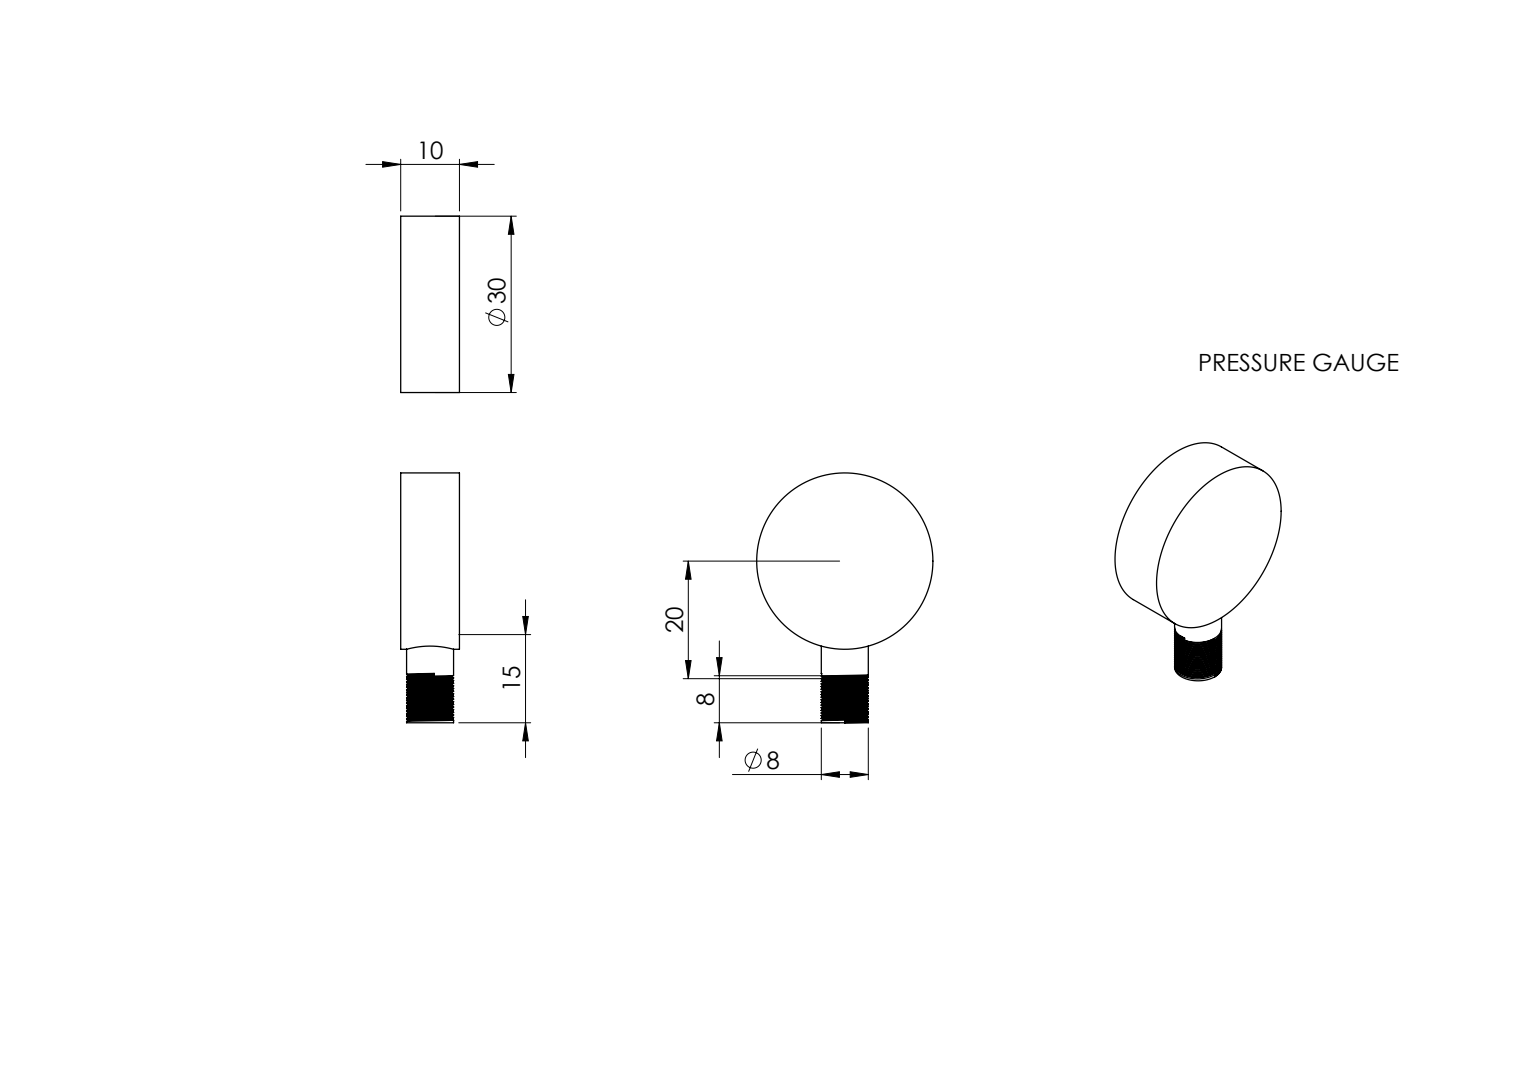
ISO-10303-21;
HEADER;
FILE_DESCRIPTION (('STEP AP214'),
    '1' );
FILE_NAME ('pressure gauge.step',
    '2026-10-26T05:42:23',
    ( '' ),
    ( '' ),
    'SwSTEP 2.0',
    'SolidWorks 2026',
    '' );
FILE_SCHEMA (( 'AUTOMOTIVE_DESIGN' ));
ENDSEC;

DATA;
#24=CARTESIAN_POINT ( 'NONE',  ( -7.967954043666661671E-16, 16.24062499938548143, 34.33755215474603517 ) ) ;
#66=CARTESIAN_POINT ( 'NONE',  ( -3.756430356250000102, 17.92812499938548498, 30.00000000000000000 ) ) ;
#88=CARTESIAN_POINT ( 'NONE',  ( -3.999999999999999112, 19.88749999999999929, 27.69059892324149530 ) ) ;
#102=CARTESIAN_POINT ( 'NONE',  ( -1.071796769724496334, 15.72634618820330310, 26.00000000000000355 ) ) ;
#120=CARTESIAN_POINT ( 'NONE',  ( 3.756430356250000546, 13.57812499938548711, 27.83122392262697886 ) ) ;
#135=CARTESIAN_POINT ( 'NONE',  ( 1.878215178125000495, 19.01562499938548356, 26.74683588394047007 ) ) ;
#150=CARTESIAN_POINT ( 'NONE',  ( 2.828200636599751609E-16, 18.40624999877096712, 25.38119784648299415 ) ) ;
#153=CARTESIAN_POINT ( 'NONE',  ( -3.999999999999999112, 17.58124999877096428, 27.69059892324149530 ) ) ;
#183=CARTESIAN_POINT ( 'NONE',  ( -1.071796769724492115, 14.61740381056766402, 34.00000000000000000 ) ) ;
#197=ORIENTED_EDGE ( 'NONE', *, *, #67048, .T. ) ;
#202=ORIENTED_EDGE ( 'NONE', *, *, #63479, .F. ) ;
#210=ORIENTED_EDGE ( 'NONE', *, *, #33045, .F. ) ;
#259=DIRECTION ( 'NONE',  ( -0.000000000000000000, -1.000000000000000000, -0.000000000000000000 ) ) ;
#264=CARTESIAN_POINT ( 'NONE',  ( -7.967954043666661671E-16, 14.44062499938548250, 34.33755215474603517 ) ) ;
#265=CARTESIAN_POINT ( 'NONE',  ( -1.999999999999999112, 13.94374999877096677, 26.53589838486224650 ) ) ;
#274=EDGE_LOOP ( 'NONE', ( #54307, #37100, #57406 ) ) ;
#276=( BOUNDED_CURVE ( )  B_SPLINE_CURVE ( 2, ( #33865, #44247, #5440, #72677, #27980, #66778, #16868, #50510, #73036 ),
 .UNSPECIFIED., .F., .F. ) 
 B_SPLINE_CURVE_WITH_KNOTS ( ( 3, 2, 2, 2, 3 ),
 ( 0.2916666666666666852, 0.2962962962962962798, 0.3055555555555555802, 0.3148148148148148251, 0.3194444444444444753 ),
 .UNSPECIFIED. ) 
 CURVE ( )  GEOMETRIC_REPRESENTATION_ITEM ( )  RATIONAL_B_SPLINE_CURVE ( ( 0.9330127018922194093, 0.9330127018922197424, 1.000000000000000000, 0.8660254037844387076, 1.000000000000000000, 0.8660254037844387076, 1.000000000000000000, 0.9330127018922189652, 0.9330127018922194093 ) ) 
 REPRESENTATION_ITEM ( '' )  );
#296=CARTESIAN_POINT ( 'NONE',  ( -1.999999999999999112, 17.60000000000000142, 26.53589838486224650 ) ) ;
#341=CARTESIAN_POINT ( 'NONE',  ( -1.626862140677534273E-15, 15.03124999877096535, 34.00000000000000000 ) ) ;
#343=CYLINDRICAL_SURFACE ( 'NONE', #34692, 4.000000000000000000 ) ;
#374=CARTESIAN_POINT ( 'NONE',  ( -1.878215178125001827, 14.85312499938548214, 33.25316411605952283 ) ) ;
#413=ORIENTED_EDGE ( 'NONE', *, *, #34178, .T. ) ;
#416=CARTESIAN_POINT ( 'NONE',  ( 2.655984681222220721E-16, 16.46562499938548285, 25.66244784525396483 ) ) ;
#458=EDGE_CURVE ( 'NONE', #51815, #43576, #43970, .T. ) ;
#473=CARTESIAN_POINT ( 'NONE',  ( 1.878215178125000495, 18.11562499938548498, 26.74683588394047007 ) ) ;
#498=CARTESIAN_POINT ( 'NONE',  ( -4.000000000000000000, 17.16874999877096641, 30.00000000000000000 ) ) ;
#506=CARTESIAN_POINT ( 'NONE',  ( 4.000000000000000000, 17.88124999877096855, 27.69059892324149530 ) ) ;
#534=CARTESIAN_POINT ( 'NONE',  ( 2.000000000000000444, 14.82500000000000107, 26.53589838486224650 ) ) ;
#617=CIRCLE ( 'NONE', #41869, 14.99999999999999822 ) ;
#625=CARTESIAN_POINT ( 'NONE',  ( 4.000000000000000000, 13.85000000000000142, 30.00000000000000000 ) ) ;
#629=CARTESIAN_POINT ( 'NONE',  ( 1.626862140677534470E-15, 13.23124999877096819, 34.00000000000000000 ) ) ;
#631=CARTESIAN_POINT ( 'NONE',  ( 3.756430356250000546, 15.94062499938548427, 27.83122392262697886 ) ) ;
#661=CARTESIAN_POINT ( 'NONE',  ( -2.000000000000001776, 19.54999999999999716, 33.46410161513775705 ) ) ;
#677=AXIS2_PLACEMENT_3D ( 'NONE', #72142, #59579, #42605 ) ;
#697=CARTESIAN_POINT ( 'NONE',  ( 1.071796769724491227, 18.38615380933863008, 26.00000000000000000 ) ) ;
#719=DIRECTION ( 'NONE',  ( -0.000000000000000000, -1.000000000000000000, -0.000000000000000000 ) ) ;
#721=EDGE_CURVE ( 'NONE', #60301, #16877, #21451, .T. ) ;
#724=CARTESIAN_POINT ( 'NONE',  ( 3.756430356250000102, 12.64062499938548356, 30.00000000000000000 ) ) ;
#743=CARTESIAN_POINT ( 'NONE',  ( -7.967954043666661671E-16, 18.49062499938548143, 34.33755215474603517 ) ) ;
#752=CARTESIAN_POINT ( 'NONE',  ( -2.000000000000001776, 16.40000000000000213, 33.46410161513775705 ) ) ;
#783=CARTESIAN_POINT ( 'NONE',  ( 1.878215178124997609, 18.52812499938548285, 33.25316411605952993 ) ) ;
#796=AXIS2_PLACEMENT_3D ( 'NONE', #15994, #54797, #66618 ) ;
#840=CARTESIAN_POINT ( 'NONE',  ( -3.756430356250000102, 16.46562499938548285, 30.00000000000000000 ) ) ;
#842=ORIENTED_EDGE ( 'NONE', *, *, #18114, .T. ) ;
#849=LINE ( 'NONE', #7827, #71099 ) ;
#872=CARTESIAN_POINT ( 'NONE',  ( -1.999999999999999112, 19.34374999877096712, 26.53589838486224650 ) ) ;
#920=ORIENTED_EDGE ( 'NONE', *, *, #27236, .F. ) ;
#926=ORIENTED_EDGE ( 'NONE', *, *, #17867, .T. ) ;
#929=CARTESIAN_POINT ( 'NONE',  ( -2.498395430326213790E-14, 18.85624999877096641, 26.00000000000000000 ) ) ;
#933=CARTESIAN_POINT ( 'NONE',  ( -3.756430356250001434, 14.25312499938548250, 32.16877607737301048 ) ) ;
#995=CARTESIAN_POINT ( 'NONE',  ( 3.756430356250000102, 16.80312499938548498, 30.00000000000000000 ) ) ;
#1026=CARTESIAN_POINT ( 'NONE',  ( 4.000000000000000000, 20.15000000000000213, 30.00000000000000000 ) ) ;
#1043=CARTESIAN_POINT ( 'NONE',  ( -1.626862140677534273E-15, 20.43124999877096570, 34.00000000000000000 ) ) ;
#1108=CARTESIAN_POINT ( 'NONE',  ( -3.756430356250001434, 18.41562499938548214, 32.16877607737301048 ) ) ;
#1110=CARTESIAN_POINT ( 'NONE',  ( 4.000000000000000000, 13.43750000000000000, 27.69059892324149530 ) ) ;
#1183=CARTESIAN_POINT ( 'NONE',  ( -4.000000000000000888, 15.85624999877096641, 32.30940107675850470 ) ) ;
#1201=CARTESIAN_POINT ( 'NONE',  ( -3.756430356250000102, 17.36562499938548498, 30.00000000000000000 ) ) ;
#1223=CARTESIAN_POINT ( 'NONE',  ( -3.999999999999999112, 17.13124999877096499, 27.69059892324149530 ) ) ;
#1230=CARTESIAN_POINT ( 'NONE',  ( 2.655984681222220721E-16, 12.86562499938548321, 25.66244784525396483 ) ) ;
#1241=CARTESIAN_POINT ( 'NONE',  ( -1.243387493232115393E-14, 16.21250000000000213, 26.00000000000000000 ) ) ;
#1260=CARTESIAN_POINT ( 'NONE',  ( -5.000000000000000000, 39.99999999999999289, 45.00000000000000000 ) ) ;
#1282=CARTESIAN_POINT ( 'NONE',  ( 5.810221930991193690E-16, 19.36250000000000071, 26.00000000000000000 ) ) ;
#1289=CARTESIAN_POINT ( 'NONE',  ( 3.756430356249998770, 16.20312499938548356, 32.16877607737302469 ) ) ;
#1316=CARTESIAN_POINT ( 'NONE',  ( -1.243387493232115393E-14, 15.70624999877096784, 26.00000000000000000 ) ) ;
#1352=CARTESIAN_POINT ( 'NONE',  ( 1.878215178125000495, 18.22812499938548214, 26.74683588394047007 ) ) ;
#1385=CARTESIAN_POINT ( 'NONE',  ( -4.000000000000000888, 19.96250000000000213, 32.30940107675850470 ) ) ;
#1412=CARTESIAN_POINT ( 'NONE',  ( -1.626862140677534273E-15, 14.63749999999999929, 34.00000000000000000 ) ) ;
#1422=ORIENTED_EDGE ( 'NONE', *, *, #54762, .F. ) ;
#1424=CARTESIAN_POINT ( 'NONE',  ( 4.000000000000000000, 14.33750000000000213, 27.69059892324149885 ) ) ;
#1435=CARTESIAN_POINT ( 'NONE',  ( 3.999999999999998668, 17.86250000000000071, 32.30940107675850470 ) ) ;
#1452=CARTESIAN_POINT ( 'NONE',  ( 2.009231068734822045, 25.40577629059018605, 33.46852441891628871 ) ) ;
#1469=CARTESIAN_POINT ( 'NONE',  ( -7.967954043666661671E-16, 18.94062499938548783, 34.33755215474603517 ) ) ;
#1471=CARTESIAN_POINT ( 'NONE',  ( 4.000000000000000000, 12.53749999999999964, 27.69059892324149530 ) ) ;
#1506=ORIENTED_EDGE ( 'NONE', *, *, #71856, .F. ) ;
#1509=CARTESIAN_POINT ( 'NONE',  ( -1.878215178125001827, 19.80312499938548143, 33.25316411605952283 ) ) ;
#1561=FACE_OUTER_BOUND ( 'NONE', #67156, .T. ) ;
#1563=CARTESIAN_POINT ( 'NONE',  ( -3.756430356250000990, 17.85312499938548214, 32.16877607737301048 ) ) ;
#1576=CARTESIAN_POINT ( 'NONE',  ( 0.000000000000000000, 27.50000000000000000, 26.00000000000000000 ) ) ;
#1592=CARTESIAN_POINT ( 'NONE',  ( 3.756430356250000546, 12.79062499938548392, 27.83122392262697886 ) ) ;
#1622=EDGE_CURVE ( 'NONE', #69015, #46020, #617, .T. ) ;
#1654=CARTESIAN_POINT ( 'NONE',  ( -3.756430356249999214, 17.32812499938548356, 27.83122392262697531 ) ) ;
#1678=CARTESIAN_POINT ( 'NONE',  ( 3.999999999999998668, 13.30624999877096748, 32.30940107675850470 ) ) ;
#1695=PLANE ( 'NONE',  #41938 ) ;
#1711=CARTESIAN_POINT ( 'NONE',  ( -1.878215178125001827, 16.65312499938548285, 33.25316411605952283 ) ) ;
#1746=CARTESIAN_POINT ( 'NONE',  ( 2.000000000000000444, 19.32500000000000284, 26.53589838486224650 ) ) ;
#1760=CARTESIAN_POINT ( 'NONE',  ( 1.626862140677534470E-15, 13.68124999877096748, 34.00000000000000000 ) ) ;
#1810=DIRECTION ( 'NONE',  ( -0.000000000000000000, -1.000000000000000000, -0.000000000000000000 ) ) ;
#1816=CARTESIAN_POINT ( 'NONE',  ( 0.5273506787484333325, 25.53584304230190938, 33.97379189798129318 ) ) ;
#1830=( BOUNDED_CURVE ( )  B_SPLINE_CURVE ( 2, ( #4171, #10790, #50685, #88, #22593, #38878, #55498, #61397, #4537 ),
 .UNSPECIFIED., .F., .F. ) 
 B_SPLINE_CURVE_WITH_KNOTS ( ( 3, 2, 2, 2, 3 ),
 ( 0.9027777777777777901, 0.9074074074074074403, 0.9166666666666666297, 0.9259259259259259300, 0.9305555555555555802 ),
 .UNSPECIFIED. ) 
 CURVE ( )  GEOMETRIC_REPRESENTATION_ITEM ( )  RATIONAL_B_SPLINE_CURVE ( ( 0.9330127018922194093, 0.9330127018922194093, 1.000000000000000000, 0.8660254037844387076, 1.000000000000000000, 0.8660254037844387076, 1.000000000000000000, 0.9330127018922194093, 0.9330127018922194093 ) ) 
 REPRESENTATION_ITEM ( '' )  );
#1832=CARTESIAN_POINT ( 'NONE',  ( 3.756430356250000102, 17.70312499938548356, 30.00000000000000000 ) ) ;
#1834=CARTESIAN_POINT ( 'NONE',  ( -8.484601909799255319E-16, 13.73749999999999893, 34.61880215351700940 ) ) ;
#1852=EDGE_CURVE ( 'NONE', #15973, #9585, #41547, .T. ) ;
#1873=CARTESIAN_POINT ( 'NONE',  ( -3.756430356250001434, 19.76562499938548356, 32.16877607737301048 ) ) ;
#1877=VECTOR ( 'NONE', #39271, 1000.000000000000000 ) ;
#1883=AXIS2_PLACEMENT_3D ( 'NONE', #31887, #72139, #43707 ) ;
#1915=CARTESIAN_POINT ( 'NONE',  ( -0.2617081364693537582, 25.54316770519903557, 33.99999999999999289 ) ) ;
#1918=CARTESIAN_POINT ( 'NONE',  ( 0.000000000000000000, 27.50000000000000000, 26.00000000000000000 ) ) ;
#1919=ORIENTED_EDGE ( 'NONE', *, *, #12871, .T. ) ;
#1930=CARTESIAN_POINT ( 'NONE',  ( -3.756430356250000990, 18.30312499938548143, 32.16877607737301048 ) ) ;
#1959=CARTESIAN_POINT ( 'NONE',  ( -4.000000000000000888, 19.90624999877096357, 32.30940107675850470 ) ) ;
#1971=EDGE_CURVE ( 'NONE', #40431, #36300, #21687, .T. ) ;
#1983=DIRECTION ( 'NONE',  ( 0.000000000000000000, 0.000000000000000000, -1.000000000000000000 ) ) ;
#2019=CARTESIAN_POINT ( 'NONE',  ( 3.756430356250000102, 17.14062499938548356, 30.00000000000000000 ) ) ;
#2042=CARTESIAN_POINT ( 'NONE',  ( -4.000000000000000000, 14.46874999877096712, 30.00000000000000000 ) ) ;
#2075=CARTESIAN_POINT ( 'NONE',  ( -1.878215178125001827, 17.55312499938548498, 33.25316411605952283 ) ) ;
#2103=VERTEX_POINT ( 'NONE', #30875 ) ;
#2127=CARTESIAN_POINT ( 'NONE',  ( 5.810221930991193690E-16, 13.96249999999999858, 26.00000000000000000 ) ) ;
#2172=CARTESIAN_POINT ( 'NONE',  ( 3.197688915245457508, 25.19820453330248000, 32.45943478522090686 ) ) ;
#2188=CARTESIAN_POINT ( 'NONE',  ( 2.655984681222220721E-16, 17.36562499938548498, 25.66244784525396483 ) ) ;
#2190=CARTESIAN_POINT ( 'NONE',  ( 2.000000000000000444, 12.57500000000000107, 26.53589838486224650 ) ) ;
#2215=( BOUNDED_CURVE ( )  B_SPLINE_CURVE ( 2, ( #15681, #21961, #60746, #10157, #29678, #12683, #12320, #13040, #47036 ),
 .UNSPECIFIED., .F., .F. ) 
 B_SPLINE_CURVE_WITH_KNOTS ( ( 3, 2, 2, 2, 3 ),
 ( 0.1805555555555555525, 0.1851851851851851749, 0.1944444444444444475, 0.2037037037037036924, 0.2083333333333333426 ),
 .UNSPECIFIED. ) 
 CURVE ( )  GEOMETRIC_REPRESENTATION_ITEM ( )  RATIONAL_B_SPLINE_CURVE ( ( 0.9330127018922194093, 0.9330127018922194093, 1.000000000000000000, 0.8660254037844387076, 1.000000000000000000, 0.8660254037844387076, 1.000000000000000000, 0.9330127018922191873, 0.9330127018922194093 ) ) 
 REPRESENTATION_ITEM ( '' )  );
#2229=CARTESIAN_POINT ( 'NONE',  ( -3.756430356249999214, 19.69062499938548427, 27.83122392262697531 ) ) ;
#2251=ORIENTED_EDGE ( 'NONE', *, *, #16220, .T. ) ;
#2280=CARTESIAN_POINT ( 'NONE',  ( 1.878215178125000495, 20.36562499938548143, 26.74683588394047007 ) ) ;
#2311=CARTESIAN_POINT ( 'NONE',  ( 3.756430356250000102, 13.20312499938548356, 30.00000000000000000 ) ) ;
#2319=CARTESIAN_POINT ( 'NONE',  ( -2.498395430326213790E-14, 18.91249999999999787, 26.00000000000000000 ) ) ;
#2322=EDGE_LOOP ( 'NONE', ( #17460, #59592, #43723 ) ) ;
#2332=CARTESIAN_POINT ( 'NONE',  ( -1.999999999999999112, 13.10000000000000142, 26.53589838486224650 ) ) ;
#2362=DIRECTION ( 'NONE',  ( -1.000000000000000000, -0.000000000000000000, -0.000000000000000000 ) ) ;
#2370=CARTESIAN_POINT ( 'NONE',  ( -1.878215178125001827, 18.34062499938548285, 33.25316411605952283 ) ) ;
#2380=CARTESIAN_POINT ( 'NONE',  ( 3.756430356250000546, 16.27812499938548285, 27.83122392262697886 ) ) ;
#2388=CARTESIAN_POINT ( 'NONE',  ( -4.000000000000000888, 15.01250000000000107, 32.30940107675850470 ) ) ;
#2424=CARTESIAN_POINT ( 'NONE',  ( 3.756430356250000102, 17.25312499938548072, 30.00000000000000000 ) ) ;
#2453=EDGE_LOOP ( 'NONE', ( #8138, #56982, #51535, #7010, #49708, #2581 ) ) ;
#2527=CARTESIAN_POINT ( 'NONE',  ( 1.039375613666550624, 25.50811497328423982, 26.12855575835990152 ) ) ;
#2545=CARTESIAN_POINT ( 'NONE',  ( -7.967954043666661671E-16, 12.97812499938548392, 34.33755215474603517 ) ) ;
#2547=CARTESIAN_POINT ( 'NONE',  ( -7.967954043666661671E-16, 19.72812499938548214, 34.33755215474603517 ) ) ;
#2580=CARTESIAN_POINT ( 'NONE',  ( -2.000000000000001776, 17.75000000000000355, 33.46410161513775705 ) ) ;
#2581=ORIENTED_EDGE ( 'NONE', *, *, #44171, .F. ) ;
#2584=CARTESIAN_POINT ( 'NONE',  ( -3.756430356250000102, 19.72812499938548214, 30.00000000000000000 ) ) ;
#2624=CARTESIAN_POINT ( 'NONE',  ( -1.878215178124999163, 13.80312499938548321, 26.74683588394047007 ) ) ;
#2626=ORIENTED_EDGE ( 'NONE', *, *, #70842, .F. ) ;
#2637=AXIS2_PLACEMENT_3D ( 'NONE', #49337, #31609, #32707 ) ;
#2639=CARTESIAN_POINT ( 'NONE',  ( 3.756430356250000546, 18.52812499938548285, 27.83122392262697886 ) ) ;
#2655=CARTESIAN_POINT ( 'NONE',  ( -1.071796769724496334, 15.33259618943233527, 26.00000000000000355 ) ) ;
#2659=EDGE_LOOP ( 'NONE', ( #4142, #55837, #64847, #1422 ) ) ;
#2671=CARTESIAN_POINT ( 'NONE',  ( -1.999999999999999112, 19.79374999877096286, 26.53589838486224650 ) ) ;
#2697=CARTESIAN_POINT ( 'NONE',  ( 2.000000000000000444, 20.22500000000000142, 26.53589838486224650 ) ) ;
#2729=CARTESIAN_POINT ( 'NONE',  ( 3.756430356250000546, 12.67812499938548143, 27.83122392262697886 ) ) ;
#2735=CARTESIAN_POINT ( 'NONE',  ( 3.756430356250000102, 16.69062499938548427, 30.00000000000000000 ) ) ;
#2744=CARTESIAN_POINT ( 'NONE',  ( -3.756430356250000102, 15.11562499938548321, 30.00000000000000000 ) ) ;
#2751=CARTESIAN_POINT ( 'NONE',  ( 1.138803498474273873E-14, 15.08749999999999858, 34.00000000000000000 ) ) ;
#2758=CARTESIAN_POINT ( 'NONE',  ( -4.000000000000000888, 14.50624999877096677, 32.30940107675850470 ) ) ;
#2787=EDGE_CURVE ( 'NONE', #53615, #51815, #29242, .T. ) ;
#2790=CARTESIAN_POINT ( 'NONE',  ( -3.756430356250000990, 19.31562499938548427, 32.16877607737301048 ) ) ;
#2825=CARTESIAN_POINT ( 'NONE',  ( 5.810221930991193690E-16, 19.36250000000000071, 26.00000000000000000 ) ) ;
#2882=CARTESIAN_POINT ( 'NONE',  ( -1.878215178124999163, 13.35312499938548392, 26.74683588394047007 ) ) ;
#2908=CARTESIAN_POINT ( 'NONE',  ( -7.967954043666661671E-16, 13.42812499938548321, 34.33755215474603517 ) ) ;
#2910=CARTESIAN_POINT ( 'NONE',  ( -4.000000000000000000, 15.87500000000000000, 30.00000000000000000 ) ) ;
#2920=( BOUNDED_CURVE ( )  B_SPLINE_CURVE ( 1, ( #61889, #16451 ),
 .UNSPECIFIED., .F., .F. ) 
 B_SPLINE_CURVE_WITH_KNOTS ( ( 2, 2 ),
 ( 0.000000000000000000, 1.000000000000000000 ),
 .UNSPECIFIED. ) 
 CURVE ( )  GEOMETRIC_REPRESENTATION_ITEM ( )  RATIONAL_B_SPLINE_CURVE ( ( 0.9401540605060327849, 0.9401540605060327849 ) ) 
 REPRESENTATION_ITEM ( '' )  );
#2944=( BOUNDED_CURVE ( )  B_SPLINE_CURVE ( 2, ( #4358, #66399, #32416, #15411, #15051, #15776, #49781, #65291, #44243 ),
 .UNSPECIFIED., .F., .F. ) 
 B_SPLINE_CURVE_WITH_KNOTS ( ( 3, 2, 2, 2, 3 ),
 ( 0.6805555555555555802, 0.6851851851851852304, 0.6944444444444444198, 0.7037037037037037202, 0.7083333333333333703 ),
 .UNSPECIFIED. ) 
 CURVE ( )  GEOMETRIC_REPRESENTATION_ITEM ( )  RATIONAL_B_SPLINE_CURVE ( ( 0.9330127018922194093, 0.9330127018922194093, 1.000000000000000000, 0.8660254037844387076, 1.000000000000000000, 0.8660254037844387076, 1.000000000000000000, 0.9330127018922185211, 0.9330127018922192983 ) ) 
 REPRESENTATION_ITEM ( '' )  );
#2989=CARTESIAN_POINT ( 'NONE',  ( -3.594031514960484675, 25.10343495127339608, 28.22486214709212149 ) ) ;
#2992=CARTESIAN_POINT ( 'NONE',  ( -3.756430356250000102, 13.87812499938548250, 30.00000000000000000 ) ) ;
#3004=CARTESIAN_POINT ( 'NONE',  ( -7.967954043666661671E-16, 18.82812499938548356, 34.33755215474603517 ) ) ;
#3023=ORIENTED_EDGE ( 'NONE', *, *, #4912, .T. ) ;
#3036=CARTESIAN_POINT ( 'NONE',  ( 2.655984681222220721E-16, 14.21562499938548463, 25.66244784525396483 ) ) ;
#3081=CARTESIAN_POINT ( 'NONE',  ( 0.000000000000000000, 12.50000000000000000, 30.00000000000000000 ) ) ;
#3101=CARTESIAN_POINT ( 'NONE',  ( -3.756430356250001434, 20.55312499938548498, 32.16877607737301048 ) ) ;
#3110=CARTESIAN_POINT ( 'NONE',  ( 3.756430356249998770, 16.20312499938548356, 32.16877607737302469 ) ) ;
#3128=CARTESIAN_POINT ( 'NONE',  ( 4.000000000000000000, 14.28124999877096535, 27.69059892324149530 ) ) ;
#3163=CARTESIAN_POINT ( 'NONE',  ( 3.756430356249998770, 19.01562499938548356, 32.16877607737301759 ) ) ;
#3165=VECTOR ( 'NONE', #44966, 1000.000000000000000 ) ;
#3283=CARTESIAN_POINT ( 'NONE',  ( -1.878215178125001827, 20.70312499938548001, 33.25316411605952283 ) ) ;
#3285=CARTESIAN_POINT ( 'NONE',  ( -4.000000000000000888, 15.46250000000000036, 32.30940107675850470 ) ) ;
#3331=AXIS2_PLACEMENT_3D ( 'NONE', #51135, #6790, #28243 ) ;
#3360=CARTESIAN_POINT ( 'NONE',  ( 1.999999999999997335, 16.47500000000000142, 33.46410161513775705 ) ) ;
#3369=CARTESIAN_POINT ( 'NONE',  ( -0.5270301578798420872, 25.53585070951882230, 26.02618134498960245 ) ) ;
#3373=CARTESIAN_POINT ( 'NONE',  ( 4.000000000000000000, 15.65000000000000036, 30.00000000000000000 ) ) ;
#3384=CARTESIAN_POINT ( 'NONE',  ( -3.756430356250000990, 19.65312499938548640, 32.16877607737301048 ) ) ;
#3396=CARTESIAN_POINT ( 'NONE',  ( 4.000000000000000000, 14.73124999877096641, 27.69059892324149885 ) ) ;
#3416=CARTESIAN_POINT ( 'NONE',  ( 3.756430356249998770, 15.86562499938548321, 32.16877607737302469 ) ) ;
#3433=PRODUCT_DEFINITION ( 'UNKNOWN', '', #16707, #69118 ) ;
#3460=CARTESIAN_POINT ( 'NONE',  ( -4.000000000000000000, 19.86874999877096570, 30.00000000000000000 ) ) ;
#3477=( BOUNDED_SURFACE ( )  B_SPLINE_SURFACE ( 1, 2, ( 
 ( #26135, #30218, #52752, #24666, #48676, #30584, #53110, #44237, #32777, #49047, #66393, #39052, #37947, #43502, #55314, #27239, #4708, #49776, #27605, #26506, #72669, #26879, #43869, #60466, #71940, #15770, #71575, #16497, #44609, #67139, #32409, #72300, #49408, #61212, #38312, #54947, #33136, #22048, #15044, #9513, #5070, #21680, #21316, #20949, #66768, #66027, #16141, #60839, #32046, #10607, #54578, #4352, #9875, #15405, #3982, #10244, #38693, #37582, #60104, #55673, #50138, #25639, #64791, #30813, #53346, #47810, #2744, #69975, #9384, #14182, #37816, #7918, #41900, #70339, #65897, #19345, #14546, #64427, #42268, #53718, #48545, #54452, #19716, #26006, #65156, #31916, #13819, #36359, #25263, #3851, #36716, #59238, #8646, #48177, #31175, #3110, #70701, #2380, #48912, #65528, #37082, #26372, #71443, #58873, #8283, #20818, #54090, #20076, #42632, #71072, #59606, #20447, #9020, #24898, #14914, #52984, #31550, #3488, #42997, #47443, #37456, #59975, #30455, #15277, #43373, #21550, #4942, #44105, #10115, #32645, #27111, #55186, #49280, #61803, #66631, #17096, #60336, #21183, #49644, #45191, #71813, #67008, #43735, #16008, #33007, #27846, #33733, #72171, #5300, #44477, #11206, #66259, #15637, #4581, #56279, #38557, #61080, #10478, #27476, #55546, #50008, #72533, #54813, #28204, #44836, #16369, #5668, #50733, #38178, #60702, #135, #21921, #38924, #67723, #39289, #61443, #4219, #10836, #9745, #33372, #22641, #55908, #50377, #72902, #26747, #22284, #67371, #16734, #32279, #2547, #12538, #18785, #52789, #35788, #58311, #13615, #19148, #63143, #57952, #68340, #35428, #7722, #30256, #7001, #18063, #23977, #7360, #63860, #41350, #46163, #35072, #24704, #69428, #52067, #40624, #30618, #12174 ),
 ( #13250, #1471, #2190, #12895, #29532, #47248, #36160, #58678, #17700, #69781, #29889, #41702, #64226, #8088, #46525, #53148, #45804, #51707, #40261, #69067, #18426, #62782, #34702, #57231, #6646, #1110, #29173, #23617, #52428, #40992, #68703, #57598, #63508, #1834, #24342, #46890, #37257, #59043, #47609, #54615, #53894, #19888, #42441, #42075, #49087, #14354, #13984, #20618, #60506, #9912, #32450, #3652, #65324, #54256, #65695, #9185, #30983, #42802, #54985, #64963, #25441, #26175, #48716, #71238, #31720, #20988, #8447, #15440, #31353, #20250, #36889, #25813, #14715, #53516, #25066, #70139, #19517, #59408, #43176, #3285, #32084, #59779, #8816, #4021, #37984, #64597, #36523, #26546, #15082, #48351, #2910, #37619, #47984, #60141, #70876, #70512, #71615, #9550, #43541, #66062, #55352, #43909, #10645, #39091, #34252, #11735, #49813, #38731, #22089, #61251, #27280, #72338, #44277, #21718, #66432, #5829, #33175, #4391, #26920, #38352, #66808, #62339, #15810, #11009, #60879, #55713, #50178, #44997, #50896, #16180, #22448, #61608, #28360, #10284, #32814, #5108, #296, #27642, #73067, #39825, #49445, #71979, #56080, #44647, #33530, #67534, #5471, #4746, #67177, #21352, #72706, #16538, #28011, #50539, #16897, #39452, #22805, #61973, #67891, #11375, #33894, #56438, #45357, #17263, #17620, #64141, #19064, #41622, #68617, #29808, #12457, #63778, #23895, #17980, #35707, #47167, #69699, #28719, #58229, #52343, #6918, #12095, #1746, #40180, #46807, #29448, #51259, #13166, #661, #40539, #23532, #34616, #23169, #63055, #18338, #13528, #56784, #29090, #34988, #1385, #57517, #6558, #51626, #46082, #1026, #45723, #7634, #51986, #6190, #68258, #62700, #46443, #57146, #68981, #63424, #40911, #12811 ) ),
 .UNSPECIFIED., .F., .F., .F. ) 
 B_SPLINE_SURFACE_WITH_KNOTS ( ( 2, 2 ),
 ( 3, 2, 2, 2, 2, 2, 2, 2, 2, 2, 2, 2, 2, 2, 2, 2, 2, 2, 2, 2, 2, 2, 2, 2, 2, 2, 2, 2, 2, 2, 2, 2, 2, 2, 2, 2, 2, 2, 2, 2, 2, 2, 2, 2, 2, 2, 2, 2, 2, 2, 2, 2, 2, 2, 2, 2, 2, 2, 2, 2, 2, 2, 2, 2, 2, 2, 2, 2, 2, 2, 2, 2, 2, 2, 2, 2, 2, 2, 2, 2, 2, 2, 2, 2, 2, 2, 2, 2, 2, 2, 2, 2, 2, 2, 2, 2, 2, 2, 2, 2, 2, 2, 2, 2, 2, 2, 2, 2, 3 ),
 ( 0.000000000000000000, 1.000000000000000000 ),
 ( 0.000000000000000000, 0.009259259259259258745, 0.01851851851851851749, 0.02777777777777777624, 0.03703703703703703498, 0.04629629629629629373, 0.05555555555555555247, 0.06481481481481481122, 0.07407407407407406996, 0.08333333333333332871, 0.09259259259259258745, 0.1018518518518518462, 0.1111111111111111049, 0.1203703703703703637, 0.1296296296296296224, 0.1388888888888888951, 0.1481481481481481399, 0.1574074074074074125, 0.1666666666666666574, 0.1759259259259259300, 0.1851851851851851749, 0.1944444444444444475, 0.2037037037037036924, 0.2129629629629629650, 0.2222222222222222099, 0.2314814814814814825, 0.2407407407407407274, 0.2500000000000000000, 0.2592592592592592449, 0.2685185185185185452, 0.2777777777777777901, 0.2870370370370370350, 0.2962962962962962798, 0.3055555555555555802, 0.3148148148148148251, 0.3240740740740740700, 0.3333333333333333148, 0.3425925925925926152, 0.3518518518518518601, 0.3611111111111111049, 0.3703703703703703498, 0.3796296296296296502, 0.3888888888888888951, 0.3981481481481481399, 0.4074074074074073848, 0.4166666666666666852, 0.4259259259259259300, 0.4351851851851851749, 0.4444444444444444198, 0.4537037037037037202, 0.4629629629629629650, 0.4722222222222222099, 0.4814814814814814548, 0.4907407407407407551, 0.5000000000000000000, 0.5092592592592593004, 0.5185185185185184897, 0.5277777777777777901, 0.5370370370370370905, 0.5462962962962962798, 0.5555555555555555802, 0.5648148148148147696, 0.5740740740740740700, 0.5833333333333333703, 0.5925925925925925597, 0.6018518518518518601, 0.6111111111111111605, 0.6203703703703703498, 0.6296296296296296502, 0.6388888888888888395, 0.6481481481481481399, 0.6574074074074074403, 0.6666666666666666297, 0.6759259259259259300, 0.6851851851851852304, 0.6944444444444444198, 0.7037037037037037202, 0.7129629629629629095, 0.7222222222222222099, 0.7314814814814815103, 0.7407407407407406996, 0.7500000000000000000, 0.7592592592592593004, 0.7685185185185184897, 0.7777777777777777901, 0.7870370370370370905, 0.7962962962962962798, 0.8055555555555555802, 0.8148148148148147696, 0.8240740740740740700, 0.8333333333333333703, 0.8425925925925925597, 0.8518518518518518601, 0.8611111111111111605, 0.8703703703703703498, 0.8796296296296296502, 0.8888888888888888395, 0.8981481481481481399, 0.9074074074074074403, 0.9166666666666666297, 0.9259259259259259300, 0.9351851851851852304, 0.9444444444444444198, 0.9537037037037037202, 0.9629629629629629095, 0.9722222222222222099, 0.9814814814814815103, 0.9876227234888749207, 0.9974989507237637110 ),
 .UNSPECIFIED. ) 
 GEOMETRIC_REPRESENTATION_ITEM ( )  RATIONAL_B_SPLINE_SURFACE ( (
 ( 1.000000000000000000, 0.8660254037844387076, 1.000000000000000000, 0.8660254037844387076, 1.000000000000000000, 0.8660254037844387076, 1.000000000000000000, 0.8660254037844387076, 1.000000000000000000, 0.8660254037844387076, 1.000000000000000000, 0.8660254037844387076, 1.000000000000000000, 0.8660254037844387076, 1.000000000000000000, 0.8660254037844387076, 1.000000000000000000, 0.8660254037844387076, 1.000000000000000000, 0.8660254037844387076, 1.000000000000000000, 0.8660254037844387076, 1.000000000000000000, 0.8660254037844387076, 1.000000000000000000, 0.8660254037844387076, 1.000000000000000000, 0.8660254037844387076, 1.000000000000000000, 0.8660254037844387076, 1.000000000000000000, 0.8660254037844387076, 1.000000000000000000, 0.8660254037844387076, 1.000000000000000000, 0.8660254037844387076, 1.000000000000000000, 0.8660254037844387076, 1.000000000000000000, 0.8660254037844387076, 1.000000000000000000, 0.8660254037844387076, 1.000000000000000000, 0.8660254037844387076, 1.000000000000000000, 0.8660254037844387076, 1.000000000000000000, 0.8660254037844387076, 1.000000000000000000, 0.8660254037844387076, 1.000000000000000000, 0.8660254037844387076, 1.000000000000000000, 0.8660254037844387076, 1.000000000000000000, 0.8660254037844387076, 1.000000000000000000, 0.8660254037844387076, 1.000000000000000000, 0.8660254037844387076, 1.000000000000000000, 0.8660254037844387076, 1.000000000000000000, 0.8660254037844387076, 1.000000000000000000, 0.8660254037844387076, 1.000000000000000000, 0.8660254037844387076, 1.000000000000000000, 0.8660254037844387076, 1.000000000000000000, 0.8660254037844387076, 1.000000000000000000, 0.8660254037844387076, 1.000000000000000000, 0.8660254037844387076, 1.000000000000000000, 0.8660254037844387076, 1.000000000000000000, 0.8660254037844387076, 1.000000000000000000, 0.8660254037844387076, 1.000000000000000000, 0.8660254037844387076, 1.000000000000000000, 0.8660254037844387076, 1.000000000000000000, 0.8660254037844387076, 1.000000000000000000, 0.8660254037844387076, 1.000000000000000000, 0.8660254037844387076, 1.000000000000000000, 0.8660254037844387076, 1.000000000000000000, 0.8660254037844387076, 1.000000000000000000, 0.8660254037844387076, 1.000000000000000000, 0.8660254037844387076, 1.000000000000000000, 0.8660254037844387076, 1.000000000000000000, 0.8660254037844387076, 1.000000000000000000, 0.8660254037844387076, 1.000000000000000000, 0.8660254037844387076, 1.000000000000000000, 0.8660254037844387076, 1.000000000000000000, 0.8660254037844387076, 1.000000000000000000, 0.8660254037844387076, 1.000000000000000000, 0.8660254037844387076, 1.000000000000000000, 0.8660254037844387076, 1.000000000000000000, 0.8660254037844387076, 1.000000000000000000, 0.8660254037844387076, 1.000000000000000000, 0.8660254037844387076, 1.000000000000000000, 0.8660254037844387076, 1.000000000000000000, 0.8660254037844387076, 1.000000000000000000, 0.8660254037844387076, 1.000000000000000000, 0.8660254037844387076, 1.000000000000000000, 0.8660254037844387076, 1.000000000000000000, 0.8660254037844387076, 1.000000000000000000, 0.8660254037844387076, 1.000000000000000000, 0.8660254037844387076, 1.000000000000000000, 0.8660254037844387076, 1.000000000000000000, 0.8660254037844387076, 1.000000000000000000, 0.8660254037844387076, 1.000000000000000000, 0.8660254037844387076, 1.000000000000000000, 0.8660254037844387076, 1.000000000000000000, 0.8660254037844387076, 1.000000000000000000, 0.8660254037844387076, 1.000000000000000000, 0.8660254037844387076, 1.000000000000000000, 0.8660254037844387076, 1.000000000000000000, 0.8660254037844387076, 1.000000000000000000, 0.8660254037844387076, 1.000000000000000000, 0.8660254037844387076, 1.000000000000000000, 0.8660254037844387076, 1.000000000000000000, 0.8660254037844387076, 1.000000000000000000, 0.8660254037844387076, 1.000000000000000000, 0.8660254037844387076, 1.000000000000000000, 0.8660254037844387076, 1.000000000000000000, 0.8660254037844387076, 1.000000000000000000, 0.8660254037844387076, 1.000000000000000000, 0.8660254037844387076, 1.000000000000000000, 0.8660254037844387076, 1.000000000000000000, 0.8660254037844387076, 1.000000000000000000, 0.8660254037844387076, 1.000000000000000000, 0.8660254037844387076, 1.000000000000000000, 0.8660254037844387076, 1.000000000000000000, 0.8660254037844387076, 1.000000000000000000, 0.8660254037844387076, 1.000000000000000000, 0.8660254037844387076, 1.000000000000000000, 0.8660254037844387076, 1.000000000000000000, 0.8660254037844387076, 1.000000000000000000, 0.8660254037844387076, 1.000000000000000000, 0.8660254037844387076, 1.000000000000000000, 0.8660254037844387076, 1.000000000000000000, 0.8660254037844387076, 1.000000000000000000, 0.8660254037844387076, 1.000000000000000000, 0.8660254037844387076, 1.000000000000000000, 0.9111407948341212482, 0.9401540605060327849, 0.9401540605060327849, 0.9401540605060327849),
 ( 1.000000000000000000, 0.8660254037844387076, 1.000000000000000000, 0.8660254037844387076, 1.000000000000000000, 0.8660254037844387076, 1.000000000000000000, 0.8660254037844387076, 1.000000000000000000, 0.8660254037844387076, 1.000000000000000000, 0.8660254037844387076, 1.000000000000000000, 0.8660254037844387076, 1.000000000000000000, 0.8660254037844387076, 1.000000000000000000, 0.8660254037844387076, 1.000000000000000000, 0.8660254037844387076, 1.000000000000000000, 0.8660254037844387076, 1.000000000000000000, 0.8660254037844387076, 1.000000000000000000, 0.8660254037844387076, 1.000000000000000000, 0.8660254037844387076, 1.000000000000000000, 0.8660254037844387076, 1.000000000000000000, 0.8660254037844387076, 1.000000000000000000, 0.8660254037844387076, 1.000000000000000000, 0.8660254037844387076, 1.000000000000000000, 0.8660254037844387076, 1.000000000000000000, 0.8660254037844387076, 1.000000000000000000, 0.8660254037844387076, 1.000000000000000000, 0.8660254037844387076, 1.000000000000000000, 0.8660254037844387076, 1.000000000000000000, 0.8660254037844387076, 1.000000000000000000, 0.8660254037844387076, 1.000000000000000000, 0.8660254037844387076, 1.000000000000000000, 0.8660254037844387076, 1.000000000000000000, 0.8660254037844387076, 1.000000000000000000, 0.8660254037844387076, 1.000000000000000000, 0.8660254037844387076, 1.000000000000000000, 0.8660254037844387076, 1.000000000000000000, 0.8660254037844387076, 1.000000000000000000, 0.8660254037844387076, 1.000000000000000000, 0.8660254037844387076, 1.000000000000000000, 0.8660254037844387076, 1.000000000000000000, 0.8660254037844387076, 1.000000000000000000, 0.8660254037844387076, 1.000000000000000000, 0.8660254037844387076, 1.000000000000000000, 0.8660254037844387076, 1.000000000000000000, 0.8660254037844387076, 1.000000000000000000, 0.8660254037844387076, 1.000000000000000000, 0.8660254037844387076, 1.000000000000000000, 0.8660254037844387076, 1.000000000000000000, 0.8660254037844387076, 1.000000000000000000, 0.8660254037844387076, 1.000000000000000000, 0.8660254037844387076, 1.000000000000000000, 0.8660254037844387076, 1.000000000000000000, 0.8660254037844387076, 1.000000000000000000, 0.8660254037844387076, 1.000000000000000000, 0.8660254037844387076, 1.000000000000000000, 0.8660254037844387076, 1.000000000000000000, 0.8660254037844387076, 1.000000000000000000, 0.8660254037844387076, 1.000000000000000000, 0.8660254037844387076, 1.000000000000000000, 0.8660254037844387076, 1.000000000000000000, 0.8660254037844387076, 1.000000000000000000, 0.8660254037844387076, 1.000000000000000000, 0.8660254037844387076, 1.000000000000000000, 0.8660254037844387076, 1.000000000000000000, 0.8660254037844387076, 1.000000000000000000, 0.8660254037844387076, 1.000000000000000000, 0.8660254037844387076, 1.000000000000000000, 0.8660254037844387076, 1.000000000000000000, 0.8660254037844387076, 1.000000000000000000, 0.8660254037844387076, 1.000000000000000000, 0.8660254037844387076, 1.000000000000000000, 0.8660254037844387076, 1.000000000000000000, 0.8660254037844387076, 1.000000000000000000, 0.8660254037844387076, 1.000000000000000000, 0.8660254037844387076, 1.000000000000000000, 0.8660254037844387076, 1.000000000000000000, 0.8660254037844387076, 1.000000000000000000, 0.8660254037844387076, 1.000000000000000000, 0.8660254037844387076, 1.000000000000000000, 0.8660254037844387076, 1.000000000000000000, 0.8660254037844387076, 1.000000000000000000, 0.8660254037844387076, 1.000000000000000000, 0.8660254037844387076, 1.000000000000000000, 0.8660254037844387076, 1.000000000000000000, 0.8660254037844387076, 1.000000000000000000, 0.8660254037844387076, 1.000000000000000000, 0.8660254037844387076, 1.000000000000000000, 0.8660254037844387076, 1.000000000000000000, 0.8660254037844387076, 1.000000000000000000, 0.8660254037844387076, 1.000000000000000000, 0.8660254037844387076, 1.000000000000000000, 0.8660254037844387076, 1.000000000000000000, 0.8660254037844387076, 1.000000000000000000, 0.8660254037844387076, 1.000000000000000000, 0.8660254037844387076, 1.000000000000000000, 0.8660254037844387076, 1.000000000000000000, 0.8660254037844387076, 1.000000000000000000, 0.8660254037844387076, 1.000000000000000000, 0.8660254037844387076, 1.000000000000000000, 0.8660254037844387076, 1.000000000000000000, 0.8660254037844387076, 1.000000000000000000, 0.8660254037844387076, 1.000000000000000000, 0.8660254037844387076, 1.000000000000000000, 0.8660254037844387076, 1.000000000000000000, 0.8660254037844387076, 1.000000000000000000, 0.8660254037844387076, 1.000000000000000000, 0.8660254037844387076, 1.000000000000000000, 0.8660254037844387076, 1.000000000000000000, 0.8660254037844387076, 1.000000000000000000, 0.8660254037844387076, 1.000000000000000000, 0.8660254037844387076, 1.000000000000000000, 0.9111407948341212482, 0.9401540605060327849, 0.9401540605060327849, 0.9401540605060327849) ) ) 
 REPRESENTATION_ITEM ( '' )  SURFACE ( )  );
#3478=CARTESIAN_POINT ( 'NONE',  ( 1.878215178125000495, 19.01562499938548356, 26.74683588394047007 ) ) ;
#3488=CARTESIAN_POINT ( 'NONE',  ( -7.967954043666661671E-16, 17.02812499938548285, 34.33755215474603517 ) ) ;
#3502=CARTESIAN_POINT ( 'NONE',  ( -2.000000000000001776, 14.99374999877096570, 33.46410161513775705 ) ) ;
#3532=CARTESIAN_POINT ( 'NONE',  ( -3.756430356249999214, 19.69062499938548427, 27.83122392262697176 ) ) ;
#3541=DIRECTION ( 'NONE',  ( -0.000000000000000000, -1.000000000000000000, -0.000000000000000000 ) ) ;
#3547=EDGE_CURVE ( 'NONE', #46020, #17018, #41522, .T. ) ;
#3561=VERTEX_POINT ( 'NONE', #25620 ) ;
#3567=CARTESIAN_POINT ( 'NONE',  ( -4.000000000000000888, 19.51250000000000284, 32.30940107675850470 ) ) ;
#3608=EDGE_CURVE ( 'NONE', #41920, #28631, #11780, .T. ) ;
#3650=CARTESIAN_POINT ( 'NONE',  ( -1.878215178124999163, 20.55312499938548143, 26.74683588394047007 ) ) ;
#3652=CARTESIAN_POINT ( 'NONE',  ( 2.828200636599751609E-16, 14.41249999999999964, 25.38119784648299415 ) ) ;
#3665=ORIENTED_EDGE ( 'NONE', *, *, #40237, .F. ) ;
#3731=PLANE ( 'NONE',  #70149 ) ;
#3735=CARTESIAN_POINT ( 'NONE',  ( 3.756430356250000102, 13.20312499938548356, 30.00000000000000000 ) ) ;
#3746=CARTESIAN_POINT ( 'NONE',  ( -7.967954043666661671E-16, 19.72812499938547859, 34.33755215474603517 ) ) ;
#3777=CARTESIAN_POINT ( 'NONE',  ( 2.655984681222220721E-16, 14.66562499938548214, 25.66244784525396483 ) ) ;
#3835=CARTESIAN_POINT ( 'NONE',  ( 1.878215178125000495, 12.71562499938548463, 26.74683588394047007 ) ) ;
#3851=CARTESIAN_POINT ( 'NONE',  ( -3.756430356249999214, 15.97812499938548392, 27.83122392262697531 ) ) ;
#3865=CARTESIAN_POINT ( 'NONE',  ( -4.000000000000000000, 16.71874999877096712, 30.00000000000000000 ) ) ;
#3897=CARTESIAN_POINT ( 'NONE',  ( 1.626862140677534470E-15, 12.83750000000000213, 34.00000000000000000 ) ) ;
#3900=CARTESIAN_POINT ( 'NONE',  ( 3.756430356250000546, 19.54062499938548214, 27.83122392262697886 ) ) ;
#3901=DIRECTION ( 'NONE',  ( 0.000000000000000000, 0.000000000000000000, -1.000000000000000000 ) ) ;
#3914=ORIENTED_EDGE ( 'NONE', *, *, #55506, .T. ) ;
#3925=CARTESIAN_POINT ( 'NONE',  ( 1.071796769724491893, 14.15134618820330203, 34.00000000000000000 ) ) ;
#3932=DIRECTION ( 'NONE',  ( -0.000000000000000000, -1.000000000000000000, -0.000000000000000000 ) ) ;
#3935=CARTESIAN_POINT ( 'NONE',  ( -3.999999999999999112, 19.43750000000000000, 27.69059892324149530 ) ) ;
#3936=CARTESIAN_POINT ( 'NONE',  ( -1.999999999999999112, 17.99374999877096570, 26.53589838486224650 ) ) ;
#3973=DIRECTION ( 'NONE',  ( -0.000000000000000000, -1.000000000000000000, -0.000000000000000000 ) ) ;
#3982=CARTESIAN_POINT ( 'NONE',  ( -3.756430356250000102, 14.66562499938548214, 30.00000000000000000 ) ) ;
#3991=CARTESIAN_POINT ( 'NONE',  ( 0.000000000000000000, 27.50000000000000000, 30.00000000000000000 ) ) ;
#4019=CARTESIAN_POINT ( 'NONE',  ( -3.756430356250000102, 20.62812499938548072, 30.00000000000000000 ) ) ;
#4021=CARTESIAN_POINT ( 'NONE',  ( 3.999999999999998668, 15.61250000000000249, 32.30940107675850470 ) ) ;
#4027=DIRECTION ( 'NONE',  ( -0.000000000000000000, -1.000000000000000000, -0.000000000000000000 ) ) ;
#4034=VERTEX_POINT ( 'NONE', #22979 ) ;
#4046=CARTESIAN_POINT ( 'NONE',  ( -2.498395430326213790E-14, 18.85624999877096641, 26.00000000000000000 ) ) ;
#4064=EDGE_CURVE ( 'NONE', #19771, #2103, #50714, .T. ) ;
#4069=CARTESIAN_POINT ( 'NONE',  ( -2.000000000000001776, 13.19374999877096677, 33.46410161513775705 ) ) ;
#4071=CARTESIAN_POINT ( 'NONE',  ( 0.000000000000000000, 27.50000000000000000, 26.00000000000000000 ) ) ;
#4073=CARTESIAN_POINT ( 'NONE',  ( -3.486133158594716510E-16, 13.00624999877096855, 26.00000000000000355 ) ) ;
#4102=ADVANCED_FACE ( 'NONE', ( #1561 ), #62510, .T. ) ;
#4106=CARTESIAN_POINT ( 'NONE',  ( -1.878215178124999163, 12.90312499938548463, 26.74683588394047007 ) ) ;
#4116=DIRECTION ( 'NONE',  ( -0.000000000000000000, -1.000000000000000000, -0.000000000000000000 ) ) ;
#4142=ORIENTED_EDGE ( 'NONE', *, *, #19175, .F. ) ;
#4146=CARTESIAN_POINT ( 'NONE',  ( 3.756430356249998770, 14.96562499938548108, 32.16877607737302469 ) ) ;
#4171=CARTESIAN_POINT ( 'NONE',  ( 5.810221930991193690E-16, 19.81250000000000000, 26.00000000000000000 ) ) ;
#4202=CARTESIAN_POINT ( 'NONE',  ( -1.878215178125001827, 14.29062499938548392, 33.25316411605952283 ) ) ;
#4205=ORIENTED_EDGE ( 'NONE', *, *, #49986, .F. ) ;
#4209=CARTESIAN_POINT ( 'NONE',  ( -3.756430356250001434, 19.20312499938548356, 32.16877607737301048 ) ) ;
#4219=CARTESIAN_POINT ( 'NONE',  ( -1.878215178125001827, 19.24062499938548143, 33.25316411605952283 ) ) ;
#4226=( BOUNDED_CURVE ( )  B_SPLINE_CURVE ( 2, ( #60031, #71128, #20501, #43058, #44537, #65583, #14973, #9443, #31971 ),
 .UNSPECIFIED., .F., .F. ) 
 B_SPLINE_CURVE_WITH_KNOTS ( ( 3, 2, 2, 2, 3 ),
 ( 0.9583333333333333703, 0.9629629629629629095, 0.9722222222222222099, 0.9814814814814815103, 0.9861111111111111605 ),
 .UNSPECIFIED. ) 
 CURVE ( )  GEOMETRIC_REPRESENTATION_ITEM ( )  RATIONAL_B_SPLINE_CURVE ( ( 0.9330127018922192983, 0.9330127018922200755, 1.000000000000000000, 0.8660254037844387076, 1.000000000000000000, 0.8660254037844387076, 1.000000000000000000, 0.9330127018922186322, 0.9330127018922194093 ) ) 
 REPRESENTATION_ITEM ( '' )  );
#4236=CARTESIAN_POINT ( 'NONE',  ( -1.999999999999999112, 16.19374999877096499, 26.53589838486224650 ) ) ;
#4270=CARTESIAN_POINT ( 'NONE',  ( -7.967954043666661671E-16, 18.94062499938548427, 34.33755215474603517 ) ) ;
#4271=CARTESIAN_POINT ( 'NONE',  ( -1.999999999999999112, 14.45000000000000107, 26.53589838486224650 ) ) ;
#4284=EDGE_CURVE ( 'NONE', #4034, #40431, #7092, .T. ) ;
#4287=CARTESIAN_POINT ( 'NONE',  ( 3.999999999999998668, 19.21250000000000213, 32.30940107675850470 ) ) ;
#4299=ORIENTED_EDGE ( 'NONE', *, *, #54732, .F. ) ;
#4344=CARTESIAN_POINT ( 'NONE',  ( 1.071796769724479237, 17.03615380933862866, 25.99999999999999645 ) ) ;
#4352=CARTESIAN_POINT ( 'NONE',  ( 2.655984681222220721E-16, 14.55312499938548321, 25.66244784525396483 ) ) ;
#4358=CARTESIAN_POINT ( 'NONE',  ( 5.810221930991193690E-16, 18.40624999877096357, 26.00000000000000000 ) ) ;
#4361=CARTESIAN_POINT ( 'NONE',  ( 3.756430356250000546, 12.79062499938548214, 27.83122392262697886 ) ) ;
#4370=CARTESIAN_POINT ( 'NONE',  ( -2.672702088255949472E-15, 13.51250000000000107, 26.00000000000000000 ) ) ;
#4389=CARTESIAN_POINT ( 'NONE',  ( 1.878215178125000495, 14.06562499938548250, 26.74683588394047007 ) ) ;
#4391=CARTESIAN_POINT ( 'NONE',  ( -8.484601909799255319E-16, 16.88749999999999929, 34.61880215351700940 ) ) ;
#4435=ORIENTED_EDGE ( 'NONE', *, *, #34178, .F. ) ;
#4471=CARTESIAN_POINT ( 'NONE',  ( -3.756430356249999214, 16.99062499938548143, 27.83122392262697531 ) ) ;
#4480=CARTESIAN_POINT ( 'NONE',  ( 4.000000000000000000, 16.49374999877096570, 30.00000000000000000 ) ) ;
#4501=ORIENTED_EDGE ( 'NONE', *, *, #23875, .F. ) ;
#4514=CARTESIAN_POINT ( 'NONE',  ( 1.878215178125000495, 15.97812499938548392, 26.74683588394047007 ) ) ;
#4537=CARTESIAN_POINT ( 'NONE',  ( -1.626862140677534273E-15, 20.03749999999999787, 34.00000000000000000 ) ) ;
#4555=CARTESIAN_POINT ( 'NONE',  ( -2.000000000000001776, 19.94374999877096499, 33.46410161513775705 ) ) ;
#4566=CARTESIAN_POINT ( 'NONE',  ( -1.878215178124999163, 15.49062499938548321, 26.74683588394047007 ) ) ;
#4572=CARTESIAN_POINT ( 'NONE',  ( 1.878215178124997609, 19.31562499938548427, 33.25316411605952993 ) ) ;
#4581=CARTESIAN_POINT ( 'NONE',  ( -7.967954043666661671E-16, 18.37812499938548427, 34.33755215474603517 ) ) ;
#4596=CARTESIAN_POINT ( 'NONE',  ( 2.000000000000000444, 15.21874999877096535, 26.53589838486224650 ) ) ;
#4606=CARTESIAN_POINT ( 'NONE',  ( 1.138803498474273873E-14, 16.38124999877096499, 34.00000000000000000 ) ) ;
#4631=CARTESIAN_POINT ( 'NONE',  ( -1.626862140677534273E-15, 14.63749999999999929, 34.00000000000000000 ) ) ;
#4664=CARTESIAN_POINT ( 'NONE',  ( 2.411242101361345515E-14, 20.88124999877096499, 34.00000000000000000 ) ) ;
#4681=CARTESIAN_POINT ( 'NONE',  ( -2.000000000000001776, 19.09999999999999787, 33.46410161513775705 ) ) ;
#4688=CARTESIAN_POINT ( 'NONE',  ( 0.6840108831340462325, 20.53567971139829496, 33.87926509921195617 ) ) ;
#4700=CARTESIAN_POINT ( 'NONE',  ( 4.000000000000000000, 16.98124999877096641, 27.69059892324149885 ) ) ;
#4708=CARTESIAN_POINT ( 'NONE',  ( -1.878215178124999163, 13.24062499938548321, 26.74683588394047007 ) ) ;
#4716=CARTESIAN_POINT ( 'NONE',  ( -3.756430356249999214, 13.84062499938548463, 27.83122392262697176 ) ) ;
#4744=CARTESIAN_POINT ( 'NONE',  ( -3.756430356250001434, 16.05312499938548143, 32.16877607737301048 ) ) ;
#4746=CARTESIAN_POINT ( 'NONE',  ( 2.828200636599751609E-16, 18.01249999999999929, 25.38119784648299415 ) ) ;
#4747=CARTESIAN_POINT ( 'NONE',  ( -1.626862140677534273E-15, 17.33749999999999858, 34.00000000000000000 ) ) ;
#4822=CARTESIAN_POINT ( 'NONE',  ( 3.999999999999998668, 17.80624999877096570, 32.30940107675850470 ) ) ;
#4827=CARTESIAN_POINT ( 'NONE',  ( 1.878215178124997609, 15.37812499938548427, 33.25316411605952993 ) ) ;
#4869=CARTESIAN_POINT ( 'NONE',  ( -3.756430356250001434, 17.96562499938548285, 32.16877607737301048 ) ) ;
#4881=ORIENTED_EDGE ( 'NONE', *, *, #35090, .T. ) ;
#4893=CARTESIAN_POINT ( 'NONE',  ( -3.486133158594716510E-16, 12.61250000000000426, 26.00000000000000355 ) ) ;
#4912=EDGE_CURVE ( 'NONE', #71132, #41920, #9412, .T. ) ;
#4926=CARTESIAN_POINT ( 'NONE',  ( -3.756430356249999214, 15.52812499938548108, 27.83122392262697176 ) ) ;
#4942=CARTESIAN_POINT ( 'NONE',  ( -3.756430356250000102, 17.36562499938548498, 30.00000000000000000 ) ) ;
#4957=CARTESIAN_POINT ( 'NONE',  ( -4.000000000000000000, 14.91874999877096641, 30.00000000000000000 ) ) ;
#5070=CARTESIAN_POINT ( 'NONE',  ( -1.878215178124999163, 14.14062499938548356, 26.74683588394047007 ) ) ;
#5079=CARTESIAN_POINT ( 'NONE',  ( 1.878215178124997609, 14.02812499938548285, 33.25316411605952993 ) ) ;
#5101=VERTEX_POINT ( 'NONE', #66900 ) ;
#5105=CARTESIAN_POINT ( 'NONE',  ( -1.878215178125001827, 15.19062499938548427, 33.25316411605952283 ) ) ;
#5108=CARTESIAN_POINT ( 'NONE',  ( 2.828200636599751609E-16, 17.56250000000000000, 25.38119784648299415 ) ) ;
#5187=CARTESIAN_POINT ( 'NONE',  ( -1.878215178124999163, 15.60312499938548392, 26.74683588394047007 ) ) ;
#5227=CARTESIAN_POINT ( 'NONE',  ( -7.967954043666661671E-16, 17.59062499938548285, 34.33755215474603517 ) ) ;
#5283=CARTESIAN_POINT ( 'NONE',  ( 3.756430356250000102, 13.99062499938548498, 30.00000000000000000 ) ) ;
#5300=CARTESIAN_POINT ( 'NONE',  ( -1.878215178124999163, 18.19062499938548427, 26.74683588394047007 ) ) ;
#5308=( BOUNDED_CURVE ( )  B_SPLINE_CURVE ( 2, ( #5748, #61523, #67092, #38642, #61166, #33089, #39008, #15723, #55628 ),
 .UNSPECIFIED., .F., .F. ) 
 B_SPLINE_CURVE_WITH_KNOTS ( ( 3, 2, 2, 2, 3 ),
 ( 0.5416666666666667407, 0.5462962962962962798, 0.5555555555555555802, 0.5648148148148147696, 0.5694444444444444198 ),
 .UNSPECIFIED. ) 
 CURVE ( )  GEOMETRIC_REPRESENTATION_ITEM ( )  RATIONAL_B_SPLINE_CURVE ( ( 0.9330127018922192983, 0.9330127018922200755, 1.000000000000000000, 0.8660254037844387076, 1.000000000000000000, 0.8660254037844387076, 1.000000000000000000, 0.9330127018922194093, 0.9330127018922194093 ) ) 
 REPRESENTATION_ITEM ( '' )  );
#5318=CARTESIAN_POINT ( 'NONE',  ( 4.000000000000000000, 19.68124999877096570, 27.69059892324149530 ) ) ;
#5433=EDGE_CURVE ( 'NONE', #7083, #19771, #8098, .T. ) ;
#5439=CARTESIAN_POINT ( 'NONE',  ( -1.878215178125001827, 15.30312499938548321, 33.25316411605952283 ) ) ;
#5440=CARTESIAN_POINT ( 'NONE',  ( -1.999999999999999112, 15.29374999877096641, 26.53589838486224650 ) ) ;
#5459=CARTESIAN_POINT ( 'NONE',  ( 2.000000000000000444, 19.77500000000000213, 26.53589838486224650 ) ) ;
#5468=CARTESIAN_POINT ( 'NONE',  ( -3.756430356250001434, 15.60312499938548392, 32.16877607737301048 ) ) ;
#5471=CARTESIAN_POINT ( 'NONE',  ( 2.000000000000000444, 17.97500000000000142, 26.53589838486224650 ) ) ;
#5518=CARTESIAN_POINT ( 'NONE',  ( -3.999999999999999112, 13.08124999877096606, 27.69059892324149530 ) ) ;
#5549=DIRECTION ( 'NONE',  ( 0.000000000000000000, 0.000000000000000000, -1.000000000000000000 ) ) ;
#5553=CARTESIAN_POINT ( 'NONE',  ( 2.655984681222220721E-16, 15.56562499938548250, 25.66244784525396483 ) ) ;
#5583=EDGE_CURVE ( 'NONE', #3561, #64855, #13260, .T. ) ;
#5597=CARTESIAN_POINT ( 'NONE',  ( 3.756430356249998770, 16.76562499938548356, 32.16877607737302469 ) ) ;
#5653=CARTESIAN_POINT ( 'NONE',  ( 1.878215178125000495, 13.61562499938548321, 26.74683588394047007 ) ) ;
#5668=CARTESIAN_POINT ( 'NONE',  ( 1.878215178124997609, 18.86562499938548143, 33.25316411605952993 ) ) ;
#5682=CARTESIAN_POINT ( 'NONE',  ( -4.000000000000000888, 18.10624999877096641, 32.30940107675850470 ) ) ;
#5701=EDGE_CURVE ( 'NONE', #68118, #41920, #63150, .T. ) ;
#5707=( BOUNDED_CURVE ( )  B_SPLINE_CURVE ( 2, ( #19430, #26091, #3936, #41991, #59694, #48629, #31639, #71154, #26459 ),
 .UNSPECIFIED., .F., .F. ) 
 B_SPLINE_CURVE_WITH_KNOTS ( ( 3, 2, 2, 2, 3 ),
 ( 0.6250000000000000000, 0.6296296296296296502, 0.6388888888888888395, 0.6481481481481481399, 0.6527777777777777901 ),
 .UNSPECIFIED. ) 
 CURVE ( )  GEOMETRIC_REPRESENTATION_ITEM ( )  RATIONAL_B_SPLINE_CURVE ( ( 0.9330127018922194093, 0.9330127018922194093, 1.000000000000000000, 0.8660254037844387076, 1.000000000000000000, 0.8660254037844387076, 1.000000000000000000, 0.9330127018922194093, 0.9330127018922194093 ) ) 
 REPRESENTATION_ITEM ( '' )  );
#5722=EDGE_CURVE ( 'NONE', #68198, #11370, #43043, .T. ) ;
#5748=CARTESIAN_POINT ( 'NONE',  ( 2.393811435568372112E-14, 17.28124999877096712, 34.00000000000000000 ) ) ;
#5764=( BOUNDED_CURVE ( )  B_SPLINE_CURVE ( 2, ( #12387, #7934, #30472, #36375, #13457, #58524, #17914, #62992, #35282 ),
 .UNSPECIFIED., .F., .F. ) 
 B_SPLINE_CURVE_WITH_KNOTS ( ( 3, 2, 2, 2, 3 ),
 ( 0.7638888888888889506, 0.7685185185185184897, 0.7777777777777777901, 0.7870370370370370905, 0.7916666666666667407 ),
 .UNSPECIFIED. ) 
 CURVE ( )  GEOMETRIC_REPRESENTATION_ITEM ( )  RATIONAL_B_SPLINE_CURVE ( ( 0.9330127018922192983, 0.9330127018922200755, 1.000000000000000000, 0.8660254037844387076, 1.000000000000000000, 0.8660254037844387076, 1.000000000000000000, 0.9330127018922185211, 0.9330127018922192983 ) ) 
 REPRESENTATION_ITEM ( '' )  );
#5798=CARTESIAN_POINT ( 'NONE',  ( -7.967954043666661671E-16, 15.79062499938548392, 34.33755215474603517 ) ) ;
#5808=ORIENTED_EDGE ( 'NONE', *, *, #65184, .T. ) ;
#5829=CARTESIAN_POINT ( 'NONE',  ( -4.000000000000000888, 16.81250000000000000, 32.30940107675850470 ) ) ;
#5878=EDGE_CURVE ( 'NONE', #51815, #71973, #18010, .T. ) ;
#5908=CARTESIAN_POINT ( 'NONE',  ( 3.756430356250000546, 15.49062499938548321, 27.83122392262697886 ) ) ;
#5950=CARTESIAN_POINT ( 'NONE',  ( -1.878215178124999163, 16.95312499938548356, 26.74683588394047007 ) ) ;
#6006=CARTESIAN_POINT ( 'NONE',  ( 3.756430356250000102, 16.69062499938548427, 30.00000000000000000 ) ) ;
#6038=CARTESIAN_POINT ( 'NONE',  ( 2.828200636599751609E-16, 17.50624999877096499, 25.38119784648299415 ) ) ;
#6118=EDGE_CURVE ( 'NONE', #2103, #38096, #2920, .T. ) ;
#6153=CARTESIAN_POINT ( 'NONE',  ( 1.999999999999997335, 13.77500000000000036, 33.46410161513775705 ) ) ;
#6159=CARTESIAN_POINT ( 'NONE',  ( 3.756430356250000102, 15.90312499938548108, 30.00000000000000000 ) ) ;
#6165=CARTESIAN_POINT ( 'NONE',  ( 0.000000000000000000, 12.50000000000000000, 30.00000000000000000 ) ) ;
#6190=CARTESIAN_POINT ( 'NONE',  ( -1.999999999999999112, 20.29999999999999716, 26.53589838486224650 ) ) ;
#6209=EDGE_CURVE ( 'NONE', #51293, #9005, #5308, .T. ) ;
#6238=DIRECTION ( 'NONE',  ( -0.000000000000000000, -1.000000000000000000, -0.000000000000000000 ) ) ;
#6268=CYLINDRICAL_SURFACE ( 'NONE', #13559, 4.000000000000000000 ) ;
#6272=CARTESIAN_POINT ( 'NONE',  ( 1.878215178125000495, 17.77812499938548285, 26.74683588394047007 ) ) ;
#6281=CARTESIAN_POINT ( 'NONE',  ( -1.999999999999999112, 16.25000000000000000, 26.53589838486224650 ) ) ;
#6299=ORIENTED_EDGE ( 'NONE', *, *, #43763, .F. ) ;
#6313=CARTESIAN_POINT ( 'NONE',  ( 1.878215178124997609, 18.07812499938548356, 33.25316411605952993 ) ) ;
#6337=CARTESIAN_POINT ( 'NONE',  ( -1.243387493232115393E-14, 15.25624999877096677, 26.00000000000000000 ) ) ;
#6351=CARTESIAN_POINT ( 'NONE',  ( -1.071796769724492115, 15.91115380933863577, 34.00000000000000000 ) ) ;
#6367=CARTESIAN_POINT ( 'NONE',  ( 1.878215178125000495, 16.31562499938548427, 26.74683588394047007 ) ) ;
#6369=DIRECTION ( 'NONE',  ( -0.000000000000000000, -1.000000000000000000, -0.000000000000000000 ) ) ;
#6401=CARTESIAN_POINT ( 'NONE',  ( -8.484601909799255319E-16, 18.63124999877096499, 34.61880215351700940 ) ) ;
#6427=CARTESIAN_POINT ( 'NONE',  ( 1.071796769724485232, 14.84240381056766545, 25.99999999999999645 ) ) ;
#6504=AXIS2_PLACEMENT_3D ( 'NONE', #54407, #65850, #43691 ) ;
#6526=CARTESIAN_POINT ( 'NONE',  ( -3.756430356249999214, 17.44062499938548072, 27.83122392262697176 ) ) ;
#6535=ORIENTED_EDGE ( 'NONE', *, *, #67586, .T. ) ;
#6551=ORIENTED_EDGE ( 'NONE', *, *, #19199, .T. ) ;
#6558=CARTESIAN_POINT ( 'NONE',  ( -8.484601909799255319E-16, 20.03750000000000142, 34.61880215351700940 ) ) ;
#6598=CARTESIAN_POINT ( 'NONE',  ( 0.000000000000000000, 27.50000000000000000, 30.00000000000000000 ) ) ;
#6627=DIRECTION ( 'NONE',  ( -0.000000000000000000, -1.000000000000000000, -0.000000000000000000 ) ) ;
#6636=FACE_OUTER_BOUND ( 'NONE', #28702, .T. ) ;
#6644=CARTESIAN_POINT ( 'NONE',  ( -3.756430356250000102, 18.37812499938548427, 30.00000000000000000 ) ) ;
#6646=CARTESIAN_POINT ( 'NONE',  ( 4.000000000000000000, 13.40000000000000036, 30.00000000000000000 ) ) ;
#6654=EDGE_LOOP ( 'NONE', ( #64634, #28623, #38613, #16531 ) ) ;
#6681=CARTESIAN_POINT ( 'NONE',  ( 1.878215178125000495, 19.12812499938548427, 26.74683588394047007 ) ) ;
#6705=CARTESIAN_POINT ( 'NONE',  ( 4.000000000000000000, 15.14374999877096606, 30.00000000000000000 ) ) ;
#6734=CARTESIAN_POINT ( 'NONE',  ( 3.756430356249998770, 16.20312499938548356, 32.16877607737301759 ) ) ;
#6752=ORIENTED_EDGE ( 'NONE', *, *, #66773, .T. ) ;
#6763=CARTESIAN_POINT ( 'NONE',  ( 3.756430356249998770, 13.16562499938548392, 32.16877607737302469 ) ) ;
#6790=DIRECTION ( 'NONE',  ( -0.000000000000000000, -1.000000000000000000, -0.000000000000000000 ) ) ;
#6816=EDGE_LOOP ( 'NONE', ( #69077, #71287, #68155, #926 ) ) ;
#6824=CARTESIAN_POINT ( 'NONE',  ( -1.878215178124999163, 15.94062499938548427, 26.74683588394047007 ) ) ;
#6844=DIRECTION ( 'NONE',  ( 0.000000000000000000, 0.000000000000000000, -1.000000000000000000 ) ) ;
#6886=CARTESIAN_POINT ( 'NONE',  ( 3.756430356250000102, 16.35312499938548569, 30.00000000000000000 ) ) ;
#6918=CARTESIAN_POINT ( 'NONE',  ( 4.000000000000000000, 19.25000000000000000, 30.00000000000000000 ) ) ;
#6954=CARTESIAN_POINT ( 'NONE',  ( 4.000000000000000000, 15.59374999877096535, 30.00000000000000000 ) ) ;
#6999=CARTESIAN_POINT ( 'NONE',  ( -1.878215178125001827, 18.90312499938548285, 33.25316411605952283 ) ) ;
#7001=CARTESIAN_POINT ( 'NONE',  ( 3.756430356249998770, 20.25312499938547717, 32.16877607737302469 ) ) ;
#7010=ORIENTED_EDGE ( 'NONE', *, *, #39141, .T. ) ;
#7038=CARTESIAN_POINT ( 'NONE',  ( 1.878215178124997609, 18.97812499938548214, 33.25316411605952993 ) ) ;
#7063=CARTESIAN_POINT ( 'NONE',  ( 0.000000000000000000, 27.50000000000000000, 30.00000000000000000 ) ) ;
#7083=VERTEX_POINT ( 'NONE', #46833 ) ;
#7092=LINE ( 'NONE', #34795, #1877 ) ;
#7094=CARTESIAN_POINT ( 'NONE',  ( -1.878215178124999163, 17.74062499938548498, 26.74683588394047007 ) ) ;
#7096=VERTEX_POINT ( 'NONE', #36831 ) ;
#7123=CARTESIAN_POINT ( 'NONE',  ( 2.655984681222220721E-16, 13.76562499938548179, 25.66244784525396483 ) ) ;
#7185=CARTESIAN_POINT ( 'NONE',  ( 3.756430356249998770, 18.00312499938548427, 32.16877607737302469 ) ) ;
#7203=CARTESIAN_POINT ( 'NONE',  ( 0.000000000000000000, 27.50000000000000000, 30.00000000000000000 ) ) ;
#7206=SHAPE_REPRESENTATION_RELATIONSHIP ( 'NONE' , 'NONE' ,  #46217, #30285 ) ;
#7210=CARTESIAN_POINT ( 'NONE',  ( -1.999999999999999112, 14.39374999877096606, 26.53589838486224650 ) ) ;
#7221=ADVANCED_FACE ( 'NONE', ( #9493 ), #17110, .T. ) ;
#7237=CARTESIAN_POINT ( 'NONE',  ( 1.138803498474273873E-14, 15.98750000000000249, 34.00000000000000000 ) ) ;
#7244=CARTESIAN_POINT ( 'NONE',  ( -7.967954043666661671E-16, 16.69062499938548427, 34.33755215474603517 ) ) ;
#7295=CARTESIAN_POINT ( 'NONE',  ( 0.000000000000000000, 27.50000000000000000, 26.00000000000000000 ) ) ;
#7315=CARTESIAN_POINT ( 'NONE',  ( 1.999999999999997335, 14.22499999999999964, 33.46410161513775705 ) ) ;
#7316=DIRECTION ( 'NONE',  ( -0.000000000000000000, -1.000000000000000000, -0.000000000000000000 ) ) ;
#7341=CARTESIAN_POINT ( 'NONE',  ( 3.973779386032386007, 25.00705285313813775, 30.52704257968602874 ) ) ;
#7358=CARTESIAN_POINT ( 'NONE',  ( -3.756430356249999214, 19.24062499938548143, 27.83122392262697531 ) ) ;
#7360=CARTESIAN_POINT ( 'NONE',  ( 1.878215178125000495, 20.36562499938548143, 26.74683588394047007 ) ) ;
#7398=CARTESIAN_POINT ( 'NONE',  ( 3.756430356250000102, 19.50312499938548072, 30.00000000000000000 ) ) ;
#7437=CARTESIAN_POINT ( 'NONE',  ( 4.898850051585143718E-16, 25.54316770519903557, 34.00000000000000000 ) ) ;
#7453=CARTESIAN_POINT ( 'NONE',  ( -1.878215178124999163, 18.19062499938548427, 26.74683588394047007 ) ) ;
#7465=CARTESIAN_POINT ( 'NONE',  ( -2.000000000000001776, 15.50000000000000000, 33.46410161513775705 ) ) ;
#7482=CARTESIAN_POINT ( 'NONE',  ( -1.878215178125001827, 13.05312499938548321, 33.25316411605952283 ) ) ;
#7541=CARTESIAN_POINT ( 'NONE',  ( 1.878215178124997609, 16.61562499938548143, 33.25316411605952993 ) ) ;
#7559=CARTESIAN_POINT ( 'NONE',  ( 5.810221930991193690E-16, 17.56250000000000000, 26.00000000000000000 ) ) ;
#7565=CARTESIAN_POINT ( 'NONE',  ( 2.000000000000000444, 13.86874999877096748, 26.53589838486224650 ) ) ;
#7598=CARTESIAN_POINT ( 'NONE',  ( 1.878215178125000495, 16.87812499938548072, 26.74683588394047007 ) ) ;
#7634=CARTESIAN_POINT ( 'NONE',  ( 2.000000000000000444, 20.22500000000000142, 26.53589838486224650 ) ) ;
#7652=DIRECTION ( 'NONE',  ( -0.000000000000000000, -1.000000000000000000, -0.000000000000000000 ) ) ;
#7695=CARTESIAN_POINT ( 'NONE',  ( 0.000000000000000000, 27.50000000000000000, 30.00000000000000000 ) ) ;
#7701=CARTESIAN_POINT ( 'NONE',  ( 1.777890502354250168, 25.43624258734061883, 26.40726507414123958 ) ) ;
#7720=CARTESIAN_POINT ( 'NONE',  ( 3.756430356250000102, 19.50312499938548072, 30.00000000000000000 ) ) ;
#7722=CARTESIAN_POINT ( 'NONE',  ( -7.967954043666661671E-16, 20.17812499938548143, 34.33755215474603517 ) ) ;
#7727=CARTESIAN_POINT ( 'NONE',  ( -1.999999999999999112, 18.05000000000000071, 26.53589838486224650 ) ) ;
#7759=CARTESIAN_POINT ( 'NONE',  ( 2.655984681222220721E-16, 20.06562499938548427, 25.66244784525396483 ) ) ;
#7770=VECTOR ( 'NONE', #37424, 1000.000000000000000 ) ;
#7773=UNCERTAINTY_MEASURE_WITH_UNIT (LENGTH_MEASURE( 1.000000000000000082E-05 ), #51324, 'distance_accuracy_value', 'NONE');
#7791=EDGE_CURVE ( 'NONE', #69714, #31816, #12842, .T. ) ;
#7801=CARTESIAN_POINT ( 'NONE',  ( -1.778782919078051528, 25.43611513164544036, 26.40779114962846919 ) ) ;
#7818=CARTESIAN_POINT ( 'NONE',  ( 1.878215178124997609, 19.76562499938548356, 33.25316411605952993 ) ) ;
#7827=CARTESIAN_POINT ( 'NONE',  ( 4.898587196589412829E-16, 27.50000000000000000, 34.00000000000000000 ) ) ;
#7848=CARTESIAN_POINT ( 'NONE',  ( 2.828200636599751609E-16, 19.75624999877096499, 25.38119784648299415 ) ) ;
#7856=CARTESIAN_POINT ( 'NONE',  ( 4.000000000000000000, 18.83749999999999858, 27.69059892324149885 ) ) ;
#7899=ORIENTED_EDGE ( 'NONE', *, *, #3547, .F. ) ;
#7907=CARTESIAN_POINT ( 'NONE',  ( 1.878215178124997609, 17.96562499938548285, 33.25316411605952993 ) ) ;
#7918=CARTESIAN_POINT ( 'NONE',  ( 3.756430356249998770, 15.30312499938548498, 32.16877607737302469 ) ) ;
#7931=CARTESIAN_POINT ( 'NONE',  ( 2.000000000000000444, 14.31874999877096499, 26.53589838486224650 ) ) ;
#7934=CARTESIAN_POINT ( 'NONE',  ( 1.071796769724500997, 19.10134618820330132, 33.99999999999999289 ) ) ;
#7966=CARTESIAN_POINT ( 'NONE',  ( 3.756430356250000546, 16.39062499938548356, 27.83122392262697886 ) ) ;
#8006=CARTESIAN_POINT ( 'NONE',  ( 4.000000000000000000, 12.89374999877096606, 30.00000000000000000 ) ) ;
#8018=ORIENTED_EDGE ( 'NONE', *, *, #69480, .T. ) ;
#8030=( BOUNDED_CURVE ( )  B_SPLINE_CURVE ( 2, ( #30191, #52720, #47184, #59338, #19084, #8749, #41639, #13546, #36093 ),
 .UNSPECIFIED., .F., .F. ) 
 B_SPLINE_CURVE_WITH_KNOTS ( ( 3, 2, 2, 2, 3 ),
 ( 0.8194444444444444198, 0.8240740740740740700, 0.8333333333333333703, 0.8425925925925925597, 0.8472222222222222099 ),
 .UNSPECIFIED. ) 
 CURVE ( )  GEOMETRIC_REPRESENTATION_ITEM ( )  RATIONAL_B_SPLINE_CURVE ( ( 0.9330127018922194093, 0.9330127018922194093, 1.000000000000000000, 0.8660254037844387076, 1.000000000000000000, 0.8660254037844387076, 1.000000000000000000, 0.9330127018922194093, 0.9330127018922194093 ) ) 
 REPRESENTATION_ITEM ( '' )  );
#8038=ORIENTED_EDGE ( 'NONE', *, *, #72602, .F. ) ;
#8042=CARTESIAN_POINT ( 'NONE',  ( 0.000000000000000000, 27.50000000000000000, 30.00000000000000000 ) ) ;
#8057=LINE ( 'NONE', #64567, #38452 ) ;
#8069=CARTESIAN_POINT ( 'NONE',  ( 0.2617799820177835191, 25.54316770519903201, 34.00000000000000000 ) ) ;
#8086=CARTESIAN_POINT ( 'NONE',  ( -3.756430356250001434, 13.35312499938548392, 32.16877607737301048 ) ) ;
#8088=CARTESIAN_POINT ( 'NONE',  ( 4.000000000000000000, 12.98749999999999893, 27.69059892324149530 ) ) ;
#8093=CARTESIAN_POINT ( 'NONE',  ( -4.000000000000000000, 18.12500000000000355, 30.00000000000000000 ) ) ;
#8098=( BOUNDED_CURVE ( )  B_SPLINE_CURVE ( 1, ( #50986, #45087 ),
 .UNSPECIFIED., .F., .F. ) 
 B_SPLINE_CURVE_WITH_KNOTS ( ( 2, 2 ),
 ( 0.000000000000000000, 1.000000000000000000 ),
 .UNSPECIFIED. ) 
 CURVE ( )  GEOMETRIC_REPRESENTATION_ITEM ( )  RATIONAL_B_SPLINE_CURVE ( ( 0.9401540804404022733, 0.9401540804404022733 ) ) 
 REPRESENTATION_ITEM ( '' )  );
#8128=CARTESIAN_POINT ( 'NONE',  ( -1.878215178125001827, 19.35312499938548214, 33.25316411605952283 ) ) ;
#8138=ORIENTED_EDGE ( 'NONE', *, *, #48242, .F. ) ;
#8164=CARTESIAN_POINT ( 'NONE',  ( -3.012979756977046897, 25.23363074891087265, 27.35627862958216738 ) ) ;
#8180=CARTESIAN_POINT ( 'NONE',  ( 1.878215178124997609, 18.41562499938548214, 33.25316411605952993 ) ) ;
#8182=ORIENTED_EDGE ( 'NONE', *, *, #4284, .T. ) ;
#8200=EDGE_LOOP ( 'NONE', ( #41656, #25321, #68798, #8038 ) ) ;
#8212=CARTESIAN_POINT ( 'NONE',  ( 1.878215178125000495, 12.82812499938548356, 26.74683588394047007 ) ) ;
#8258=DIRECTION ( 'NONE',  ( -0.000000000000000000, -1.000000000000000000, -0.000000000000000000 ) ) ;
#8274=CARTESIAN_POINT ( 'NONE',  ( -7.967954043666661671E-16, 17.47812499938548214, 34.33755215474603517 ) ) ;
#8283=CARTESIAN_POINT ( 'NONE',  ( -1.878215178125001827, 16.54062499938548569, 33.25316411605952283 ) ) ;
#8298=CARTESIAN_POINT ( 'NONE',  ( -4.000000000000000888, 13.15624999877096535, 32.30940107675850470 ) ) ;
#8308=( BOUNDED_CURVE ( )  B_SPLINE_CURVE ( 2, ( #19130, #69411, #25420, #64207, #19497, #42055, #59024, #47963, #4370 ),
 .UNSPECIFIED., .F., .F. ) 
 B_SPLINE_CURVE_WITH_KNOTS ( ( 3, 2, 2, 2, 3 ),
 ( 0.09722222222222222376, 0.1018518518518518462, 0.1111111111111111049, 0.1203703703703703637, 0.1250000000000000000 ),
 .UNSPECIFIED. ) 
 CURVE ( )  GEOMETRIC_REPRESENTATION_ITEM ( )  RATIONAL_B_SPLINE_CURVE ( ( 0.9330127018922192983, 0.9330127018922194093, 1.000000000000000000, 0.8660254037844387076, 1.000000000000000000, 0.8660254037844387076, 1.000000000000000000, 0.9330127018922191873, 0.9330127018922192983 ) ) 
 REPRESENTATION_ITEM ( '' )  );
#8329=CARTESIAN_POINT ( 'NONE',  ( -3.756430356250000102, 18.37812499938548427, 30.00000000000000000 ) ) ;
#8425=CARTESIAN_POINT ( 'NONE',  ( 3.012598849231780118, 25.23371056053735728, 27.35582546009486649 ) ) ;
#8436=DIRECTION ( 'NONE',  ( -0.000000000000000000, -1.000000000000000000, -0.000000000000000000 ) ) ;
#8445=CARTESIAN_POINT ( 'NONE',  ( -3.756430356249999214, 13.27812499938548463, 27.83122392262697531 ) ) ;
#8447=CARTESIAN_POINT ( 'NONE',  ( -4.000000000000000000, 14.97499999999999964, 30.00000000000000000 ) ) ;
#8452=( BOUNDED_CURVE ( )  B_SPLINE_CURVE ( 2, ( #20644, #30001, #60166, #9576, #32108, #52544, #54641, #41108, #4046 ),
 .UNSPECIFIED., .F., .F. ) 
 B_SPLINE_CURVE_WITH_KNOTS ( ( 3, 2, 2, 2, 3 ),
 ( 0.7083333333333333703, 0.7129629629629629095, 0.7222222222222222099, 0.7314814814814815103, 0.7361111111111111605 ),
 .UNSPECIFIED. ) 
 CURVE ( )  GEOMETRIC_REPRESENTATION_ITEM ( )  RATIONAL_B_SPLINE_CURVE ( ( 0.9330127018922192983, 0.9330127018922200755, 1.000000000000000000, 0.8660254037844387076, 1.000000000000000000, 0.8660254037844387076, 1.000000000000000000, 0.9330127018922185211, 0.9330127018922192983 ) ) 
 REPRESENTATION_ITEM ( '' )  );
#8531=CARTESIAN_POINT ( 'NONE',  ( 3.756430356250000546, 13.69062499938548250, 27.83122392262697886 ) ) ;
#8545=CARTESIAN_POINT ( 'NONE',  ( -7.967954043666661671E-16, 18.37812499938548427, 34.33755215474603517 ) ) ;
#8576=CARTESIAN_POINT ( 'NONE',  ( -1.878215178124999163, 14.70312499938548356, 26.74683588394047007 ) ) ;
#8584=CARTESIAN_POINT ( 'NONE',  ( 2.393811435568372112E-14, 18.68750000000000355, 34.00000000000000000 ) ) ;
#8637=CARTESIAN_POINT ( 'NONE',  ( -1.878215178125001827, 16.54062499938548569, 33.25316411605952283 ) ) ;
#8646=CARTESIAN_POINT ( 'NONE',  ( -1.878215178125001827, 16.09062499938548285, 33.25316411605952283 ) ) ;
#8654=CARTESIAN_POINT ( 'NONE',  ( 4.648177544792955741E-15, 13.73749999999999716, 33.99999999999999289 ) ) ;
#8662=CARTESIAN_POINT ( 'NONE',  ( 3.999999999999998668, 13.75624999877096677, 32.30940107675850470 ) ) ;
#8686=CARTESIAN_POINT ( 'NONE',  ( 2.393811435568372112E-14, 18.68750000000000355, 34.00000000000000000 ) ) ;
#8694=CARTESIAN_POINT ( 'NONE',  ( 3.756430356249998770, 20.36562499938548143, 32.16877607737301759 ) ) ;
#8695=CARTESIAN_POINT ( 'NONE',  ( 4.898587196589407898E-16, 12.50000000000000000, 34.00000000000000000 ) ) ;
#8725=CARTESIAN_POINT ( 'NONE',  ( -2.498395430326213790E-14, 18.91249999999999787, 26.00000000000000000 ) ) ;
#8749=CARTESIAN_POINT ( 'NONE',  ( 4.000000000000000000, 19.68124999877096570, 27.69059892324149885 ) ) ;
#8787=CARTESIAN_POINT ( 'NONE',  ( 1.999999999999997335, 16.92500000000000071, 33.46410161513775705 ) ) ;
#8790=DIRECTION ( 'NONE',  ( 0.000000000000000000, 0.000000000000000000, -1.000000000000000000 ) ) ;
#8814=CARTESIAN_POINT ( 'NONE',  ( 2.655984681222220721E-16, 19.61562499938548143, 25.66244784525396483 ) ) ;
#8816=CARTESIAN_POINT ( 'NONE',  ( 1.999999999999997335, 15.57500000000000107, 33.46410161513775705 ) ) ;
#8829=CARTESIAN_POINT ( 'NONE',  ( 4.898587196589412829E-16, 27.50000000000000000, 34.00000000000000000 ) ) ;
#8874=VECTOR ( 'NONE', #3541, 1000.000000000000000 ) ;
#8899=CARTESIAN_POINT ( 'NONE',  ( -3.179521419646683889, 25.19832693812782054, 32.44092611819090166 ) ) ;
#8903=EDGE_CURVE ( 'NONE', #16877, #35360, #45857, .T. ) ;
#8904=CARTESIAN_POINT ( 'NONE',  ( -1.878215178125001827, 13.95312499938548356, 33.25316411605952283 ) ) ;
#8915=CARTESIAN_POINT ( 'NONE',  ( -3.756430356250000990, 19.20312499938548356, 32.16877607737301048 ) ) ;
#8942=VERTEX_POINT ( 'NONE', #1316 ) ;
#8946=CARTESIAN_POINT ( 'NONE',  ( -7.967954043666661671E-16, 15.34062499938548463, 34.33755215474603517 ) ) ;
#8976=CARTESIAN_POINT ( 'NONE',  ( -1.243387493232115393E-14, 15.76249999999999929, 26.00000000000000000 ) ) ;
#8994=VERTEX_POINT ( 'NONE', #22387 ) ;
#8999=CARTESIAN_POINT ( 'NONE',  ( -4.000000000000000000, 16.71874999877096712, 30.00000000000000000 ) ) ;
#9002=CARTESIAN_POINT ( 'NONE',  ( -7.967954043666661671E-16, 13.42812499938548321, 34.33755215474603517 ) ) ;
#9005=VERTEX_POINT ( 'NONE', #62279 ) ;
#9009=CARTESIAN_POINT ( 'NONE',  ( 3.756430356249998770, 19.35312499938548214, 32.16877607737302469 ) ) ;
#9012=ADVANCED_FACE ( 'NONE', ( #36372 ), #30469, .T. ) ;
#9020=CARTESIAN_POINT ( 'NONE',  ( -1.878215178124999163, 16.84062499938548285, 26.74683588394047007 ) ) ;
#9028=CARTESIAN_POINT ( 'NONE',  ( -1.626862140677534273E-15, 16.43750000000000000, 34.00000000000000000 ) ) ;
#9035=CARTESIAN_POINT ( 'NONE',  ( -1.999999999999999112, 17.09374999877096712, 26.53589838486224650 ) ) ;
#9044=CARTESIAN_POINT ( 'NONE',  ( 3.756430356250000102, 12.75312499938548427, 30.00000000000000000 ) ) ;
#9054=ADVANCED_FACE ( 'NONE', ( #25280 ), #55781, .T. ) ;
#9063=CARTESIAN_POINT ( 'NONE',  ( -2.000000000000001776, 12.80000000000000071, 33.46410161513775705 ) ) ;
#9066=CARTESIAN_POINT ( 'NONE',  ( 3.756430356250000546, 20.44062499938548427, 27.83122392262697886 ) ) ;
#9090=CARTESIAN_POINT ( 'NONE',  ( 4.000000000000000000, 14.24374999877096748, 30.00000000000000000 ) ) ;
#9153=LINE ( 'NONE', #21686, #65597 ) ;
#9183=CARTESIAN_POINT ( 'NONE',  ( 1.878215178125000495, 20.47812499938548569, 26.74683588394047007 ) ) ;
#9185=CARTESIAN_POINT ( 'NONE',  ( -4.000000000000000888, 14.56250000000000000, 32.30940107675850470 ) ) ;
#9186=CARTESIAN_POINT ( 'NONE',  ( -2.000000000000001776, 17.30000000000000071, 33.46410161513775705 ) ) ;
#9222=EDGE_LOOP ( 'NONE', ( #42752, #16126, #24636, #20805 ) ) ;
#9253=CARTESIAN_POINT ( 'NONE',  ( -2.498395430326213790E-14, 18.85624999877096641, 26.00000000000000000 ) ) ;
#9264=CARTESIAN_POINT ( 'NONE',  ( 1.071796769724488785, 17.75134618820329635, 34.00000000000000000 ) ) ;
#9268=CARTESIAN_POINT ( 'NONE',  ( -1.878215178125001827, 14.40312499938548463, 33.25316411605952283 ) ) ;
#9280=CARTESIAN_POINT ( 'NONE',  ( 2.655984681222220721E-16, 19.05312499938548143, 25.66244784525396483 ) ) ;
#9292=CARTESIAN_POINT ( 'NONE',  ( 1.999999999999997335, 14.61874999877096570, 33.46410161513775705 ) ) ;
#9312=CARTESIAN_POINT ( 'NONE',  ( -7.967954043666661671E-16, 14.44062499938548427, 34.33755215474603517 ) ) ;
#9384=CARTESIAN_POINT ( 'NONE',  ( -1.878215178125001827, 15.19062499938548427, 33.25316411605952283 ) ) ;
#9394=CARTESIAN_POINT ( 'NONE',  ( 1.138803498474273873E-14, 15.08749999999999858, 34.00000000000000000 ) ) ;
#9400=CARTESIAN_POINT ( 'NONE',  ( 4.000000000000000000, 15.63124999877096499, 27.69059892324149530 ) ) ;
#9412=( BOUNDED_CURVE ( )  B_SPLINE_CURVE ( 2, ( #26642, #38076, #32542, #55080, #4480, #27370, #72063, #21443, #14807 ),
 .UNSPECIFIED., .F., .F. ) 
 B_SPLINE_CURVE_WITH_KNOTS ( ( 3, 2, 2, 2, 3 ),
 ( 0.4305555555555555802, 0.4351851851851851749, 0.4444444444444444198, 0.4537037037037037202, 0.4583333333333333703 ),
 .UNSPECIFIED. ) 
 CURVE ( )  GEOMETRIC_REPRESENTATION_ITEM ( )  RATIONAL_B_SPLINE_CURVE ( ( 0.9330127018922194093, 0.9330127018922197424, 1.000000000000000000, 0.8660254037844387076, 1.000000000000000000, 0.8660254037844387076, 1.000000000000000000, 0.9330127018922189652, 0.9330127018922194093 ) ) 
 REPRESENTATION_ITEM ( '' )  );
#9433=CARTESIAN_POINT ( 'NONE',  ( -1.878215178125001827, 19.35312499938548214, 33.25316411605952283 ) ) ;
#9443=CARTESIAN_POINT ( 'NONE',  ( -1.071796769724479903, 20.46740381056766367, 34.00000000000000000 ) ) ;
#9493=FACE_OUTER_BOUND ( 'NONE', #36924, .T. ) ;
#9505=CARTESIAN_POINT ( 'NONE',  ( 0.000000000000000000, 27.50000000000000000, 26.00000000000000000 ) ) ;
#9513=CARTESIAN_POINT ( 'NONE',  ( 2.655984681222220721E-16, 14.10312499938548392, 25.66244784525396483 ) ) ;
#9517=ADVANCED_FACE ( 'NONE', ( #45034 ), #66468, .T. ) ;
#9525=CARTESIAN_POINT ( 'NONE',  ( -2.498395430326213790E-14, 16.66250000000000497, 26.00000000000000000 ) ) ;
#9544=CARTESIAN_POINT ( 'NONE',  ( 5.810221930991193690E-16, 14.80624999877096570, 26.00000000000000000 ) ) ;
#9548=CARTESIAN_POINT ( 'NONE',  ( 1.878215178125000495, 13.16562499938548392, 26.74683588394047007 ) ) ;
#9550=CARTESIAN_POINT ( 'NONE',  ( 4.000000000000000000, 16.13749999999999929, 27.69059892324149530 ) ) ;
#9576=CARTESIAN_POINT ( 'NONE',  ( 3.999999999999998668, 18.70624999877096784, 32.30940107675850470 ) ) ;
#9585=VERTEX_POINT ( 'NONE', #22484 ) ;
#9634=CARTESIAN_POINT ( 'NONE',  ( -7.967954043666661671E-16, 13.99062499938548498, 34.33755215474603517 ) ) ;
#9677=CARTESIAN_POINT ( 'NONE',  ( 3.756430356250000546, 14.59062499938548463, 27.83122392262697886 ) ) ;
#9729=CARTESIAN_POINT ( 'NONE',  ( 1.878215178124997609, 14.36562499938548321, 33.25316411605952993 ) ) ;
#9736=CARTESIAN_POINT ( 'NONE',  ( -3.756430356249999214, 19.12812499938548427, 27.83122392262697531 ) ) ;
#9745=CARTESIAN_POINT ( 'NONE',  ( 1.878215178124997609, 19.31562499938548427, 33.25316411605952993 ) ) ;
#9760=CARTESIAN_POINT ( 'NONE',  ( -3.999999999999999556, 15.33124999877096606, 27.69059892324149175 ) ) ;
#9792=CARTESIAN_POINT ( 'NONE',  ( 1.878215178124997609, 18.97812499938548214, 33.25316411605952993 ) ) ;
#9845=DIRECTION ( 'NONE',  ( 0.000000000000000000, 0.000000000000000000, -1.000000000000000000 ) ) ;
#9867=CARTESIAN_POINT ( 'NONE',  ( 4.000000000000000000, 16.94374999877096499, 30.00000000000000000 ) ) ;
#9875=CARTESIAN_POINT ( 'NONE',  ( -1.878215178124999163, 14.59062499938548463, 26.74683588394047007 ) ) ;
#9884=CARTESIAN_POINT ( 'NONE',  ( 1.878215178125000495, 12.82812499938548356, 26.74683588394047007 ) ) ;
#9901=CARTESIAN_POINT ( 'NONE',  ( 1.999999999999997335, 19.62500000000000000, 33.46410161513775705 ) ) ;
#9910=CARTESIAN_POINT ( 'NONE',  ( -1.878215178125001827, 14.74062499938548321, 33.25316411605952283 ) ) ;
#9912=CARTESIAN_POINT ( 'NONE',  ( 4.000000000000000000, 14.33750000000000213, 27.69059892324149530 ) ) ;
#9913=CARTESIAN_POINT ( 'NONE',  ( -1.999999999999999112, 17.14999999999999858, 26.53589838486224650 ) ) ;
#9966=CARTESIAN_POINT ( 'NONE',  ( 2.000000000000000444, 12.96874999877096712, 26.53589838486224650 ) ) ;
#9976=CARTESIAN_POINT ( 'NONE',  ( 0.000000000000000000, 27.50000000000000000, 26.00000000000000000 ) ) ;
#9983=AXIS2_PLACEMENT_3D ( 'NONE', #71711, #4116, #72428 ) ;
#9999=CARTESIAN_POINT ( 'NONE',  ( -3.756430356249999214, 13.84062499938548463, 27.83122392262697531 ) ) ;
#10043=CARTESIAN_POINT ( 'NONE',  ( 1.878215178124997609, 14.47812499938548214, 33.25316411605952993 ) ) ;
#10057=CIRCLE ( 'NONE', #23005, 4.000000000000003553 ) ;
#10101=CARTESIAN_POINT ( 'NONE',  ( -1.878215178124999163, 14.59062499938548463, 26.74683588394047007 ) ) ;
#10106=CARTESIAN_POINT ( 'NONE',  ( -7.967954043666661671E-16, 19.72812499938548214, 34.33755215474603517 ) ) ;
#10115=CARTESIAN_POINT ( 'NONE',  ( -1.878215178125001827, 17.44062499938548072, 33.25316411605952283 ) ) ;
#10125=CARTESIAN_POINT ( 'NONE',  ( 4.898587196589412829E-16, 27.50000000000000000, 34.00000000000000000 ) ) ;
#10130=CARTESIAN_POINT ( 'NONE',  ( -4.000000000000000000, 16.26874999877096784, 30.00000000000000000 ) ) ;
#10157=CARTESIAN_POINT ( 'NONE',  ( -3.999999999999999112, 14.43124999877096570, 27.69059892324149530 ) ) ;
#10164=LINE ( 'NONE', #28248, #17674 ) ;
#10193=CARTESIAN_POINT ( 'NONE',  ( 1.138803498474273873E-14, 16.38124999877096499, 34.00000000000000000 ) ) ;
#10213=EDGE_CURVE ( 'NONE', #29842, #67424, #30314, .T. ) ;
#10225=EDGE_CURVE ( 'NONE', #29715, #8942, #37861, .T. ) ;
#10244=CARTESIAN_POINT ( 'NONE',  ( -3.756430356250001434, 14.70312499938548179, 32.16877607737301048 ) ) ;
#10250=( BOUNDED_CURVE ( )  B_SPLINE_CURVE ( 2, ( #26628, #9264, #27356, #4822, #59860, #44360, #43986, #31799, #21794 ),
 .UNSPECIFIED., .F., .F. ) 
 B_SPLINE_CURVE_WITH_KNOTS ( ( 3, 2, 2, 2, 3 ),
 ( 0.5972222222222222099, 0.6018518518518518601, 0.6111111111111111605, 0.6203703703703703498, 0.6250000000000000000 ),
 .UNSPECIFIED. ) 
 CURVE ( )  GEOMETRIC_REPRESENTATION_ITEM ( )  RATIONAL_B_SPLINE_CURVE ( ( 0.9330127018922194093, 0.9330127018922194093, 1.000000000000000000, 0.8660254037844387076, 1.000000000000000000, 0.8660254037844387076, 1.000000000000000000, 0.9330127018922194093, 0.9330127018922194093 ) ) 
 REPRESENTATION_ITEM ( '' )  );
#10254=CARTESIAN_POINT ( 'NONE',  ( 3.756430356250000546, 13.24062499938548321, 27.83122392262697886 ) ) ;
#10271=CARTESIAN_POINT ( 'NONE',  ( 5.810221930991193690E-16, 19.81250000000000000, 26.00000000000000000 ) ) ;
#10282=CARTESIAN_POINT ( 'NONE',  ( 3.756430356250000546, 15.37812499938548427, 27.83122392262697886 ) ) ;
#10284=CARTESIAN_POINT ( 'NONE',  ( 4.000000000000000000, 17.48750000000000071, 27.69059892324149530 ) ) ;
#10308=EDGE_CURVE ( 'NONE', #58357, #21163, #56222, .T. ) ;
#10333=ADVANCED_FACE ( 'NONE', ( #34656 ), #57185, .T. ) ;
#10360=CARTESIAN_POINT ( 'NONE',  ( 5.000000000000000000, 39.99999999999999289, 30.00000000000000000 ) ) ;
#10364=CARTESIAN_POINT ( 'NONE',  ( 1.878215178125000495, 15.07812499938548179, 26.74683588394047007 ) ) ;
#10407=CARTESIAN_POINT ( 'NONE',  ( 3.756430356250000546, 17.29062499938548214, 27.83122392262697886 ) ) ;
#10462=CARTESIAN_POINT ( 'NONE',  ( 3.756430356250000102, 15.79062499938548392, 30.00000000000000000 ) ) ;
#10468=CARTESIAN_POINT ( 'NONE',  ( 3.756430356249998770, 20.25312499938547717, 32.16877607737302469 ) ) ;
#10478=CARTESIAN_POINT ( 'NONE',  ( 3.756430356250000546, 18.52812499938548285, 27.83122392262697886 ) ) ;
#10482=ORIENTED_EDGE ( 'NONE', *, *, #458, .T. ) ;
#10495=CARTESIAN_POINT ( 'NONE',  ( -8.484601909799255319E-16, 15.48124999877096641, 34.61880215351700940 ) ) ;
#10498=CARTESIAN_POINT ( 'NONE',  ( -1.999999999999999112, 17.54374999877096641, 26.53589838486224650 ) ) ;
#10607=CARTESIAN_POINT ( 'NONE',  ( 3.756430356250000546, 14.47812499938548747, 27.83122392262697886 ) ) ;
#10615=CARTESIAN_POINT ( 'NONE',  ( 3.756430356250000102, 14.55312499938548321, 30.00000000000000000 ) ) ;
#10643=CARTESIAN_POINT ( 'NONE',  ( 3.756430356250000546, 14.02812499938548463, 27.83122392262697886 ) ) ;
#10645=CARTESIAN_POINT ( 'NONE',  ( -4.000000000000000000, 16.32499999999999929, 30.00000000000000000 ) ) ;
#10722=FACE_OUTER_BOUND ( 'NONE', #48151, .T. ) ;
#10727=CARTESIAN_POINT ( 'NONE',  ( -7.967954043666661671E-16, 14.89062499938548179, 34.33755215474603517 ) ) ;
#10769=CARTESIAN_POINT ( 'NONE',  ( -1.878215178124999163, 16.50312499938548427, 26.74683588394047007 ) ) ;
#10780=ORIENTED_EDGE ( 'NONE', *, *, #14213, .F. ) ;
#10790=CARTESIAN_POINT ( 'NONE',  ( -1.071796769724490339, 19.83259618943233704, 26.00000000000000000 ) ) ;
#10821=CARTESIAN_POINT ( 'NONE',  ( -3.756430356249999214, 14.17812499938548498, 27.83122392262697176 ) ) ;
#10836=CARTESIAN_POINT ( 'NONE',  ( -7.967954043666661671E-16, 19.27812499938548640, 34.33755215474603517 ) ) ;
#10846=CARTESIAN_POINT ( 'NONE',  ( -2.000000000000001776, 17.24374999877096570, 33.46410161513775705 ) ) ;
#10852=CARTESIAN_POINT ( 'NONE',  ( -8.484601909799255319E-16, 18.18124999877096215, 34.61880215351700940 ) ) ;
#10878=VECTOR ( 'NONE', #14421, 1000.000000000000000 ) ;
#10880=( BOUNDED_CURVE ( )  B_SPLINE_CURVE ( 2, ( #43956, #72023, #21400, #5518, #27325, #33938, #4069, #66478, #15856 ),
 .UNSPECIFIED., .F., .F. ) 
 B_SPLINE_CURVE_WITH_KNOTS ( ( 3, 2, 2, 2, 3 ),
 ( 0.01388888888888888985, 0.01851851851851851749, 0.02777777777777777624, 0.03703703703703703498, 0.04166666666666667129 ),
 .UNSPECIFIED. ) 
 CURVE ( )  GEOMETRIC_REPRESENTATION_ITEM ( )  RATIONAL_B_SPLINE_CURVE ( ( 0.9330127018922194093, 0.9330127018922194093, 1.000000000000000000, 0.8660254037844387076, 1.000000000000000000, 0.8660254037844387076, 1.000000000000000000, 0.9330127018922191873, 0.9330127018922192983 ) ) 
 REPRESENTATION_ITEM ( '' )  );
#10935=CIRCLE ( 'NONE', #61649, 14.99999999999999822 ) ;
#10941=SURFACE_SIDE_STYLE ('',( #62985 ) ) ;
#10977=CARTESIAN_POINT ( 'NONE',  ( -3.756430356250000990, 14.36562499938548321, 32.16877607737301048 ) ) ;
#10978=CARTESIAN_POINT ( 'NONE',  ( -4.000000000000000000, 14.01874999877096606, 30.00000000000000000 ) ) ;
#11006=CARTESIAN_POINT ( 'NONE',  ( 1.878215178124997609, 14.81562499938548427, 33.25316411605952993 ) ) ;
#11009=CARTESIAN_POINT ( 'NONE',  ( 2.828200636599751609E-16, 17.11250000000000071, 25.38119784648299415 ) ) ;
#11087=CARTESIAN_POINT ( 'NONE',  ( -3.756430356249999214, 15.19062499938548250, 27.83122392262697531 ) ) ;
#11097=CARTESIAN_POINT ( 'NONE',  ( 4.000000000000000000, 18.34999999999999787, 30.00000000000000000 ) ) ;
#11132=CARTESIAN_POINT ( 'NONE',  ( -3.756430356249999214, 16.99062499938548143, 27.83122392262697531 ) ) ;
#11148=ADVANCED_FACE ( 'NONE', ( #20804 ), #61430, .T. ) ;
#11158=CARTESIAN_POINT ( 'NONE',  ( 1.626862140677534470E-15, 13.68124999877096748, 34.00000000000000000 ) ) ;
#11187=CARTESIAN_POINT ( 'NONE',  ( 0.000000000000000000, 27.50000000000000000, 30.00000000000000000 ) ) ;
#11190=CARTESIAN_POINT ( 'NONE',  ( -3.756430356250000102, 14.66562499938548214, 30.00000000000000000 ) ) ;
#11206=CARTESIAN_POINT ( 'NONE',  ( -3.756430356250000102, 18.26562499938548356, 30.00000000000000000 ) ) ;
#11223=CARTESIAN_POINT ( 'NONE',  ( -2.000000000000001776, 17.69374999877096855, 33.46410161513775705 ) ) ;
#11258=CARTESIAN_POINT ( 'NONE',  ( -3.999999999999999112, 20.73124999877096641, 27.69059892324149530 ) ) ;
#11280=ORIENTED_EDGE ( 'NONE', *, *, #72942, .F. ) ;
#11347=CARTESIAN_POINT ( 'NONE',  ( -1.878215178125001827, 14.85312499938548214, 33.25316411605952283 ) ) ;
#11356=ORIENTED_EDGE ( 'NONE', *, *, #40217, .T. ) ;
#11370=VERTEX_POINT ( 'NONE', #32265 ) ;
#11375=CARTESIAN_POINT ( 'NONE',  ( 2.828200636599751609E-16, 18.46249999999999858, 25.38119784648299415 ) ) ;
#11420=CARTESIAN_POINT ( 'NONE',  ( 5.810221930991193690E-16, 20.20624999877096428, 26.00000000000000000 ) ) ;
#11455=CARTESIAN_POINT ( 'NONE',  ( -3.756430356250001434, 15.26562499938548356, 32.16877607737301048 ) ) ;
#11497=CARTESIAN_POINT ( 'NONE',  ( -3.756430356250000102, 17.02812499938548285, 30.00000000000000000 ) ) ;
#11535=CARTESIAN_POINT ( 'NONE',  ( -4.000000000000000000, 15.81874999877096499, 30.00000000000000000 ) ) ;
#11555=CARTESIAN_POINT ( 'NONE',  ( 3.756430356250000546, 16.72812499938548569, 27.83122392262697886 ) ) ;
#11587=CARTESIAN_POINT ( 'NONE',  ( 1.999999999999997335, 18.21874999877096712, 33.46410161513775705 ) ) ;
#11590=CARTESIAN_POINT ( 'NONE',  ( 5.810221930991193690E-16, 17.50624999877096499, 26.00000000000000000 ) ) ;
#11597=CARTESIAN_POINT ( 'NONE',  ( -2.672702088255949472E-15, 13.90624999877096890, 26.00000000000000000 ) ) ;
#11636=ADVANCED_FACE ( 'NONE', ( #45178 ), #41356, .T. ) ;
#11641=CARTESIAN_POINT ( 'NONE',  ( 1.071796769724491227, 19.34240381056766722, 26.00000000000000000 ) ) ;
#11705=CARTESIAN_POINT ( 'NONE',  ( 3.756430356249998770, 15.86562499938548321, 32.16877607737301759 ) ) ;
#11735=CARTESIAN_POINT ( 'NONE',  ( -8.484601909799255319E-16, 16.43750000000000000, 34.61880215351700940 ) ) ;
#11748=ORIENTED_EDGE ( 'NONE', *, *, #1852, .F. ) ;
#11780=( BOUNDED_CURVE ( )  B_SPLINE_CURVE ( 2, ( #42613, #37062, #13802, #59587, #8999, #31531, #30797, #54071, #24522 ),
 .UNSPECIFIED., .F., .F. ) 
 B_SPLINE_CURVE_WITH_KNOTS ( ( 3, 2, 2, 2, 3 ),
 ( 0.4583333333333333703, 0.4629629629629629650, 0.4722222222222222099, 0.4814814814814814548, 0.4861111111111111049 ),
 .UNSPECIFIED. ) 
 CURVE ( )  GEOMETRIC_REPRESENTATION_ITEM ( )  RATIONAL_B_SPLINE_CURVE ( ( 0.9330127018922194093, 0.9330127018922197424, 1.000000000000000000, 0.8660254037844387076, 1.000000000000000000, 0.8660254037844387076, 1.000000000000000000, 0.9330127018922194093, 0.9330127018922194093 ) ) 
 REPRESENTATION_ITEM ( '' )  );
#11800=CYLINDRICAL_SURFACE ( 'NONE', #12750, 4.000000000000000000 ) ;
#11812=CARTESIAN_POINT ( 'NONE',  ( 5.810221930991193690E-16, 18.01249999999999574, 26.00000000000000000 ) ) ;
#11817=CARTESIAN_POINT ( 'NONE',  ( 3.756430356250000102, 18.60312499938548214, 30.00000000000000000 ) ) ;
#11823=LINE ( 'NONE', #28097, #15998 ) ;
#11826=CARTESIAN_POINT ( 'NONE',  ( -4.000000000000000000, 16.32499999999999929, 30.00000000000000000 ) ) ;
#11853=ORIENTED_EDGE ( 'NONE', *, *, #19369, .F. ) ;
#11856=CARTESIAN_POINT ( 'NONE',  ( 1.878215178125000495, 18.22812499938548214, 26.74683588394047007 ) ) ;
#11870=DIRECTION ( 'NONE',  ( -0.000000000000000000, -1.000000000000000000, -0.000000000000000000 ) ) ;
#11881=CARTESIAN_POINT ( 'NONE',  ( 1.071796769724488785, 15.05134618820330061, 34.00000000000000000 ) ) ;
#11910=CARTESIAN_POINT ( 'NONE',  ( -3.756430356250000102, 16.01562499938548356, 30.00000000000000000 ) ) ;
#11941=CARTESIAN_POINT ( 'NONE',  ( 4.000000000000000000, 18.74374999877096570, 30.00000000000000000 ) ) ;
#11951=CARTESIAN_POINT ( 'NONE',  ( 3.999999999999998668, 16.06250000000000000, 32.30940107675850470 ) ) ;
#11966=DIRECTION ( 'NONE',  ( 0.000000000000000000, 0.000000000000000000, -1.000000000000000000 ) ) ;
#11969=CARTESIAN_POINT ( 'NONE',  ( 1.999999999999997335, 14.67500000000000071, 33.46410161513775705 ) ) ;
#12063=CARTESIAN_POINT ( 'NONE',  ( 1.878215178125000495, 15.52812499938548285, 26.74683588394047007 ) ) ;
#12077=EDGE_LOOP ( 'NONE', ( #60413, #20561, #29935, #57048, #69383, #13880, #29068, #39982 ) ) ;
#12095=CARTESIAN_POINT ( 'NONE',  ( 4.000000000000000000, 19.28750000000000142, 27.69059892324149530 ) ) ;
#12168=EDGE_CURVE ( 'NONE', #11370, #21163, #37624, .T. ) ;
#12172=CARTESIAN_POINT ( 'NONE',  ( 1.878215178125000495, 19.12812499938548427, 26.74683588394047007 ) ) ;
#12174=CARTESIAN_POINT ( 'NONE',  ( 4.849326327477522014, 20.72494550184886819, 32.95932117208439394 ) ) ;
#12211=CARTESIAN_POINT ( 'NONE',  ( -3.756430356250000102, 20.17812499938548143, 30.00000000000000000 ) ) ;
#12248=VERTEX_POINT ( 'NONE', #42081 ) ;
#12267=CARTESIAN_POINT ( 'NONE',  ( 3.756430356250000546, 17.17812499938548498, 27.83122392262697886 ) ) ;
#12290=AXIS2_PLACEMENT_3D ( 'NONE', #71861, #61491, #56324 ) ;
#12296=CARTESIAN_POINT ( 'NONE',  ( 2.828200636599751609E-16, 19.30624999877096570, 25.38119784648299415 ) ) ;
#12320=CARTESIAN_POINT ( 'NONE',  ( -2.000000000000001776, 14.54374999877096641, 33.46410161513775705 ) ) ;
#12342=EDGE_LOOP ( 'NONE', ( #67886, #54651, #60398, #22071 ) ) ;
#12351=CARTESIAN_POINT ( 'NONE',  ( -4.000000000000000000, 18.96874999877096357, 30.00000000000000000 ) ) ;
#12357=CARTESIAN_POINT ( 'NONE',  ( 3.756430356250000102, 13.99062499938548498, 30.00000000000000000 ) ) ;
#12380=PRESENTATION_STYLE_ASSIGNMENT (( #61906 ) ) ;
#12384=CARTESIAN_POINT ( 'NONE',  ( -3.486133158594716510E-16, 12.61250000000000426, 26.00000000000000355 ) ) ;
#12387=CARTESIAN_POINT ( 'NONE',  ( 2.393811435568372112E-14, 19.08124999877097139, 34.00000000000000000 ) ) ;
#12422=CARTESIAN_POINT ( 'NONE',  ( -3.756430356250000990, 17.51562499938548356, 32.16877607737301048 ) ) ;
#12457=CARTESIAN_POINT ( 'NONE',  ( 2.000000000000000444, 18.87500000000000000, 26.53589838486224650 ) ) ;
#12536=CARTESIAN_POINT ( 'NONE',  ( 3.756430356249998770, 18.56562499938548427, 32.16877607737302469 ) ) ;
#12538=CARTESIAN_POINT ( 'NONE',  ( 1.878215178124997609, 19.76562499938548356, 33.25316411605952993 ) ) ;
#12542=ADVANCED_FACE ( 'NONE', ( #58997 ), #13570, .T. ) ;
#12545=CARTESIAN_POINT ( 'NONE',  ( 0.000000000000000000, 27.50000000000000000, 26.00000000000000000 ) ) ;
#12597=AXIS2_PLACEMENT_3D ( 'NONE', #54500, #43423, #3901 ) ;
#12600=FACE_OUTER_BOUND ( 'NONE', #34654, .T. ) ;
#12630=CARTESIAN_POINT ( 'NONE',  ( 3.756430356249998770, 17.55312499938548498, 32.16877607737301759 ) ) ;
#12632=VERTEX_POINT ( 'NONE', #47938 ) ;
#12658=CARTESIAN_POINT ( 'NONE',  ( 3.756430356250000102, 13.65312499938548285, 30.00000000000000000 ) ) ;
#12683=CARTESIAN_POINT ( 'NONE',  ( -4.000000000000000888, 14.50624999877096499, 32.30940107675850470 ) ) ;
#12718=CARTESIAN_POINT ( 'NONE',  ( 3.756430356250000102, 18.49062499938548143, 30.00000000000000000 ) ) ;
#12743=CARTESIAN_POINT ( 'NONE',  ( -8.484601909799255319E-16, 13.23124999877096641, 34.61880215351700940 ) ) ;
#12750=AXIS2_PLACEMENT_3D ( 'NONE', #56498, #6627, #16601 ) ;
#12777=CARTESIAN_POINT ( 'NONE',  ( -1.878215178124999163, 16.95312499938548356, 26.74683588394047007 ) ) ;
#12811=CARTESIAN_POINT ( 'NONE',  ( 5.163760131380204399, 20.58432050246338108, 33.15120568351349561 ) ) ;
#12842=( BOUNDED_CURVE ( )  B_SPLINE_CURVE ( 2, ( #37620, #15811, #9913, #60142, #60880, #32815, #9186, #32451, #4747 ),
 .UNSPECIFIED., .F., .F. ) 
 B_SPLINE_CURVE_WITH_KNOTS ( ( 3, 2, 2, 2, 3 ),
 ( 0.5694444444444444198, 0.5740740740740740700, 0.5833333333333333703, 0.5925925925925925597, 0.5972222222222222099 ),
 .UNSPECIFIED. ) 
 CURVE ( )  GEOMETRIC_REPRESENTATION_ITEM ( )  RATIONAL_B_SPLINE_CURVE ( ( 0.9330127018922194093, 0.9330127018922194093, 1.000000000000000000, 0.8660254037844387076, 1.000000000000000000, 0.8660254037844387076, 1.000000000000000000, 0.9330127018922194093, 0.9330127018922194093 ) ) 
 REPRESENTATION_ITEM ( '' )  );
#12858=FACE_OUTER_BOUND ( 'NONE', #50572, .T. ) ;
#12859=( BOUNDED_CURVE ( )  B_SPLINE_CURVE ( 2, ( #51112, #49663, #44495, #67028, #50750, #67389, #22301, #33389, #17474 ),
 .UNSPECIFIED., .F., .F. ) 
 B_SPLINE_CURVE_WITH_KNOTS ( ( 3, 2, 2, 2, 3 ),
 ( 0.04166666666666667129, 0.04629629629629629373, 0.05555555555555555247, 0.06481481481481481122, 0.06944444444444444753 ),
 .UNSPECIFIED. ) 
 CURVE ( )  GEOMETRIC_REPRESENTATION_ITEM ( )  RATIONAL_B_SPLINE_CURVE ( ( 0.9330127018922192983, 0.9330127018922194093, 1.000000000000000000, 0.8660254037844387076, 1.000000000000000000, 0.8660254037844387076, 1.000000000000000000, 0.9330127018922191873, 0.9330127018922192983 ) ) 
 REPRESENTATION_ITEM ( '' )  );
#12871=EDGE_CURVE ( 'NONE', #49855, #12248, #55306, .T. ) ;
#12876=CARTESIAN_POINT ( 'NONE',  ( 0.5264921881209824184, 25.53585038844605037, 26.02618720140712227 ) ) ;
#12893=CARTESIAN_POINT ( 'NONE',  ( -3.756430356250001434, 19.31562499938548427, 32.16877607737301048 ) ) ;
#12895=CARTESIAN_POINT ( 'NONE',  ( 2.828200636599751609E-16, 12.61249999999999893, 25.38119784648299415 ) ) ;
#12973=EDGE_CURVE ( 'NONE', #28631, #32715, #47787, .T. ) ;
#12988=CARTESIAN_POINT ( 'NONE',  ( -3.756430356250000102, 17.81562499938548427, 30.00000000000000000 ) ) ;
#13015=CARTESIAN_POINT ( 'NONE',  ( 2.000000000000000444, 20.16874999877096641, 26.53589838486224650 ) ) ;
#13040=CARTESIAN_POINT ( 'NONE',  ( -1.071796769724489229, 14.56115380933863257, 34.00000000000000000 ) ) ;
#13041=CYLINDRICAL_SURFACE ( 'NONE', #70129, 4.000000000000000000 ) ;
#13048=CARTESIAN_POINT ( 'NONE',  ( 4.000000000000000000, 16.55000000000000071, 30.00000000000000000 ) ) ;
#13067=VERTEX_POINT ( 'NONE', #48302 ) ;
#13076=CARTESIAN_POINT ( 'NONE',  ( -3.756430356250001434, 16.95312499938548356, 32.16877607737301048 ) ) ;
#13095=CARTESIAN_POINT ( 'NONE',  ( 2.000000000000000444, 17.52499999999999858, 26.53589838486224650 ) ) ;
#13101=CARTESIAN_POINT ( 'NONE',  ( -2.000000000000001776, 14.54374999877096641, 33.46410161513775705 ) ) ;
#13121=VECTOR ( 'NONE', #7652, 1000.000000000000000 ) ;
#13133=CARTESIAN_POINT ( 'NONE',  ( -3.756430356249999214, 16.54062499938548569, 27.83122392262697176 ) ) ;
#13166=CARTESIAN_POINT ( 'NONE',  ( -4.000000000000000888, 19.51250000000000284, 32.30940107675850470 ) ) ;
#13170=CARTESIAN_POINT ( 'NONE',  ( -1.999999999999999112, 19.34374999877096712, 26.53589838486224650 ) ) ;
#13190=DIRECTION ( 'NONE',  ( -0.000000000000000000, -1.000000000000000000, -0.000000000000000000 ) ) ;
#13206=CARTESIAN_POINT ( 'NONE',  ( 1.138803498474273873E-14, 15.48124999877096641, 34.00000000000000000 ) ) ;
#13233=CARTESIAN_POINT ( 'NONE',  ( 3.177768106359410094, 25.19871980768746411, 27.55645491167268091 ) ) ;
#13248=CARTESIAN_POINT ( 'NONE',  ( -3.756430356250000102, 17.47812499938548214, 30.00000000000000000 ) ) ;
#13250=CARTESIAN_POINT ( 'NONE',  ( 4.000000000000000000, 12.50000000000000000, 30.00000000000000000 ) ) ;
#13260=( BOUNDED_CURVE ( )  B_SPLINE_CURVE ( 2, ( #34344, #17357, #6281, #62789, #11826, #28811, #752, #67622, #45811 ),
 .UNSPECIFIED., .F., .F. ) 
 B_SPLINE_CURVE_WITH_KNOTS ( ( 3, 2, 2, 2, 3 ),
 ( 0.4583333333333333703, 0.4629629629629629650, 0.4722222222222222099, 0.4814814814814814548, 0.4861111111111111049 ),
 .UNSPECIFIED. ) 
 CURVE ( )  GEOMETRIC_REPRESENTATION_ITEM ( )  RATIONAL_B_SPLINE_CURVE ( ( 0.9330127018922194093, 0.9330127018922197424, 1.000000000000000000, 0.8660254037844387076, 1.000000000000000000, 0.8660254037844387076, 1.000000000000000000, 0.9330127018922194093, 0.9330127018922194093 ) ) 
 REPRESENTATION_ITEM ( '' )  );
#13288=CARTESIAN_POINT ( 'NONE',  ( 3.756430356250000546, 19.54062499938548214, 27.83122392262697886 ) ) ;
#13326=CARTESIAN_POINT ( 'NONE',  ( -3.468515707051626151, 25.13356901665284937, 32.00919774098884574 ) ) ;
#13343=CARTESIAN_POINT ( 'NONE',  ( 1.878215178125000495, 19.46562499938548640, 26.74683588394047007 ) ) ;
#13370=CARTESIAN_POINT ( 'NONE',  ( 3.999999999999998668, 20.05624999877096570, 32.30940107675850470 ) ) ;
#13378=CARTESIAN_POINT ( 'NONE',  ( 1.071796769724479237, 18.89240381056766793, 25.99999999999999645 ) ) ;
#13414=ORIENTED_EDGE ( 'NONE', *, *, #19199, .F. ) ;
#13429=CARTESIAN_POINT ( 'NONE',  ( 2.655984681222220721E-16, 16.35312499938548214, 25.66244784525396483 ) ) ;
#13454=CARTESIAN_POINT ( 'NONE',  ( -8.484601909799255319E-16, 14.13124999877096855, 34.61880215351700940 ) ) ;
#13457=CARTESIAN_POINT ( 'NONE',  ( 4.000000000000000000, 19.19374999877096499, 30.00000000000000000 ) ) ;
#13465=( BOUNDED_CURVE ( )  B_SPLINE_CURVE ( 2, ( #67418, #49694, #55594, #11258, #22687, #56323, #67771, #72584, #17146 ),
 .UNSPECIFIED., .F., .F. ) 
 B_SPLINE_CURVE_WITH_KNOTS ( ( 3, 2, 2, 2, 3 ),
 ( 0.9583333333333333703, 0.9629629629629629095, 0.9722222222222222099, 0.9814814814814815103, 0.9861111111111111605 ),
 .UNSPECIFIED. ) 
 CURVE ( )  GEOMETRIC_REPRESENTATION_ITEM ( )  RATIONAL_B_SPLINE_CURVE ( ( 0.9330127018922192983, 0.9330127018922200755, 1.000000000000000000, 0.8660254037844387076, 1.000000000000000000, 0.8660254037844387076, 1.000000000000000000, 0.9330127018922185211, 0.9330127018922194093 ) ) 
 REPRESENTATION_ITEM ( '' )  );
#13490=CARTESIAN_POINT ( 'NONE',  ( 1.878215178125000495, 15.97812499938548392, 26.74683588394047007 ) ) ;
#13528=CARTESIAN_POINT ( 'NONE',  ( 2.828200636599751609E-16, 19.81250000000000000, 25.38119784648299415 ) ) ;
#13546=CARTESIAN_POINT ( 'NONE',  ( 1.071796769724491227, 19.73615380933863150, 26.00000000000000000 ) ) ;
#13559=AXIS2_PLACEMENT_3D ( 'NONE', #22878, #67255, #5549 ) ;
#13570=CYLINDRICAL_SURFACE ( 'NONE', #43301, 4.000000000000000000 ) ;
#13596=CARTESIAN_POINT ( 'NONE',  ( 1.774929369453897232, 25.43659371523960644, 33.59414506192486982 ) ) ;
#13605=CARTESIAN_POINT ( 'NONE',  ( 0.000000000000000000, 27.50000000000000000, 30.00000000000000000 ) ) ;
#13613=CARTESIAN_POINT ( 'NONE',  ( 3.756430356250000102, 12.64062499938548356, 30.00000000000000000 ) ) ;
#13615=CARTESIAN_POINT ( 'NONE',  ( 2.655984681222220721E-16, 19.95312499938548356, 25.66244784525396483 ) ) ;
#13684=CARTESIAN_POINT ( 'NONE',  ( 1.071796769724488785, 20.45134618820329919, 34.00000000000000000 ) ) ;
#13697=CARTESIAN_POINT ( 'NONE',  ( -3.179381680195804805, 25.19837022949101168, 27.55859303876839306 ) ) ;
#13714=CARTESIAN_POINT ( 'NONE',  ( -0.6941602726958887581, 20.61426555956768780, 33.93677853444431491 ) ) ;
#13747=CARTESIAN_POINT ( 'NONE',  ( -7.967954043666661671E-16, 13.09062499938548285, 34.33755215474603517 ) ) ;
#13783=VERTEX_POINT ( 'NONE', #69173 ) ;
#13802=CARTESIAN_POINT ( 'NONE',  ( -1.999999999999999112, 16.64374999877096784, 26.53589838486224650 ) ) ;
#13804=CARTESIAN_POINT ( 'NONE',  ( -3.999999999999999112, 14.03750000000000142, 27.69059892324149530 ) ) ;
#13810=CARTESIAN_POINT ( 'NONE',  ( -1.878215178124999163, 16.39062499938548356, 26.74683588394047007 ) ) ;
#13819=CARTESIAN_POINT ( 'NONE',  ( 1.878215178125000495, 15.86562499938548321, 26.74683588394047007 ) ) ;
#13833=CARTESIAN_POINT ( 'NONE',  ( -3.999999999999999556, 14.88124999877096499, 27.69059892324149175 ) ) ;
#13863=EDGE_CURVE ( 'NONE', #62113, #25000, #29459, .T. ) ;
#13867=CARTESIAN_POINT ( 'NONE',  ( -3.756430356250000102, 19.72812499938548214, 30.00000000000000000 ) ) ;
#13880=ORIENTED_EDGE ( 'NONE', *, *, #71305, .T. ) ;
#13892=CARTESIAN_POINT ( 'NONE',  ( 3.999999999999998668, 14.20624999877096606, 32.30940107675850470 ) ) ;
#13907=CARTESIAN_POINT ( 'NONE',  ( -1.071796769724492115, 19.51115380933863008, 34.00000000000000000 ) ) ;
#13939=ORIENTED_EDGE ( 'NONE', *, *, #5583, .T. ) ;
#13966=CARTESIAN_POINT ( 'NONE',  ( 3.795044958738071461, 25.05366892013418934, 31.29105878821236786 ) ) ;
#13982=CARTESIAN_POINT ( 'NONE',  ( -3.756430356250001434, 12.90312499938548463, 32.16877607737301048 ) ) ;
#13984=CARTESIAN_POINT ( 'NONE',  ( 1.999999999999997335, 14.22499999999999964, 33.46410161513775705 ) ) ;
#14061=CARTESIAN_POINT ( 'NONE',  ( 0.000000000000000000, 25.54316770519903557, 26.00000000000000000 ) ) ;
#14064=CARTESIAN_POINT ( 'NONE',  ( 3.756430356249998770, 13.16562499938548392, 32.16877607737302469 ) ) ;
#14106=CARTESIAN_POINT ( 'NONE',  ( 3.756430356250000546, 13.24062499938548321, 27.83122392262697886 ) ) ;
#14120=EDGE_LOOP ( 'NONE', ( #29700, #57009, #23078, #30077 ) ) ;
#14135=CARTESIAN_POINT ( 'NONE',  ( 4.000000000000000000, 20.15000000000000213, 30.00000000000000000 ) ) ;
#14149=ORIENTED_EDGE ( 'NONE', *, *, #37745, .T. ) ;
#14156=CARTESIAN_POINT ( 'NONE',  ( -1.626862140677534273E-15, 19.98124999877096641, 34.00000000000000000 ) ) ;
#14166=CARTESIAN_POINT ( 'NONE',  ( 3.756430356250000102, 13.09062499938548463, 30.00000000000000000 ) ) ;
#14173=CARTESIAN_POINT ( 'NONE',  ( -3.756430356250000102, 16.91562499938548214, 30.00000000000000000 ) ) ;
#14182=CARTESIAN_POINT ( 'NONE',  ( -7.967954043666661671E-16, 15.22812499938548214, 34.33755215474603517 ) ) ;
#14197=CARTESIAN_POINT ( 'NONE',  ( 3.999999999999998668, 14.65624999877096535, 32.30940107675850470 ) ) ;
#14213=EDGE_CURVE ( 'NONE', #38333, #12248, #70458, .T. ) ;
#14223=CARTESIAN_POINT ( 'NONE',  ( -2.498395430326213790E-14, 18.46250000000000213, 26.00000000000000000 ) ) ;
#14230=CARTESIAN_POINT ( 'NONE',  ( -3.756430356249999214, 20.14062499938548356, 27.83122392262697176 ) ) ;
#14280=PRODUCT ( 'pressure gauge', 'pressure gauge', '', ( #60715 ) ) ;
#14332=MECHANICAL_DESIGN_GEOMETRIC_PRESENTATION_REPRESENTATION('',(#46204),#65071);
#14352=CARTESIAN_POINT ( 'NONE',  ( -1.878215178124999163, 13.69062499938548427, 26.74683588394047007 ) ) ;
#14354=CARTESIAN_POINT ( 'NONE',  ( -8.484601909799255319E-16, 14.18750000000000000, 34.61880215351700940 ) ) ;
#14421=DIRECTION ( 'NONE',  ( -0.000000000000000000, -1.000000000000000000, -0.000000000000000000 ) ) ;
#14434=CARTESIAN_POINT ( 'NONE',  ( -7.967954043666661671E-16, 14.44062499938548427, 34.33755215474603517 ) ) ;
#14446=CARTESIAN_POINT ( 'NONE',  ( 1.878215178125000495, 19.91562499938548569, 26.74683588394047007 ) ) ;
#14477=CARTESIAN_POINT ( 'NONE',  ( 1.878215178124997609, 14.92812499938548321, 33.25316411605952993 ) ) ;
#14518=CARTESIAN_POINT ( 'NONE',  ( 4.898587196589412829E-16, 27.50000000000000000, 34.00000000000000000 ) ) ;
#14531=CARTESIAN_POINT ( 'NONE',  ( -3.756430356250000102, 13.31562499938548427, 30.00000000000000000 ) ) ;
#14537=CARTESIAN_POINT ( 'NONE',  ( -1.878215178125001827, 20.14062499938548356, 33.25316411605952283 ) ) ;
#14546=CARTESIAN_POINT ( 'NONE',  ( -1.878215178124999163, 15.49062499938548321, 26.74683588394047007 ) ) ;
#14563=CARTESIAN_POINT ( 'NONE',  ( -4.000000000000000888, 16.30624999877096570, 32.30940107675850470 ) ) ;
#14593=CARTESIAN_POINT ( 'NONE',  ( -1.878215178124999163, 20.10312499938548569, 26.74683588394047007 ) ) ;
#14653=CARTESIAN_POINT ( 'NONE',  ( 0.000000000000000000, 27.50000000000000000, 30.00000000000000000 ) ) ;
#14686=FACE_OUTER_BOUND ( 'NONE', #12077, .T. ) ;
#14703=CARTESIAN_POINT ( 'NONE',  ( 4.898587196589412829E-16, 27.50000000000000000, 34.00000000000000000 ) ) ;
#14707=EDGE_CURVE ( 'NONE', #59214, #23775, #29110, .T. ) ;
#14713=CARTESIAN_POINT ( 'NONE',  ( 1.878215178125000495, 20.02812499938548285, 26.74683588394047007 ) ) ;
#14715=CARTESIAN_POINT ( 'NONE',  ( 4.000000000000000000, 15.19999999999999929, 30.00000000000000000 ) ) ;
#14768=CARTESIAN_POINT ( 'NONE',  ( 4.898587196589412829E-16, 27.50000000000000000, 34.00000000000000000 ) ) ;
#14798=CARTESIAN_POINT ( 'NONE',  ( -3.756430356250001434, 13.91562499938548392, 32.16877607737301048 ) ) ;
#14807=CARTESIAN_POINT ( 'NONE',  ( -1.243387493232115393E-14, 16.60624999877096641, 26.00000000000000000 ) ) ;
#14809=CARTESIAN_POINT ( 'NONE',  ( 3.756430356249998770, 18.45312499938548356, 32.16877607737301759 ) ) ;
#14843=CARTESIAN_POINT ( 'NONE',  ( -1.878215178125001827, 16.20312499938548356, 33.25316411605952283 ) ) ;
#14869=CARTESIAN_POINT ( 'NONE',  ( 1.071796769724488785, 15.95134618820330097, 34.00000000000000000 ) ) ;
#14898=CARTESIAN_POINT ( 'NONE',  ( 1.878215178124997609, 13.46562499938548285, 33.25316411605952993 ) ) ;
#14905=CARTESIAN_POINT ( 'NONE',  ( -1.878215178124999163, 19.99062499938548143, 26.74683588394047007 ) ) ;
#14914=CARTESIAN_POINT ( 'NONE',  ( -3.756430356250000102, 16.91562499938548214, 30.00000000000000000 ) ) ;
#14924=AXIS2_PLACEMENT_3D ( 'NONE', #17751, #11870, #34391 ) ;
#14930=CARTESIAN_POINT ( 'NONE',  ( -4.000000000000000888, 15.85624999877096641, 32.30940107675850470 ) ) ;
#14963=CARTESIAN_POINT ( 'NONE',  ( 3.756430356249998770, 18.56562499938548427, 32.16877607737301759 ) ) ;
#14973=CARTESIAN_POINT ( 'NONE',  ( -2.000000000000001776, 20.44999999999999929, 33.46410161513775705 ) ) ;
#15044=CARTESIAN_POINT ( 'NONE',  ( 1.878215178125000495, 14.06562499938548250, 26.74683588394047007 ) ) ;
#15051=CARTESIAN_POINT ( 'NONE',  ( -4.000000000000000000, 18.51874999877096784, 30.00000000000000000 ) ) ;
#15054=CARTESIAN_POINT ( 'NONE',  ( 3.756430356250000102, 13.20312499938548356, 30.00000000000000000 ) ) ;
#15080=CARTESIAN_POINT ( 'NONE',  ( -3.756430356249999214, 20.59062499938548640, 27.83122392262697531 ) ) ;
#15082=CARTESIAN_POINT ( 'NONE',  ( -1.999999999999999112, 15.80000000000000071, 26.53589838486224650 ) ) ;
#15094=LINE ( 'NONE', #8829, #30116 ) ;
#15101=CARTESIAN_POINT ( 'NONE',  ( -4.000000000000000000, 15.42500000000000071, 30.00000000000000000 ) ) ;
#15153=CARTESIAN_POINT ( 'NONE',  ( 0.000000000000000000, 27.50000000000000000, 30.00000000000000000 ) ) ;
#15162=CARTESIAN_POINT ( 'NONE',  ( 2.655984681222220721E-16, 13.31562499938548783, 25.66244784525396483 ) ) ;
#15205=CARTESIAN_POINT ( 'NONE',  ( -7.967954043666661671E-16, 13.99062499938548498, 34.33755215474603517 ) ) ;
#15251=CARTESIAN_POINT ( 'NONE',  ( 5.810221930991193690E-16, 19.75624999877096499, 26.00000000000000000 ) ) ;
#15268=CARTESIAN_POINT ( 'NONE',  ( 3.756430356249998770, 18.90312499938548640, 32.16877607737302469 ) ) ;
#15277=CARTESIAN_POINT ( 'NONE',  ( 2.655984681222220721E-16, 17.25312499938548072, 25.66244784525396483 ) ) ;
#15292=CARTESIAN_POINT ( 'NONE',  ( -1.999999999999999112, 15.29374999877096641, 26.53589838486224650 ) ) ;
#15321=CARTESIAN_POINT ( 'NONE',  ( -1.999999999999999112, 12.65000000000000213, 26.53589838486224650 ) ) ;
#15324=CARTESIAN_POINT ( 'NONE',  ( -7.967954043666661671E-16, 19.84062499938548285, 34.33755215474603517 ) ) ;
#15378=CARTESIAN_POINT ( 'NONE',  ( -2.498395430326213790E-14, 18.91249999999999787, 26.00000000000000000 ) ) ;
#15405=CARTESIAN_POINT ( 'NONE',  ( -3.756430356249999214, 14.62812499938548250, 27.83122392262697531 ) ) ;
#15411=CARTESIAN_POINT ( 'NONE',  ( -3.999999999999999112, 18.48124999877096641, 27.69059892324149530 ) ) ;
#15434=ORIENTED_EDGE ( 'NONE', *, *, #35065, .F. ) ;
#15438=CARTESIAN_POINT ( 'NONE',  ( 2.655984681222220721E-16, 15.00312499938548427, 25.66244784525396483 ) ) ;
#15440=CARTESIAN_POINT ( 'NONE',  ( -4.000000000000000888, 15.01250000000000107, 32.30940107675850470 ) ) ;
#15453=ORIENTED_EDGE ( 'NONE', *, *, #48200, .F. ) ;
#15468=EDGE_CURVE ( 'NONE', #3561, #45011, #23695, .T. ) ;
#15488=PRODUCT_DEFINITION_SHAPE ( 'NONE', 'NONE',  #3433 ) ;
#15515=DIRECTION ( 'NONE',  ( -0.000000000000000000, -1.000000000000000000, -0.000000000000000000 ) ) ;
#15524=CARTESIAN_POINT ( 'NONE',  ( -7.967954043666661671E-16, 13.54062499938548214, 34.33755215474603517 ) ) ;
#15567=CARTESIAN_POINT ( 'NONE',  ( 3.756430356250000102, 14.55312499938548321, 30.00000000000000000 ) ) ;
#15590=CARTESIAN_POINT ( 'NONE',  ( -3.999999999999999112, 13.53124999877096535, 27.69059892324149530 ) ) ;
#15607=( BOUNDED_CURVE ( )  B_SPLINE_CURVE ( 2, ( #15251, #65499, #49254, #20791, #3460, #43710, #4555, #49616, #14156 ),
 .UNSPECIFIED., .F., .F. ) 
 B_SPLINE_CURVE_WITH_KNOTS ( ( 3, 2, 2, 2, 3 ),
 ( 0.8472222222222222099, 0.8518518518518518601, 0.8611111111111111605, 0.8703703703703703498, 0.8750000000000000000 ),
 .UNSPECIFIED. ) 
 CURVE ( )  GEOMETRIC_REPRESENTATION_ITEM ( )  RATIONAL_B_SPLINE_CURVE ( ( 0.9330127018922194093, 0.9330127018922194093, 1.000000000000000000, 0.8660254037844387076, 1.000000000000000000, 0.8660254037844387076, 1.000000000000000000, 0.9330127018922194093, 0.9330127018922194093 ) ) 
 REPRESENTATION_ITEM ( '' )  );
#15621=CARTESIAN_POINT ( 'NONE',  ( 2.655984681222220721E-16, 15.00312499938548605, 25.66244784525396483 ) ) ;
#15627=CARTESIAN_POINT ( 'NONE',  ( -1.878215178125001827, 19.69062499938548072, 33.25316411605952283 ) ) ;
#15637=CARTESIAN_POINT ( 'NONE',  ( -1.878215178125001827, 18.34062499938548285, 33.25316411605952283 ) ) ;
#15654=CARTESIAN_POINT ( 'NONE',  ( 4.000000000000000000, 16.04374999877096641, 30.00000000000000000 ) ) ;
#15681=CARTESIAN_POINT ( 'NONE',  ( 5.810221930991193690E-16, 14.35624999877096464, 26.00000000000000000 ) ) ;
#15689=DIRECTION ( 'NONE',  ( 0.000000000000000000, 0.000000000000000000, -1.000000000000000000 ) ) ;
#15717=ORIENTED_EDGE ( 'NONE', *, *, #19271, .T. ) ;
#15723=CARTESIAN_POINT ( 'NONE',  ( 1.071796769724491227, 17.48615380933863506, 26.00000000000000000 ) ) ;
#15741=CARTESIAN_POINT ( 'NONE',  ( -3.999999999999999112, 18.98749999999999716, 27.69059892324149530 ) ) ;
#15770=CARTESIAN_POINT ( 'NONE',  ( 3.756430356250000546, 13.57812499938548711, 27.83122392262697886 ) ) ;
#15776=CARTESIAN_POINT ( 'NONE',  ( -4.000000000000000888, 18.55624999877096570, 32.30940107675850470 ) ) ;
#15779=CARTESIAN_POINT ( 'NONE',  ( -1.878215178125001827, 13.05312499938548321, 33.25316411605952283 ) ) ;
#15780=CARTESIAN_POINT ( 'NONE',  ( -1.626862140677534273E-15, 20.03749999999999787, 34.00000000000000000 ) ) ;
#15808=CARTESIAN_POINT ( 'NONE',  ( 1.878215178124997609, 15.71562499938548108, 33.25316411605952993 ) ) ;
#15810=CARTESIAN_POINT ( 'NONE',  ( 2.000000000000000444, 17.07499999999999929, 26.53589838486224650 ) ) ;
#15811=CARTESIAN_POINT ( 'NONE',  ( -1.071796769724490339, 17.13259618943233420, 26.00000000000000000 ) ) ;
#15856=CARTESIAN_POINT ( 'NONE',  ( 1.626862140677534470E-15, 13.23124999877096819, 34.00000000000000000 ) ) ;
#15874=DIRECTION ( 'NONE',  ( 0.000000000000000000, 0.000000000000000000, -1.000000000000000000 ) ) ;
#15888=DIRECTION ( 'NONE',  ( 0.000000000000000000, 0.000000000000000000, -1.000000000000000000 ) ) ;
#15893=CARTESIAN_POINT ( 'NONE',  ( -1.878215178124999163, 16.95312499938548356, 26.74683588394047007 ) ) ;
#15935=CARTESIAN_POINT ( 'NONE',  ( -1.878215178125001827, 15.30312499938548321, 33.25316411605952283 ) ) ;
#15973=VERTEX_POINT ( 'NONE', #629 ) ;
#15986=AXIS2_PLACEMENT_3D ( 'NONE', #14653, #42745, #21295 ) ;
#15992=CARTESIAN_POINT ( 'NONE',  ( -1.878215178125001827, 14.74062499938548321, 33.25316411605952283 ) ) ;
#15994=CARTESIAN_POINT ( 'NONE',  ( 0.000000000000000000, 27.50000000000000000, 30.00000000000000000 ) ) ;
#15998=VECTOR ( 'NONE', #33266, 1000.000000000000000 ) ;
#15999=CARTESIAN_POINT ( 'NONE',  ( 3.756430356249998770, 19.80312499938548498, 32.16877607737302469 ) ) ;
#16008=CARTESIAN_POINT ( 'NONE',  ( 3.756430356249998770, 18.00312499938548427, 32.16877607737302469 ) ) ;
#16025=CARTESIAN_POINT ( 'NONE',  ( 3.999999999999998668, 15.10624999877096641, 32.30940107675850470 ) ) ;
#16029=ORIENTED_EDGE ( 'NONE', *, *, #27236, .T. ) ;
#16077=ORIENTED_EDGE ( 'NONE', *, *, #19175, .T. ) ;
#16126=ORIENTED_EDGE ( 'NONE', *, *, #32305, .T. ) ;
#16141=CARTESIAN_POINT ( 'NONE',  ( 1.878215178124997609, 14.36562499938548321, 33.25316411605952993 ) ) ;
#16149=CARTESIAN_POINT ( 'NONE',  ( -3.756430356250000990, 13.91562499938548392, 32.16877607737301048 ) ) ;
#16150=LINE ( 'NONE', #68228, #3165 ) ;
#16156=EDGE_CURVE ( 'NONE', #38031, #17018, #32692, .T. ) ;
#16168=CARTESIAN_POINT ( 'NONE',  ( 1.071796769724491227, 19.79240381056766651, 26.00000000000000000 ) ) ;
#16178=CARTESIAN_POINT ( 'NONE',  ( -3.756430356250000102, 14.66562499938548214, 30.00000000000000000 ) ) ;
#16180=CARTESIAN_POINT ( 'NONE',  ( -8.484601909799255319E-16, 17.33749999999999858, 34.61880215351700940 ) ) ;
#16220=EDGE_CURVE ( 'NONE', #35360, #27263, #62468, .T. ) ;
#16259=CARTESIAN_POINT ( 'NONE',  ( -3.756430356250001434, 17.06562499938548427, 32.16877607737301048 ) ) ;
#16289=ORIENTED_EDGE ( 'NONE', *, *, #67586, .F. ) ;
#16293=( BOUNDED_CURVE ( )  B_SPLINE_CURVE ( 2, ( #21342, #50528, #9901, #27632, #66797, #38340, #5459, #16168, #10271 ),
 .UNSPECIFIED., .F., .F. ) 
 B_SPLINE_CURVE_WITH_KNOTS ( ( 3, 2, 2, 2, 3 ),
 ( 0.8750000000000000000, 0.8796296296296296502, 0.8888888888888888395, 0.8981481481481481399, 0.9027777777777777901 ),
 .UNSPECIFIED. ) 
 CURVE ( )  GEOMETRIC_REPRESENTATION_ITEM ( )  RATIONAL_B_SPLINE_CURVE ( ( 0.9330127018922194093, 0.9330127018922194093, 1.000000000000000000, 0.8660254037844387076, 1.000000000000000000, 0.8660254037844387076, 1.000000000000000000, 0.9330127018922194093, 0.9330127018922194093 ) ) 
 REPRESENTATION_ITEM ( '' )  );
#16303=CARTESIAN_POINT ( 'NONE',  ( 1.878215178125000495, 18.67812499938548143, 26.74683588394047007 ) ) ;
#16325=CARTESIAN_POINT ( 'NONE',  ( -4.000000000000000888, 13.60624999877096641, 32.30940107675850470 ) ) ;
#16345=ORIENTED_EDGE ( 'NONE', *, *, #3608, .F. ) ;
#16354=CARTESIAN_POINT ( 'NONE',  ( -3.756430356250000102, 14.21562499938548285, 30.00000000000000000 ) ) ;
#16369=CARTESIAN_POINT ( 'NONE',  ( -7.967954043666661671E-16, 18.82812499938548356, 34.33755215474603517 ) ) ;
#16385=CARTESIAN_POINT ( 'NONE',  ( 4.000000000000000000, 19.23124999877096641, 27.69059892324149530 ) ) ;
#16451=CARTESIAN_POINT ( 'NONE',  ( 0.6522972858965978560, 20.64114861271052348, 33.69936173848522998 ) ) ;
#16497=CARTESIAN_POINT ( 'NONE',  ( 2.655984681222220721E-16, 13.65312499938548463, 25.66244784525396483 ) ) ;
#16507=CARTESIAN_POINT ( 'NONE',  ( -1.878215178124999163, 15.15312499938548285, 26.74683588394047007 ) ) ;
#16508=CARTESIAN_POINT ( 'NONE',  ( 4.648177544792955741E-15, 14.13124999877096322, 33.99999999999999289 ) ) ;
#16531=ORIENTED_EDGE ( 'NONE', *, *, #49494, .F. ) ;
#16535=CARTESIAN_POINT ( 'NONE',  ( 1.878215178125000495, 14.51562499938548356, 26.74683588394047007 ) ) ;
#16538=CARTESIAN_POINT ( 'NONE',  ( -4.000000000000000888, 18.16249999999999787, 32.30940107675850470 ) ) ;
#16558=CARTESIAN_POINT ( 'NONE',  ( 1.071796769724488785, 20.00134618820329635, 34.00000000000000000 ) ) ;
#16601=DIRECTION ( 'NONE',  ( 0.000000000000000000, 0.000000000000000000, -1.000000000000000000 ) ) ;
#16608=CARTESIAN_POINT ( 'NONE',  ( 1.626862140677534470E-15, 12.83750000000000213, 34.00000000000000000 ) ) ;
#16617=CARTESIAN_POINT ( 'NONE',  ( 3.756430356250000102, 15.45312499938548356, 30.00000000000000000 ) ) ;
#16661=CARTESIAN_POINT ( 'NONE',  ( 3.756430356250000102, 17.25312499938548072, 30.00000000000000000 ) ) ;
#16672=VERTEX_POINT ( 'NONE', #16777 ) ;
#16707=PRODUCT_DEFINITION_FORMATION_WITH_SPECIFIED_SOURCE ( 'ANY', '', #14280, .NOT_KNOWN. ) ;
#16708=ORIENTED_EDGE ( 'NONE', *, *, #12168, .F. ) ;
#16719=CARTESIAN_POINT ( 'NONE',  ( 2.655984681222220721E-16, 15.90312499938548108, 25.66244784525396483 ) ) ;
#16734=CARTESIAN_POINT ( 'NONE',  ( -3.756430356250001434, 19.65312499938548640, 32.16877607737301048 ) ) ;
#16748=CARTESIAN_POINT ( 'NONE',  ( 3.999999999999998668, 18.25624999877096499, 32.30940107675850470 ) ) ;
#16759=DIRECTION ( 'NONE',  ( -0.000000000000000000, -1.000000000000000000, -0.000000000000000000 ) ) ;
#16769=AXIS2_PLACEMENT_3D ( 'NONE', #17122, #16759, #68469 ) ;
#16777=CARTESIAN_POINT ( 'NONE',  ( -1.243387493232115393E-14, 14.86250000000000071, 26.00000000000000000 ) ) ;
#16867=CARTESIAN_POINT ( 'NONE',  ( -3.756430356250000102, 15.67812499938548143, 30.00000000000000000 ) ) ;
#16868=CARTESIAN_POINT ( 'NONE',  ( -2.000000000000001776, 15.44374999877096677, 33.46410161513775705 ) ) ;
#16877=VERTEX_POINT ( 'NONE', #40414 ) ;
#16897=CARTESIAN_POINT ( 'NONE',  ( 1.999999999999997335, 18.27499999999999858, 33.46410161513775705 ) ) ;
#16916=CARTESIAN_POINT ( 'NONE',  ( 3.999999999999998668, 20.05624999877096570, 32.30940107675850470 ) ) ;
#16934=DIRECTION ( 'NONE',  ( -0.000000000000000000, -1.000000000000000000, -0.000000000000000000 ) ) ;
#16979=CARTESIAN_POINT ( 'NONE',  ( -1.878215178125001827, 17.10312499938548214, 33.25316411605952283 ) ) ;
#17018=VERTEX_POINT ( 'NONE', #1260 ) ;
#17021=CARTESIAN_POINT ( 'NONE',  ( -1.878215178125001827, 16.65312499938548285, 33.25316411605952283 ) ) ;
#17031=ORIENTED_EDGE ( 'NONE', *, *, #65041, .T. ) ;
#17034=VECTOR ( 'NONE', #26597, 1000.000000000000000 ) ;
#17069=ORIENTED_EDGE ( 'NONE', *, *, #5701, .T. ) ;
#17079=CARTESIAN_POINT ( 'NONE',  ( 1.878215178125000495, 14.06562499938548250, 26.74683588394047007 ) ) ;
#17096=CARTESIAN_POINT ( 'NONE',  ( 2.655984681222220721E-16, 17.70312499938548356, 25.66244784525396483 ) ) ;
#17110=PLANE ( 'NONE',  #38671 ) ;
#17112=CARTESIAN_POINT ( 'NONE',  ( 4.000000000000000000, 18.78124999877096357, 27.69059892324149530 ) ) ;
#17122=CARTESIAN_POINT ( 'NONE',  ( 0.000000000000000000, 27.50000000000000000, 30.00000000000000000 ) ) ;
#17139=DIRECTION ( 'NONE',  ( -1.000000000000000000, -0.000000000000000000, -0.000000000000000000 ) ) ;
#17146=CARTESIAN_POINT ( 'NONE',  ( 2.411242101361345515E-14, 20.88124999877096499, 34.00000000000000000 ) ) ;
#17155=CARTESIAN_POINT ( 'NONE',  ( -5.000000000000000000, 39.99999999999999289, 30.00000000000000000 ) ) ;
#17201=CARTESIAN_POINT ( 'NONE',  ( 1.071796769724490783, 12.59240381056766722, 26.00000000000000000 ) ) ;
#17232=CARTESIAN_POINT ( 'NONE',  ( 3.756430356250000546, 15.49062499938548321, 27.83122392262697886 ) ) ;
#17263=CARTESIAN_POINT ( 'NONE',  ( -4.000000000000000888, 18.61250000000000426, 32.30940107675850470 ) ) ;
#17275=CARTESIAN_POINT ( 'NONE',  ( 3.999999999999998668, 13.75624999877096677, 32.30940107675850470 ) ) ;
#17306=( BOUNDED_CURVE ( )  B_SPLINE_CURVE ( 2, ( #20770, #42950, #65478, #20029, #14135, #33232, #2697, #60287, #36311 ),
 .UNSPECIFIED., .F., .F. ) 
 B_SPLINE_CURVE_WITH_KNOTS ( ( 3, 2, 2, 2, 3 ),
 ( 0.9305555555555555802, 0.9351851851851852304, 0.9444444444444444198, 0.9537037037037037202, 0.9583333333333333703 ),
 .UNSPECIFIED. ) 
 CURVE ( )  GEOMETRIC_REPRESENTATION_ITEM ( )  RATIONAL_B_SPLINE_CURVE ( ( 0.9330127018922194093, 0.9330127018922194093, 1.000000000000000000, 0.8660254037844387076, 1.000000000000000000, 0.8660254037844387076, 1.000000000000000000, 0.9330127018922185211, 0.9330127018922192983 ) ) 
 REPRESENTATION_ITEM ( '' )  );
#17317=ADVANCED_FACE ( 'NONE', ( #6636 ), #68694, .T. ) ;
#17322=CARTESIAN_POINT ( 'NONE',  ( -1.626862140677534273E-15, 17.78749999999999787, 34.00000000000000000 ) ) ;
#17346=CARTESIAN_POINT ( 'NONE',  ( -3.756430356250000102, 15.22812499938548392, 30.00000000000000000 ) ) ;
#17357=CARTESIAN_POINT ( 'NONE',  ( -1.071796769724496334, 16.23259618943233562, 26.00000000000000355 ) ) ;
#17387=CARTESIAN_POINT ( 'NONE',  ( 1.878215178125000495, 17.77812499938548285, 26.74683588394047007 ) ) ;
#17439=DIRECTION ( 'NONE',  ( -0.000000000000000000, -1.000000000000000000, -0.000000000000000000 ) ) ;
#17441=CARTESIAN_POINT ( 'NONE',  ( 1.878215178124997609, 16.61562499938548143, 33.25316411605952993 ) ) ;
#17460=ORIENTED_EDGE ( 'NONE', *, *, #60559, .F. ) ;
#17471=CARTESIAN_POINT ( 'NONE',  ( 4.000000000000000000, 18.33124999877096784, 27.69059892324149530 ) ) ;
#17474=CARTESIAN_POINT ( 'NONE',  ( -2.672702088255949472E-15, 13.06250000000000355, 26.00000000000000000 ) ) ;
#17496=CARTESIAN_POINT ( 'NONE',  ( -2.498395430326213790E-14, 20.65624999877097068, 26.00000000000000000 ) ) ;
#17498=CYLINDRICAL_SURFACE ( 'NONE', #3331, 4.000000000000000000 ) ;
#17523=ORIENTED_EDGE ( 'NONE', *, *, #5583, .F. ) ;
#17561=ORIENTED_EDGE ( 'NONE', *, *, #65041, .F. ) ;
#17590=CARTESIAN_POINT ( 'NONE',  ( -3.756430356250000990, 15.26562499938548356, 32.16877607737301048 ) ) ;
#17591=CARTESIAN_POINT ( 'NONE',  ( -2.000000000000001776, 14.09374999877096535, 33.46410161513775705 ) ) ;
#17620=CARTESIAN_POINT ( 'NONE',  ( -2.000000000000001776, 18.64999999999999858, 33.46410161513775705 ) ) ;
#17632=CARTESIAN_POINT ( 'NONE',  ( 1.071796769724490561, 13.70134618820330097, 34.00000000000000000 ) ) ;
#17661=CARTESIAN_POINT ( 'NONE',  ( -4.000000000000000000, 20.31874999877096499, 30.00000000000000000 ) ) ;
#17674=VECTOR ( 'NONE', #51140, 1000.000000000000000 ) ;
#17698=CARTESIAN_POINT ( 'NONE',  ( -3.756430356250001434, 18.86562499938548498, 32.16877607737301048 ) ) ;
#17700=CARTESIAN_POINT ( 'NONE',  ( -2.000000000000001776, 12.80000000000000071, 33.46410161513775705 ) ) ;
#17706=ADVANCED_FACE ( 'NONE', ( #59396 ), #42792, .T. ) ;
#17735=ORIENTED_EDGE ( 'NONE', *, *, #49537, .F. ) ;
#17738=CARTESIAN_POINT ( 'NONE',  ( -1.878215178125001827, 18.90312499938548285, 33.25316411605952283 ) ) ;
#17751=CARTESIAN_POINT ( 'NONE',  ( 0.000000000000000000, 27.50000000000000000, 30.00000000000000000 ) ) ;
#17761=CARTESIAN_POINT ( 'NONE',  ( 3.999999999999998668, 15.10624999877096641, 32.30940107675850470 ) ) ;
#17792=CARTESIAN_POINT ( 'NONE',  ( -3.756430356249999214, 16.87812499938548427, 27.83122392262697176 ) ) ;
#17821=CARTESIAN_POINT ( 'NONE',  ( -2.000000000000001776, 19.49374999877096570, 33.46410161513775705 ) ) ;
#17831=CARTESIAN_POINT ( 'NONE',  ( 4.000000000000000000, 16.10000000000000142, 30.00000000000000000 ) ) ;
#17867=EDGE_CURVE ( 'NONE', #57346, #55447, #50856, .T. ) ;
#17885=CARTESIAN_POINT ( 'NONE',  ( 3.756430356249998770, 15.30312499938548498, 32.16877607737302469 ) ) ;
#17914=CARTESIAN_POINT ( 'NONE',  ( 2.000000000000000444, 19.26874999877096784, 26.53589838486224650 ) ) ;
#17942=EDGE_CURVE ( 'NONE', #68198, #58357, #60495, .T. ) ;
#17946=CARTESIAN_POINT ( 'NONE',  ( 3.756430356250000102, 18.15312499938548285, 30.00000000000000000 ) ) ;
#17971=CARTESIAN_POINT ( 'NONE',  ( -1.626862140677534273E-15, 16.83124999877096428, 34.00000000000000000 ) ) ;
#17975=( BOUNDED_SURFACE ( )  B_SPLINE_SURFACE ( 1, 2, ( 
 ( #59491, #25520, #38066, #19596, #4106, #59124, #48797, #25894, #36603, #43259, #21073, #14064, #3735, #71326, #20701, #15162, #26633, #66146, #42152, #65408, #49170, #15524, #65044, #37699, #60221, #8531, #53598, #60590, #2624, #9999, #2992, #14798, #8904, #9634, #37341, #70590, #19965, #42518, #47686, #31435, #54341, #48434, #43624, #32168, #9268, #14434, #36969, #53227, #53975, #70959, #20332, #59864, #31803, #26260, #70222, #27001, #374, #10727, #45440, #27725, #43991, #38439, #10364, #56515, #67259, #11087, #17346, #11455, #32895, #49531, #4827, #62418, #16617, #5908, #61329, #5553, #5187, #72055, #33259, #66891, #44364, #55797, #62061, #28442, #21799, #21434, #28091, #67973, #39905, #32534, #33615, #72788, #61688, #24, #39172, #60965, #50263, #55070, #27361, #55435, #56159, #50619, #22530, #45077, #50977, #66512, #22882, #38814, #22171, #49892, #44724, #67613, #15893, #4471, #72417, #16259, #16979, #39536, #33976, #18783, #52065, #46161, #63858, #2188, #24702, #56868, #13248, #57950, #35070, #40259, #29887, #68338, #1832, #57596, #6272, #41348, #28800, #68701, #51705, #62780, #51341, #18061, #46523, #41700, #19146, #57229, #40622, #29530, #63141, #34700, #6644, #1108, #29171, #743, #35786, #12536, #11817, #34334, #45802, #23615, #69779, #23252, #18424, #17698, #6999, #1469, #52426, #58309, #23975, #69065, #12172, #40990, #63506, #7358, #47246, #12893, #35426, #24340, #46888, #69426, #7720, #30254, #52787, #8814, #20986, #59041, #64595, #20248, #65322, #42800, #70874, #60139, #25064, #54613, #14713, #30981, #30616, #65693, #70137, #59777, #36887, #47607, #54254, #32082, #19515, #37255, #9183, #31718, #3650, #15080, #4019, #53146, #3283, #37617, #26544 ),
 ( #13613, #71613, #42073, #25811, #19886, #26173, #48349, #13982, #36521, #2545, #36158, #70510, #48714, #59406, #9548, #71236, #20616, #8445, #58676, #8086, #53514, #2908, #25439, #42439, #47982, #53892, #43174, #49085, #14352, #64961, #64224, #31351, #27278, #43539, #23441, #49811, #12357, #10643, #4389, #38350, #34891, #60877, #33173, #933, #33527, #45987, #72336, #61605, #40445, #49443, #16535, #71977, #72703, #66060, #16178, #28996, #9910, #21350, #11006, #56077, #55711, #66806, #62961, #15438, #68524, #54983, #38729, #39088, #5105, #26918, #37982, #17885, #21716, #10282, #32812, #57420, #43907, #60504, #44275, #5468, #27639, #66430, #15808, #32448, #55350, #61249, #44644, #50175, #6824, #51533, #22086, #4744, #67174, #29358, #51891, #1289, #29713, #52613, #18612, #13429, #13810, #41890, #47074, #63686, #8637, #35615, #7541, #23799, #2735, #30075, #64782, #64049, #57775, #41177, #14173, #13076, #35979, #53337, #36350, #25252, #2019, #64417, #19706, #52251, #69964, #1654, #52974, #46350, #69609, #8274, #63330, #24163, #58864, #30804, #58498, #18970, #42259, #68884, #47801, #35254, #41530, #19335, #7907, #7185, #18241, #70330, #24530, #58135, #30445, #36707, #46715, #40814, #2370, #59229, #31166, #53708, #12718, #69250, #24888, #47433, #25630, #65887, #38169, #60693, #37446, #48536, #54443, #15268, #21173, #49271, #3478, #65519, #55176, #9736, #21540, #4209, #42987, #42623, #4572, #9009, #71804, #48902, #59597, #66249, #44095, #37073, #26737, #43726, #15627, #10106, #27102, #15999, #65147, #37806, #49634, #38548, #14905, #32636, #72161, #31541, #14537, #61071, #48167, #10468, #54081, #60326, #66622, #31906, #32998, #43364, #59966, #3101, #70692, #20067, #25997 ) ),
 .UNSPECIFIED., .F., .F., .F. ) 
 B_SPLINE_SURFACE_WITH_KNOTS ( ( 2, 2 ),
 ( 3, 2, 2, 2, 2, 2, 2, 2, 2, 2, 2, 2, 2, 2, 2, 2, 2, 2, 2, 2, 2, 2, 2, 2, 2, 2, 2, 2, 2, 2, 2, 2, 2, 2, 2, 2, 2, 2, 2, 2, 2, 2, 2, 2, 2, 2, 2, 2, 2, 2, 2, 2, 2, 2, 2, 2, 2, 2, 2, 2, 2, 2, 2, 2, 2, 2, 2, 2, 2, 2, 2, 2, 2, 2, 2, 2, 2, 2, 2, 2, 2, 2, 2, 2, 2, 2, 2, 2, 2, 2, 2, 2, 2, 2, 2, 2, 2, 2, 2, 2, 2, 2, 2, 2, 2, 2, 2, 3 ),
 ( 0.000000000000000000, 1.000000000000000000 ),
 ( 0.000000000000000000, 0.009259259259259258745, 0.01851851851851851749, 0.02777777777777777624, 0.03703703703703703498, 0.04629629629629629373, 0.05555555555555555247, 0.06481481481481481122, 0.07407407407407406996, 0.08333333333333332871, 0.09259259259259258745, 0.1018518518518518462, 0.1111111111111111049, 0.1203703703703703637, 0.1296296296296296224, 0.1388888888888888951, 0.1481481481481481399, 0.1574074074074074125, 0.1666666666666666574, 0.1759259259259259300, 0.1851851851851851749, 0.1944444444444444475, 0.2037037037037036924, 0.2129629629629629650, 0.2222222222222222099, 0.2314814814814814825, 0.2407407407407407274, 0.2500000000000000000, 0.2592592592592592449, 0.2685185185185185452, 0.2777777777777777901, 0.2870370370370370350, 0.2962962962962962798, 0.3055555555555555802, 0.3148148148148148251, 0.3240740740740740700, 0.3333333333333333148, 0.3425925925925926152, 0.3518518518518518601, 0.3611111111111111049, 0.3703703703703703498, 0.3796296296296296502, 0.3888888888888888951, 0.3981481481481481399, 0.4074074074074073848, 0.4166666666666666852, 0.4259259259259259300, 0.4351851851851851749, 0.4444444444444444198, 0.4537037037037037202, 0.4629629629629629650, 0.4722222222222222099, 0.4814814814814814548, 0.4907407407407407551, 0.5000000000000000000, 0.5092592592592593004, 0.5185185185185184897, 0.5277777777777777901, 0.5370370370370370905, 0.5462962962962962798, 0.5555555555555555802, 0.5648148148148147696, 0.5740740740740740700, 0.5833333333333333703, 0.5925925925925925597, 0.6018518518518518601, 0.6111111111111111605, 0.6203703703703703498, 0.6296296296296296502, 0.6388888888888888395, 0.6481481481481481399, 0.6574074074074074403, 0.6666666666666666297, 0.6759259259259259300, 0.6851851851851852304, 0.6944444444444444198, 0.7037037037037037202, 0.7129629629629629095, 0.7222222222222222099, 0.7314814814814815103, 0.7407407407407406996, 0.7500000000000000000, 0.7592592592592593004, 0.7685185185185184897, 0.7777777777777777901, 0.7870370370370370905, 0.7962962962962962798, 0.8055555555555555802, 0.8148148148148147696, 0.8240740740740740700, 0.8333333333333333703, 0.8425925925925925597, 0.8518518518518518601, 0.8611111111111111605, 0.8703703703703703498, 0.8796296296296296502, 0.8888888888888888395, 0.8981481481481481399, 0.9074074074074074403, 0.9166666666666666297, 0.9259259259259259300, 0.9351851851851852304, 0.9444444444444444198, 0.9537037037037037202, 0.9629629629629629095, 0.9722222222222222099, 0.9814814814814815103, 0.9876227413766924812 ),
 .UNSPECIFIED. ) 
 GEOMETRIC_REPRESENTATION_ITEM ( )  RATIONAL_B_SPLINE_SURFACE ( (
 ( 1.000000000000000000, 0.8660254037844387076, 1.000000000000000000, 0.8660254037844387076, 1.000000000000000000, 0.8660254037844387076, 1.000000000000000000, 0.8660254037844387076, 1.000000000000000000, 0.8660254037844387076, 1.000000000000000000, 0.8660254037844387076, 1.000000000000000000, 0.8660254037844387076, 1.000000000000000000, 0.8660254037844387076, 1.000000000000000000, 0.8660254037844387076, 1.000000000000000000, 0.8660254037844387076, 1.000000000000000000, 0.8660254037844387076, 1.000000000000000000, 0.8660254037844387076, 1.000000000000000000, 0.8660254037844387076, 1.000000000000000000, 0.8660254037844387076, 1.000000000000000000, 0.8660254037844387076, 1.000000000000000000, 0.8660254037844387076, 1.000000000000000000, 0.8660254037844387076, 1.000000000000000000, 0.8660254037844387076, 1.000000000000000000, 0.8660254037844387076, 1.000000000000000000, 0.8660254037844387076, 1.000000000000000000, 0.8660254037844387076, 1.000000000000000000, 0.8660254037844387076, 1.000000000000000000, 0.8660254037844387076, 1.000000000000000000, 0.8660254037844387076, 1.000000000000000000, 0.8660254037844387076, 1.000000000000000000, 0.8660254037844387076, 1.000000000000000000, 0.8660254037844387076, 1.000000000000000000, 0.8660254037844387076, 1.000000000000000000, 0.8660254037844387076, 1.000000000000000000, 0.8660254037844387076, 1.000000000000000000, 0.8660254037844387076, 1.000000000000000000, 0.8660254037844387076, 1.000000000000000000, 0.8660254037844387076, 1.000000000000000000, 0.8660254037844387076, 1.000000000000000000, 0.8660254037844387076, 1.000000000000000000, 0.8660254037844387076, 1.000000000000000000, 0.8660254037844387076, 1.000000000000000000, 0.8660254037844387076, 1.000000000000000000, 0.8660254037844387076, 1.000000000000000000, 0.8660254037844387076, 1.000000000000000000, 0.8660254037844387076, 1.000000000000000000, 0.8660254037844387076, 1.000000000000000000, 0.8660254037844387076, 1.000000000000000000, 0.8660254037844387076, 1.000000000000000000, 0.8660254037844387076, 1.000000000000000000, 0.8660254037844387076, 1.000000000000000000, 0.8660254037844387076, 1.000000000000000000, 0.8660254037844387076, 1.000000000000000000, 0.8660254037844387076, 1.000000000000000000, 0.8660254037844387076, 1.000000000000000000, 0.8660254037844387076, 1.000000000000000000, 0.8660254037844387076, 1.000000000000000000, 0.8660254037844387076, 1.000000000000000000, 0.8660254037844387076, 1.000000000000000000, 0.8660254037844387076, 1.000000000000000000, 0.8660254037844387076, 1.000000000000000000, 0.8660254037844387076, 1.000000000000000000, 0.8660254037844387076, 1.000000000000000000, 0.8660254037844387076, 1.000000000000000000, 0.8660254037844387076, 1.000000000000000000, 0.8660254037844387076, 1.000000000000000000, 0.8660254037844387076, 1.000000000000000000, 0.8660254037844387076, 1.000000000000000000, 0.8660254037844387076, 1.000000000000000000, 0.8660254037844387076, 1.000000000000000000, 0.8660254037844387076, 1.000000000000000000, 0.8660254037844387076, 1.000000000000000000, 0.8660254037844387076, 1.000000000000000000, 0.8660254037844387076, 1.000000000000000000, 0.8660254037844387076, 1.000000000000000000, 0.8660254037844387076, 1.000000000000000000, 0.8660254037844387076, 1.000000000000000000, 0.8660254037844387076, 1.000000000000000000, 0.8660254037844387076, 1.000000000000000000, 0.8660254037844387076, 1.000000000000000000, 0.8660254037844387076, 1.000000000000000000, 0.8660254037844387076, 1.000000000000000000, 0.8660254037844387076, 1.000000000000000000, 0.8660254037844387076, 1.000000000000000000, 0.8660254037844387076, 1.000000000000000000, 0.8660254037844387076, 1.000000000000000000, 0.8660254037844387076, 1.000000000000000000, 0.8660254037844387076, 1.000000000000000000, 0.8660254037844387076, 1.000000000000000000, 0.8660254037844387076, 1.000000000000000000, 0.8660254037844387076, 1.000000000000000000, 0.8660254037844387076, 1.000000000000000000, 0.8660254037844387076, 1.000000000000000000, 0.8660254037844387076, 1.000000000000000000, 0.8660254037844387076, 1.000000000000000000, 0.8660254037844387076, 1.000000000000000000, 0.8660254037844387076, 1.000000000000000000, 0.8660254037844387076, 1.000000000000000000, 0.8660254037844387076, 1.000000000000000000, 0.8660254037844387076, 1.000000000000000000, 0.8660254037844387076, 1.000000000000000000, 0.8660254037844387076, 1.000000000000000000, 0.8660254037844387076, 1.000000000000000000, 0.8660254037844387076, 1.000000000000000000, 0.8660254037844387076, 1.000000000000000000, 0.8660254037844387076, 1.000000000000000000, 0.8660254037844387076, 1.000000000000000000, 0.8660254037844387076, 1.000000000000000000, 0.8660254037844387076, 1.000000000000000000, 0.8660254037844387076, 1.000000000000000000, 0.8660254037844387076, 1.000000000000000000, 0.9111405360107026619, 0.9401542295230078672),
 ( 1.000000000000000000, 0.8660254037844387076, 1.000000000000000000, 0.8660254037844387076, 1.000000000000000000, 0.8660254037844387076, 1.000000000000000000, 0.8660254037844387076, 1.000000000000000000, 0.8660254037844387076, 1.000000000000000000, 0.8660254037844387076, 1.000000000000000000, 0.8660254037844387076, 1.000000000000000000, 0.8660254037844387076, 1.000000000000000000, 0.8660254037844387076, 1.000000000000000000, 0.8660254037844387076, 1.000000000000000000, 0.8660254037844387076, 1.000000000000000000, 0.8660254037844387076, 1.000000000000000000, 0.8660254037844387076, 1.000000000000000000, 0.8660254037844387076, 1.000000000000000000, 0.8660254037844387076, 1.000000000000000000, 0.8660254037844387076, 1.000000000000000000, 0.8660254037844387076, 1.000000000000000000, 0.8660254037844387076, 1.000000000000000000, 0.8660254037844387076, 1.000000000000000000, 0.8660254037844387076, 1.000000000000000000, 0.8660254037844387076, 1.000000000000000000, 0.8660254037844387076, 1.000000000000000000, 0.8660254037844387076, 1.000000000000000000, 0.8660254037844387076, 1.000000000000000000, 0.8660254037844387076, 1.000000000000000000, 0.8660254037844387076, 1.000000000000000000, 0.8660254037844387076, 1.000000000000000000, 0.8660254037844387076, 1.000000000000000000, 0.8660254037844387076, 1.000000000000000000, 0.8660254037844387076, 1.000000000000000000, 0.8660254037844387076, 1.000000000000000000, 0.8660254037844387076, 1.000000000000000000, 0.8660254037844387076, 1.000000000000000000, 0.8660254037844387076, 1.000000000000000000, 0.8660254037844387076, 1.000000000000000000, 0.8660254037844387076, 1.000000000000000000, 0.8660254037844387076, 1.000000000000000000, 0.8660254037844387076, 1.000000000000000000, 0.8660254037844387076, 1.000000000000000000, 0.8660254037844387076, 1.000000000000000000, 0.8660254037844387076, 1.000000000000000000, 0.8660254037844387076, 1.000000000000000000, 0.8660254037844387076, 1.000000000000000000, 0.8660254037844387076, 1.000000000000000000, 0.8660254037844387076, 1.000000000000000000, 0.8660254037844387076, 1.000000000000000000, 0.8660254037844387076, 1.000000000000000000, 0.8660254037844387076, 1.000000000000000000, 0.8660254037844387076, 1.000000000000000000, 0.8660254037844387076, 1.000000000000000000, 0.8660254037844387076, 1.000000000000000000, 0.8660254037844387076, 1.000000000000000000, 0.8660254037844387076, 1.000000000000000000, 0.8660254037844387076, 1.000000000000000000, 0.8660254037844387076, 1.000000000000000000, 0.8660254037844387076, 1.000000000000000000, 0.8660254037844387076, 1.000000000000000000, 0.8660254037844387076, 1.000000000000000000, 0.8660254037844387076, 1.000000000000000000, 0.8660254037844387076, 1.000000000000000000, 0.8660254037844387076, 1.000000000000000000, 0.8660254037844387076, 1.000000000000000000, 0.8660254037844387076, 1.000000000000000000, 0.8660254037844387076, 1.000000000000000000, 0.8660254037844387076, 1.000000000000000000, 0.8660254037844387076, 1.000000000000000000, 0.8660254037844387076, 1.000000000000000000, 0.8660254037844387076, 1.000000000000000000, 0.8660254037844387076, 1.000000000000000000, 0.8660254037844387076, 1.000000000000000000, 0.8660254037844387076, 1.000000000000000000, 0.8660254037844387076, 1.000000000000000000, 0.8660254037844387076, 1.000000000000000000, 0.8660254037844387076, 1.000000000000000000, 0.8660254037844387076, 1.000000000000000000, 0.8660254037844387076, 1.000000000000000000, 0.8660254037844387076, 1.000000000000000000, 0.8660254037844387076, 1.000000000000000000, 0.8660254037844387076, 1.000000000000000000, 0.8660254037844387076, 1.000000000000000000, 0.8660254037844387076, 1.000000000000000000, 0.8660254037844387076, 1.000000000000000000, 0.8660254037844387076, 1.000000000000000000, 0.8660254037844387076, 1.000000000000000000, 0.8660254037844387076, 1.000000000000000000, 0.8660254037844387076, 1.000000000000000000, 0.8660254037844387076, 1.000000000000000000, 0.8660254037844387076, 1.000000000000000000, 0.8660254037844387076, 1.000000000000000000, 0.8660254037844387076, 1.000000000000000000, 0.8660254037844387076, 1.000000000000000000, 0.8660254037844387076, 1.000000000000000000, 0.8660254037844387076, 1.000000000000000000, 0.8660254037844387076, 1.000000000000000000, 0.8660254037844387076, 1.000000000000000000, 0.8660254037844387076, 1.000000000000000000, 0.8660254037844387076, 1.000000000000000000, 0.8660254037844387076, 1.000000000000000000, 0.8660254037844387076, 1.000000000000000000, 0.8660254037844387076, 1.000000000000000000, 0.8660254037844387076, 1.000000000000000000, 0.8660254037844387076, 1.000000000000000000, 0.8660254037844387076, 1.000000000000000000, 0.8660254037844387076, 1.000000000000000000, 0.8660254037844387076, 1.000000000000000000, 0.8660254037844387076, 1.000000000000000000, 0.9111405360107026619, 0.9401542295230078672) ) ) 
 REPRESENTATION_ITEM ( '' )  SURFACE ( )  );
#17980=CARTESIAN_POINT ( 'NONE',  ( -3.999999999999999556, 18.98749999999999716, 27.69059892324149175 ) ) ;
#18010=( BOUNDED_CURVE ( )  B_SPLINE_CURVE ( 2, ( #2825, #53804, #54533, #3935, #29539, #3567, #43457, #26458, #48264 ),
 .UNSPECIFIED., .F., .F. ) 
 B_SPLINE_CURVE_WITH_KNOTS ( ( 3, 2, 2, 2, 3 ),
 ( 0.8472222222222222099, 0.8518518518518518601, 0.8611111111111111605, 0.8703703703703703498, 0.8750000000000000000 ),
 .UNSPECIFIED. ) 
 CURVE ( )  GEOMETRIC_REPRESENTATION_ITEM ( )  RATIONAL_B_SPLINE_CURVE ( ( 0.9330127018922194093, 0.9330127018922194093, 1.000000000000000000, 0.8660254037844387076, 1.000000000000000000, 0.8660254037844387076, 1.000000000000000000, 0.9330127018922194093, 0.9330127018922194093 ) ) 
 REPRESENTATION_ITEM ( '' )  );
#18030=CARTESIAN_POINT ( 'NONE',  ( 1.999999999999997335, 17.82499999999999929, 33.46410161513775705 ) ) ;
#18061=CARTESIAN_POINT ( 'NONE',  ( -7.967954043666661671E-16, 18.04062499938548214, 34.33755215474603517 ) ) ;
#18063=CARTESIAN_POINT ( 'NONE',  ( 3.756430356250000102, 20.29062499938548569, 30.00000000000000000 ) ) ;
#18094=CARTESIAN_POINT ( 'NONE',  ( 5.810221930991193690E-16, 19.36250000000000071, 26.00000000000000000 ) ) ;
#18098=CARTESIAN_POINT ( 'NONE',  ( 3.756430356250000546, 20.44062499938547717, 27.83122392262697886 ) ) ;
#18114=EDGE_CURVE ( 'NONE', #71973, #41056, #16293, .T. ) ;
#18123=CARTESIAN_POINT ( 'NONE',  ( 1.071796769724485232, 15.23615380933862973, 25.99999999999999645 ) ) ;
#18152=CARTESIAN_POINT ( 'NONE',  ( -3.756430356249999214, 15.97812499938548392, 27.83122392262697176 ) ) ;
#18182=CARTESIAN_POINT ( 'NONE',  ( 4.000000000000000000, 20.54374999877096641, 30.00000000000000000 ) ) ;
#18236=CARTESIAN_POINT ( 'NONE',  ( 0.6945846161026939525, 20.50052346155192140, 33.93923243933046763 ) ) ;
#18241=CARTESIAN_POINT ( 'NONE',  ( 3.756430356250000102, 18.04062499938548214, 30.00000000000000000 ) ) ;
#18268=CARTESIAN_POINT ( 'NONE',  ( -4.000000000000000000, 13.56874999877096677, 30.00000000000000000 ) ) ;
#18271=ORIENTED_EDGE ( 'NONE', *, *, #54489, .F. ) ;
#18292=VECTOR ( 'NONE', #54507, 1000.000000000000000 ) ;
#18304=CARTESIAN_POINT ( 'NONE',  ( -3.756430356250000102, 16.12812499938548427, 30.00000000000000000 ) ) ;
#18338=CARTESIAN_POINT ( 'NONE',  ( 2.000000000000000444, 19.77500000000000213, 26.53589838486224650 ) ) ;
#18356=AXIS2_PLACEMENT_3D ( 'NONE', #61775, #51425, #38898 ) ;
#18424=CARTESIAN_POINT ( 'NONE',  ( -3.756430356250000102, 18.82812499938548356, 30.00000000000000000 ) ) ;
#18426=CARTESIAN_POINT ( 'NONE',  ( -2.000000000000001776, 13.25000000000000178, 33.46410161513775705 ) ) ;
#18463=VERTEX_POINT ( 'NONE', #40528 ) ;
#18466=CARTESIAN_POINT ( 'NONE',  ( -1.878215178124999163, 18.75312499938548427, 26.74683588394047007 ) ) ;
#18493=CARTESIAN_POINT ( 'NONE',  ( -2.498395430326213790E-14, 20.65624999877097068, 26.00000000000000000 ) ) ;
#18504=CARTESIAN_POINT ( 'NONE',  ( -3.999999999999999112, 15.78124999877096535, 27.69059892324149530 ) ) ;
#18521=CARTESIAN_POINT ( 'NONE',  ( 3.756430356249998770, 16.65312499938548285, 32.16877607737301759 ) ) ;
#18550=CARTESIAN_POINT ( 'NONE',  ( -3.999999999999999556, 20.73124999877096641, 27.69059892324149175 ) ) ;
#18562=VERTEX_POINT ( 'NONE', #40233 ) ;
#18574=CARTESIAN_POINT ( 'NONE',  ( -3.999999999999999112, 13.13749999999999751, 27.69059892324149530 ) ) ;
#18606=CARTESIAN_POINT ( 'NONE',  ( 2.417052323292336544E-14, 20.48749999999999716, 34.00000000000000000 ) ) ;
#18612=CARTESIAN_POINT ( 'NONE',  ( 1.878215178125000495, 16.31562499938548427, 26.74683588394047007 ) ) ;
#18637=CARTESIAN_POINT ( 'NONE',  ( 1.999999999999997335, 14.61874999877096570, 33.46410161513775705 ) ) ;
#18656=CARTESIAN_POINT ( 'NONE',  ( 3.878215178125000051, 12.57031249969274178, 30.00000000000000000 ) ) ;
#18670=CARTESIAN_POINT ( 'NONE',  ( -3.756430356250000102, 17.02812499938548285, 30.00000000000000000 ) ) ;
#18740=CARTESIAN_POINT ( 'NONE',  ( 1.071796769724488785, 18.20134618820329919, 34.00000000000000000 ) ) ;
#18751=FACE_OUTER_BOUND ( 'NONE', #6654, .T. ) ;
#18783=CARTESIAN_POINT ( 'NONE',  ( 3.756430356249998770, 17.21562499938548285, 32.16877607737302469 ) ) ;
#18785=CARTESIAN_POINT ( 'NONE',  ( 3.756430356249998770, 19.80312499938548498, 32.16877607737302469 ) ) ;
#18823=CARTESIAN_POINT ( 'NONE',  ( 3.756430356250000102, 20.40312499938548285, 30.00000000000000000 ) ) ;
#18878=CARTESIAN_POINT ( 'NONE',  ( 1.878215178125000495, 16.76562499938548356, 26.74683588394047007 ) ) ;
#18908=CARTESIAN_POINT ( 'NONE',  ( -8.484601909799255319E-16, 20.43124999877096570, 34.61880215351700940 ) ) ;
#18932=CARTESIAN_POINT ( 'NONE',  ( 1.626862140677534470E-15, 13.28750000000000142, 34.00000000000000000 ) ) ;
#18970=CARTESIAN_POINT ( 'NONE',  ( 2.655984681222220721E-16, 17.70312499938548356, 25.66244784525396483 ) ) ;
#18987=CARTESIAN_POINT ( 'NONE',  ( -1.626862140677534273E-15, 17.33749999999999858, 34.00000000000000000 ) ) ;
#18993=DIRECTION ( 'NONE',  ( -0.000000000000000000, -1.000000000000000000, -0.000000000000000000 ) ) ;
#19024=ADVANCED_FACE ( 'NONE', ( #20957 ), #66035, .T. ) ;
#19029=CARTESIAN_POINT ( 'NONE',  ( 1.878215178124997609, 16.72812499938548214, 33.25316411605952993 ) ) ;
#19058=EDGE_LOOP ( 'NONE', ( #49261, #47435 ) ) ;
#19064=CARTESIAN_POINT ( 'NONE',  ( 1.999999999999997335, 18.72499999999999787, 33.46410161513775705 ) ) ;
#19084=CARTESIAN_POINT ( 'NONE',  ( 4.000000000000000000, 19.64374999877096428, 30.00000000000000000 ) ) ;
#19130=CARTESIAN_POINT ( 'NONE',  ( 1.626862140677534470E-15, 13.28750000000000142, 34.00000000000000000 ) ) ;
#19146=CARTESIAN_POINT ( 'NONE',  ( 3.756430356250000102, 18.15312499938548285, 30.00000000000000000 ) ) ;
#19148=CARTESIAN_POINT ( 'NONE',  ( -1.878215178124999163, 19.99062499938548143, 26.74683588394047007 ) ) ;
#19153=CARTESIAN_POINT ( 'NONE',  ( -1.071796769724490339, 18.03259618943233633, 26.00000000000000000 ) ) ;
#19175=EDGE_CURVE ( 'NONE', #29564, #69714, #33769, .T. ) ;
#19177=VECTOR ( 'NONE', #54167, 1000.000000000000000 ) ;
#19186=CARTESIAN_POINT ( 'NONE',  ( -3.756430356250000102, 18.82812499938548356, 30.00000000000000000 ) ) ;
#19199=EDGE_CURVE ( 'NONE', #71220, #7083, #59197, .T. ) ;
#19224=CARTESIAN_POINT ( 'NONE',  ( -3.794534703783686069, 25.05380129398097822, 31.29271267519124322 ) ) ;
#19239=CARTESIAN_POINT ( 'NONE',  ( -3.756430356250000990, 18.75312499938548427, 32.16877607737301048 ) ) ;
#19270=CARTESIAN_POINT ( 'NONE',  ( 0.6945855708053418898, 20.89427347822356040, 33.93923227099254092 ) ) ;
#19271=EDGE_CURVE ( 'NONE', #60913, #7096, #13465, .T. ) ;
#19285=EDGE_LOOP ( 'NONE', ( #35800, #17561, #34599, #70282 ) ) ;
#19328=CARTESIAN_POINT ( 'NONE',  ( -4.000000000000000888, 14.11250000000000071, 32.30940107675850470 ) ) ;
#19331=VECTOR ( 'NONE', #54461, 1000.000000000000000 ) ;
#19335=CARTESIAN_POINT ( 'NONE',  ( -7.967954043666661671E-16, 17.92812499938548498, 34.33755215474603517 ) ) ;
#19345=CARTESIAN_POINT ( 'NONE',  ( 2.655984681222220721E-16, 15.45312499938548179, 25.66244784525396483 ) ) ;
#19359=CARTESIAN_POINT ( 'NONE',  ( -3.999999999999999556, 14.43124999877096570, 27.69059892324149175 ) ) ;
#19369=EDGE_CURVE ( 'NONE', #70824, #9005, #10164, .T. ) ;
#19392=CARTESIAN_POINT ( 'NONE',  ( 1.878215178124997609, 18.07812499938548356, 33.25316411605952993 ) ) ;
#19430=CARTESIAN_POINT ( 'NONE',  ( 5.810221930991193690E-16, 17.95624999877096784, 26.00000000000000000 ) ) ;
#19433=CARTESIAN_POINT ( 'NONE',  ( -1.071796769724502107, 19.32634618820330630, 26.00000000000000711 ) ) ;
#19497=CARTESIAN_POINT ( 'NONE',  ( 4.000000000000000000, 13.40000000000000036, 30.00000000000000000 ) ) ;
#19507=DIRECTION ( 'NONE',  ( 0.000000000000000000, 0.000000000000000000, -1.000000000000000000 ) ) ;
#19515=CARTESIAN_POINT ( 'NONE',  ( 3.756430356250000102, 20.40312499938548285, 30.00000000000000000 ) ) ;
#19517=CARTESIAN_POINT ( 'NONE',  ( -1.999999999999999112, 15.35000000000000142, 26.53589838486224650 ) ) ;
#19553=ORIENTED_EDGE ( 'NONE', *, *, #32305, .F. ) ;
#19596=CARTESIAN_POINT ( 'NONE',  ( 2.655984681222220721E-16, 12.86562499938548321, 25.66244784525396483 ) ) ;
#19609=CARTESIAN_POINT ( 'NONE',  ( -3.756430356250000990, 20.10312499938548925, 32.16877607737301048 ) ) ;
#19642=CARTESIAN_POINT ( 'NONE',  ( 4.000000000000000000, 20.58124999877096784, 27.69059892324149530 ) ) ;
#19650=CARTESIAN_POINT ( 'NONE',  ( 2.000000000000000444, 18.87500000000000000, 26.53589838486224650 ) ) ;
#19681=ORIENTED_EDGE ( 'NONE', *, *, #33045, .T. ) ;
#19699=CARTESIAN_POINT ( 'NONE',  ( 1.878215178124997609, 13.01562499938548356, 33.25316411605952993 ) ) ;
#19706=CARTESIAN_POINT ( 'NONE',  ( 1.878215178125000495, 17.21562499938548285, 26.74683588394047007 ) ) ;
#19716=CARTESIAN_POINT ( 'NONE',  ( 1.878215178124997609, 15.71562499938548108, 33.25316411605952993 ) ) ;
#19724=CARTESIAN_POINT ( 'NONE',  ( -1.243387493232115393E-14, 14.86250000000000071, 26.00000000000000000 ) ) ;
#19733=DIRECTION ( 'NONE',  ( 0.000000000000000000, 0.000000000000000000, -1.000000000000000000 ) ) ;
#19759=CARTESIAN_POINT ( 'NONE',  ( -1.071796769724502107, 18.48259618943233207, 26.00000000000000711 ) ) ;
#19766=CARTESIAN_POINT ( 'NONE',  ( 3.756430356249998770, 19.91562499938548925, 32.16877607737301759 ) ) ;
#19771=VERTEX_POINT ( 'NONE', #41149 ) ;
#19843=EDGE_CURVE ( 'NONE', #64855, #68118, #38962, .T. ) ;
#19863=FACE_OUTER_BOUND ( 'NONE', #57754, .T. ) ;
#19868=CARTESIAN_POINT ( 'NONE',  ( 0.2655917726329427575, 25.54316770519903557, 26.00000000000000711 ) ) ;
#19886=CARTESIAN_POINT ( 'NONE',  ( -1.878215178124999163, 12.79062499938548392, 26.74683588394047007 ) ) ;
#19888=CARTESIAN_POINT ( 'NONE',  ( -3.999999999999999556, 14.03750000000000142, 27.69059892324149175 ) ) ;
#19900=DIRECTION ( 'NONE',  ( -1.000000000000000000, -0.000000000000000000, -0.000000000000000000 ) ) ;
#19953=CARTESIAN_POINT ( 'NONE',  ( -1.626862140677534273E-15, 20.43124999877096570, 34.00000000000000000 ) ) ;
#19955=EDGE_CURVE ( 'NONE', #46020, #69015, #23550, .T. ) ;
#19965=CARTESIAN_POINT ( 'NONE',  ( 3.756430356250000102, 14.10312499938548392, 30.00000000000000000 ) ) ;
#19976=CARTESIAN_POINT ( 'NONE',  ( 1.878215178124997609, 20.21562499938548285, 33.25316411605952993 ) ) ;
#19987=CARTESIAN_POINT ( 'NONE',  ( 3.999999999999998668, 14.65624999877096890, 32.30940107675850470 ) ) ;
#20006=CARTESIAN_POINT ( 'NONE',  ( -1.878215178125001827, 14.40312499938548463, 33.25316411605952283 ) ) ;
#20029=CARTESIAN_POINT ( 'NONE',  ( 3.999999999999998668, 20.11249999999999716, 32.30940107675850470 ) ) ;
#20056=ORIENTED_EDGE ( 'NONE', *, *, #34930, .F. ) ;
#20067=CARTESIAN_POINT ( 'NONE',  ( -0.6941602726958887581, 20.61426555956768780, 33.93677853444431491 ) ) ;
#20076=CARTESIAN_POINT ( 'NONE',  ( 3.756430356249998770, 16.65312499938548285, 32.16877607737302469 ) ) ;
#20091=CARTESIAN_POINT ( 'NONE',  ( 1.999999999999997335, 15.96874999877096535, 33.46410161513775705 ) ) ;
#20101=( BOUNDED_CURVE ( )  B_SPLINE_CURVE ( 2, ( #69216, #63290, #2332, #18574, #41141, #51852, #30036, #52575, #18932 ),
 .UNSPECIFIED., .F., .F. ) 
 B_SPLINE_CURVE_WITH_KNOTS ( ( 3, 2, 2, 2, 3 ),
 ( 0.06944444444444444753, 0.07407407407407406996, 0.08333333333333332871, 0.09259259259259258745, 0.09722222222222222376 ),
 .UNSPECIFIED. ) 
 CURVE ( )  GEOMETRIC_REPRESENTATION_ITEM ( )  RATIONAL_B_SPLINE_CURVE ( ( 0.9330127018922192983, 0.9330127018922194093, 1.000000000000000000, 0.8660254037844387076, 1.000000000000000000, 0.8660254037844387076, 1.000000000000000000, 0.9330127018922191873, 0.9330127018922192983 ) ) 
 REPRESENTATION_ITEM ( '' )  );
#20103=EDGE_CURVE ( 'NONE', #67424, #41970, #31791, .T. ) ;
#20126=CARTESIAN_POINT ( 'NONE',  ( -1.878215178125001827, 18.45312499938548356, 33.25316411605952283 ) ) ;
#20142=( BOUNDED_CURVE ( )  B_SPLINE_CURVE ( 2, ( #36700, #2729, #3835, #41883, #71425, #25244, #42980, #64411, #47793, #70323, #19699, #42252, #14166, #31159, #25623, #65511, #48160, #65140, #14531, #54074, #37065, #9002, #14898, #59960, #37439, #120, #5653, #72155, #32263, #50717, #22625, #32630, #49992, #66243, #45176, #71798, #5283, #67707, #17079, #55894, #39640, #10821, #16354, #27829, #4202, #72516, #9729, #21905, #38541, #61786, #32992, #50361, #10101, #21534, #11190, #33356, #15992, #55170, #33717, #49265, #56262, #43720, #60686, #15621, #61428, #66616, #44461, #66992, #55532, #67356, #44089, #28188, #54795, #26730, #72888, #38909, #4566, #4926, #61065, #21167, #22269, #38163, #44821, #27096, #10462, #49628, #27461, #16719, #39274, #18152, #11910, #39998, #40719, #34435, #23349, #6734, #45898, #56963, #6367, #28899, #51438, #56611, #840, #68429, #68072, #62512, #17441, #18521, #6006, #11555, #18878, #63236, #62871, #17792, #69520, #28541, #24435, #45543, #51798, #58045, #40352, #12267, #62158, #34797, #57330, #29268, #1201, #23706, #35524, #46257, #68796, #12630, #57689, #51076, #52160, #35165, #7094, #29623, #12988, #1563, #24073, #46618, #69162, #41086, #63598, #34071, #473, #22981, #7453, #29980, #52521, #1930, #46984, #8545, #8180, #14809, #47340, #2639, #30708, #36980, #58405, #42529, #69874, #19239, #65420, #3004, #31446, #25158, #64692, #70236, #59875, #9280, #31073, #41441, #70970, #8915, #31814, #37353, #53241, #63959, #54353, #53987, #13343, #20345, #70603, #42896, #48446, #3384, #25906, #3746, #7818, #47699, #65055, #48075, #14446, #35880, #53613, #26271, #25533, #19609, #48808, #59502, #19976, #71337, #30353, #52882, #2280, #24797, #41794, #58771, #42166, #59137, #64322, #13714, #36256 ),
 .UNSPECIFIED., .F., .F. ) 
 B_SPLINE_CURVE_WITH_KNOTS ( ( 3, 2, 2, 2, 2, 2, 2, 2, 2, 2, 2, 2, 2, 2, 2, 2, 2, 2, 2, 2, 2, 2, 2, 2, 2, 2, 2, 2, 2, 2, 2, 2, 2, 2, 2, 2, 2, 2, 2, 2, 2, 2, 2, 2, 2, 2, 2, 2, 2, 2, 2, 2, 2, 2, 2, 2, 2, 2, 2, 2, 2, 2, 2, 2, 2, 2, 2, 2, 2, 2, 2, 2, 2, 2, 2, 2, 2, 2, 2, 2, 2, 2, 2, 2, 2, 2, 2, 2, 2, 2, 2, 2, 2, 2, 2, 2, 2, 2, 2, 2, 2, 2, 2, 2, 2, 2, 2, 3 ),
 ( 0.000000000000000000, 0.009375299769173351880, 0.01875059953834670376, 0.02812589930752005737, 0.03750119907669340752, 0.04687649884586676113, 0.05625179861504011475, 0.06562709838421346142, 0.07500239815338681504, 0.08437769792256016865, 0.09375299769173352227, 0.1031282974609068759, 0.1125035972300802295, 0.1218788969992535831, 0.1312541967684269228, 0.1406294965376002903, 0.1500047963067736301, 0.1593800960759469976, 0.1687553958451203373, 0.1781306956142937048, 0.1875059953834670445, 0.1968812951526404120, 0.2062565949218137518, 0.2156318946909871193, 0.2250071944601604590, 0.2343824942293338265, 0.2437577939985071662, 0.2531330937676805615, 0.2625083935368538457, 0.2718836933060272409, 0.2812589930752005807, 0.2906342928443739204, 0.3000095926135472602, 0.3093848923827206554, 0.3187601921518939951, 0.3281354919210673349, 0.3375107916902406746, 0.3468860914594140699, 0.3562613912285874096, 0.3656366909977607493, 0.3750119907669340891, 0.3843872905361074843, 0.3937625903052808241, 0.4031378900744541638, 0.4125131898436275035, 0.4218884896128008988, 0.4312637893819742385, 0.4406390891511475782, 0.4500143889203209180, 0.4593896886894943132, 0.4687649884586676530, 0.4781402882278409927, 0.4875155879970143324, 0.4968908877661877277, 0.5062661875353611229, 0.5156414873045345182, 0.5250167870737076914, 0.5343920868428810866, 0.5437673866120544819, 0.5531426863812277661, 0.5625179861504011614, 0.5718932859195744456, 0.5812685856887478408, 0.5906438854579212361, 0.6000191852270945203, 0.6093944849962679156, 0.6187697847654413108, 0.6281450845346145950, 0.6375203843037879903, 0.6468956840729612745, 0.6562709838421346698, 0.6656462836113080650, 0.6750215833804813492, 0.6843968831496547445, 0.6937721829188281397, 0.7031474826880014239, 0.7125227824571748192, 0.7218980822263481034, 0.7312733819955214987, 0.7406486817646948939, 0.7500239815338681781, 0.7593992813030415734, 0.7687745810722149686, 0.7781498808413882529, 0.7875251806105616481, 0.7969004803797350434, 0.8062757801489083276, 0.8156510799180817228, 0.8250263796872550071, 0.8344016794564284023, 0.8437769792256017976, 0.8531522789947750818, 0.8625275787639484770, 0.8719028785331218723, 0.8812781783022951565, 0.8906534780714685517, 0.9000287778406418360, 0.9094040776098152312, 0.9187793773789886265, 0.9281546771481619107, 0.9375299769173353059, 0.9469052766865087012, 0.9562805764556819854, 0.9656558762248553807, 0.9750311759940286649, 0.9844064757632020601, 0.9937817755323754554, 1.000000000000000000 ),
 .UNSPECIFIED. ) 
 CURVE ( )  GEOMETRIC_REPRESENTATION_ITEM ( )  RATIONAL_B_SPLINE_CURVE ( ( 1.000000000000000000, 0.8660254037844387076, 1.000000000000000000, 0.8660254037844387076, 1.000000000000000000, 0.8660254037844387076, 1.000000000000000000, 0.8660254037844387076, 1.000000000000000000, 0.8660254037844387076, 1.000000000000000000, 0.8660254037844387076, 1.000000000000000000, 0.8660254037844387076, 1.000000000000000000, 0.8660254037844387076, 1.000000000000000000, 0.8660254037844387076, 1.000000000000000000, 0.8660254037844387076, 1.000000000000000000, 0.8660254037844387076, 1.000000000000000000, 0.8660254037844387076, 1.000000000000000000, 0.8660254037844387076, 1.000000000000000000, 0.8660254037844387076, 1.000000000000000000, 0.8660254037844387076, 1.000000000000000000, 0.8660254037844387076, 1.000000000000000000, 0.8660254037844387076, 1.000000000000000000, 0.8660254037844387076, 1.000000000000000000, 0.8660254037844387076, 1.000000000000000000, 0.8660254037844387076, 1.000000000000000000, 0.8660254037844387076, 1.000000000000000000, 0.8660254037844387076, 1.000000000000000000, 0.8660254037844387076, 1.000000000000000000, 0.8660254037844387076, 1.000000000000000000, 0.8660254037844387076, 1.000000000000000000, 0.8660254037844387076, 1.000000000000000000, 0.8660254037844387076, 1.000000000000000000, 0.8660254037844387076, 1.000000000000000000, 0.8660254037844387076, 1.000000000000000000, 0.8660254037844387076, 1.000000000000000000, 0.8660254037844387076, 1.000000000000000000, 0.8660254037844387076, 1.000000000000000000, 0.8660254037844387076, 1.000000000000000000, 0.8660254037844387076, 1.000000000000000000, 0.8660254037844387076, 1.000000000000000000, 0.8660254037844387076, 1.000000000000000000, 0.8660254037844387076, 1.000000000000000000, 0.8660254037844387076, 1.000000000000000000, 0.8660254037844387076, 1.000000000000000000, 0.8660254037844387076, 1.000000000000000000, 0.8660254037844387076, 1.000000000000000000, 0.8660254037844387076, 1.000000000000000000, 0.8660254037844387076, 1.000000000000000000, 0.8660254037844387076, 1.000000000000000000, 0.8660254037844387076, 1.000000000000000000, 0.8660254037844387076, 1.000000000000000000, 0.8660254037844387076, 1.000000000000000000, 0.8660254037844387076, 1.000000000000000000, 0.8660254037844387076, 1.000000000000000000, 0.8660254037844387076, 1.000000000000000000, 0.8660254037844387076, 1.000000000000000000, 0.8660254037844387076, 1.000000000000000000, 0.8660254037844387076, 1.000000000000000000, 0.8660254037844387076, 1.000000000000000000, 0.8660254037844387076, 1.000000000000000000, 0.8660254037844387076, 1.000000000000000000, 0.8660254037844387076, 1.000000000000000000, 0.8660254037844387076, 1.000000000000000000, 0.8660254037844387076, 1.000000000000000000, 0.8660254037844387076, 1.000000000000000000, 0.8660254037844387076, 1.000000000000000000, 0.8660254037844387076, 1.000000000000000000, 0.8660254037844387076, 1.000000000000000000, 0.8660254037844387076, 1.000000000000000000, 0.8660254037844387076, 1.000000000000000000, 0.8660254037844387076, 1.000000000000000000, 0.8660254037844387076, 1.000000000000000000, 0.8660254037844387076, 1.000000000000000000, 0.8660254037844387076, 1.000000000000000000, 0.8660254037844387076, 1.000000000000000000, 0.8660254037844387076, 1.000000000000000000, 0.8660254037844387076, 1.000000000000000000, 0.8660254037844387076, 1.000000000000000000, 0.8660254037844387076, 1.000000000000000000, 0.8660254037844387076, 1.000000000000000000, 0.8660254037844387076, 1.000000000000000000, 0.8660254037844387076, 1.000000000000000000, 0.8660254037844387076, 1.000000000000000000, 0.8660254037844387076, 1.000000000000000000, 0.8660254037844387076, 1.000000000000000000, 0.8660254037844387076, 1.000000000000000000, 0.8660254037844387076, 1.000000000000000000, 0.8660254037844387076, 1.000000000000000000, 0.8660254037844387076, 1.000000000000000000, 0.8660254037844387076, 1.000000000000000000, 0.8660254037844387076, 1.000000000000000000, 0.8660254037844387076, 1.000000000000000000, 0.8660254037844387076, 1.000000000000000000, 0.8660254037844387076, 1.000000000000000000, 0.8660254037844387076, 1.000000000000000000, 0.8660254037844387076, 1.000000000000000000, 0.8660254037844387076, 1.000000000000000000, 0.8660254037844387076, 1.000000000000000000, 0.8660254037844387076, 1.000000000000000000, 0.8660254037844387076, 1.000000000000000000, 0.8660254037844387076, 1.000000000000000000, 0.8660254037844387076, 1.000000000000000000, 0.8660254037844387076, 1.000000000000000000, 0.8660254037844387076, 1.000000000000000000, 0.8660254037844387076, 1.000000000000000000, 0.8660254037844387076, 1.000000000000000000, 0.8660254037844387076, 1.000000000000000000, 0.8660254037844387076, 1.000000000000000000, 0.8660254037844387076, 1.000000000000000000, 0.8660254037844387076, 1.000000000000000000, 0.8660254037844387076, 1.000000000000000000, 0.9111405360107026619, 0.9401542295230078672 ) ) 
 REPRESENTATION_ITEM ( '' )  );
#20160=LINE ( 'NONE', #26086, #69872 ) ;
#20220=CARTESIAN_POINT ( 'NONE',  ( 1.071796769724491227, 17.09240381056766367, 26.00000000000000000 ) ) ;
#20248=CARTESIAN_POINT ( 'NONE',  ( -3.756430356250001434, 19.76562499938548356, 32.16877607737301048 ) ) ;
#20250=CARTESIAN_POINT ( 'NONE',  ( -8.484601909799255319E-16, 15.08750000000000036, 34.61880215351700940 ) ) ;
#20262=FACE_OUTER_BOUND ( 'NONE', #32096, .T. ) ;
#20332=CARTESIAN_POINT ( 'NONE',  ( 1.878215178125000495, 14.62812499938548427, 26.74683588394047007 ) ) ;
#20345=CARTESIAN_POINT ( 'NONE',  ( 2.655984681222220721E-16, 19.50312499938548427, 25.66244784525396483 ) ) ;
#20356=CARTESIAN_POINT ( 'NONE',  ( 1.071796769724491227, 14.78615380933863044, 26.00000000000000000 ) ) ;
#20376=CARTESIAN_POINT ( 'NONE',  ( 3.756430356250000546, 15.94062499938548427, 27.83122392262697886 ) ) ;
#20384=CARTESIAN_POINT ( 'NONE',  ( 2.393811435568372112E-14, 18.23750000000000071, 34.00000000000000000 ) ) ;
#20389=EDGE_LOOP ( 'NONE', ( #69940, #45298, #34513, #27593 ) ) ;
#20418=CYLINDRICAL_SURFACE ( 'NONE', #1883, 4.000000000000000000 ) ;
#20423=ORIENTED_EDGE ( 'NONE', *, *, #6209, .F. ) ;
#20447=CARTESIAN_POINT ( 'NONE',  ( 2.655984681222220721E-16, 16.80312499938548143, 25.66244784525396483 ) ) ;
#20460=CARTESIAN_POINT ( 'NONE',  ( -2.000000000000001776, 17.24374999877096570, 33.46410161513775705 ) ) ;
#20464=ORIENTED_EDGE ( 'NONE', *, *, #23875, .T. ) ;
#20488=CARTESIAN_POINT ( 'NONE',  ( -5.000000000000000000, 39.99999999999999289, 30.00000000000000000 ) ) ;
#20491=CARTESIAN_POINT ( 'NONE',  ( 3.756430356250000102, 19.50312499938548072, 30.00000000000000000 ) ) ;
#20498=CARTESIAN_POINT ( 'NONE',  ( 4.000000000000000000, 12.69687499938548392, 30.00000000000000000 ) ) ;
#20501=CARTESIAN_POINT ( 'NONE',  ( -1.999999999999999112, 20.29999999999999716, 26.53589838486224650 ) ) ;
#20541=FACE_OUTER_BOUND ( 'NONE', #66466, .T. ) ;
#20561=ORIENTED_EDGE ( 'NONE', *, *, #42309, .T. ) ;
#20586=CARTESIAN_POINT ( 'NONE',  ( -3.756430356250000990, 13.46562499938548285, 32.16877607737301048 ) ) ;
#20605=VECTOR ( 'NONE', #57741, 1000.000000000000000 ) ;
#20616=CARTESIAN_POINT ( 'NONE',  ( -1.878215178124999163, 13.24062499938548321, 26.74683588394047007 ) ) ;
#20618=CARTESIAN_POINT ( 'NONE',  ( 3.999999999999998668, 14.26250000000000107, 32.30940107675850470 ) ) ;
#20629=FACE_BOUND ( 'NONE', #22442, .T. ) ;
#20644=CARTESIAN_POINT ( 'NONE',  ( 2.393811435568372112E-14, 18.63124999877096855, 34.00000000000000000 ) ) ;
#20659=MANIFOLD_SOLID_BREP ( 'Thread1', #48907 ) ;
#20661=ADVANCED_FACE ( 'NONE', ( #57213 ), #11800, .T. ) ;
#20696=FACE_OUTER_BOUND ( 'NONE', #19058, .T. ) ;
#20701=CARTESIAN_POINT ( 'NONE',  ( 1.878215178125000495, 13.27812499938548285, 26.74683588394047007 ) ) ;
#20734=AXIS2_PLACEMENT_3D ( 'NONE', #3081, #25609, #52594 ) ;
#20745=CARTESIAN_POINT ( 'NONE',  ( -3.756430356250001434, 14.36562499938548143, 32.16877607737301048 ) ) ;
#20770=CARTESIAN_POINT ( 'NONE',  ( -1.626862140677534273E-15, 20.03749999999999787, 34.00000000000000000 ) ) ;
#20771=CARTESIAN_POINT ( 'NONE',  ( -1.071796769724491671, 13.47634618820330132, 26.00000000000000355 ) ) ;
#20791=CARTESIAN_POINT ( 'NONE',  ( -3.999999999999999112, 19.83124999877096784, 27.69059892324149530 ) ) ;
#20802=CARTESIAN_POINT ( 'NONE',  ( -4.000000000000000000, 14.07500000000000107, 30.00000000000000000 ) ) ;
#20804=FACE_OUTER_BOUND ( 'NONE', #2453, .T. ) ;
#20805=ORIENTED_EDGE ( 'NONE', *, *, #26971, .F. ) ;
#20818=CARTESIAN_POINT ( 'NONE',  ( -7.967954043666661671E-16, 16.57812499938548356, 34.33755215474603517 ) ) ;
#20827=CARTESIAN_POINT ( 'NONE',  ( -1.243387493232115393E-14, 15.31250000000000000, 26.00000000000000000 ) ) ;
#20835=CARTESIAN_POINT ( 'NONE',  ( 2.828200636599751609E-16, 17.05624999877096570, 25.38119784648299415 ) ) ;
#20849=( BOUNDED_CURVE ( )  B_SPLINE_CURVE ( 1, ( #30562, #25378 ),
 .UNSPECIFIED., .F., .F. ) 
 B_SPLINE_CURVE_WITH_KNOTS ( ( 2, 2 ),
 ( 0.000000000000000000, 1.000000000000000000 ),
 .UNSPECIFIED. ) 
 CURVE ( )  GEOMETRIC_REPRESENTATION_ITEM ( )  RATIONAL_B_SPLINE_CURVE ( ( 0.9401542295230078672, 0.9401542295230078672 ) ) 
 REPRESENTATION_ITEM ( '' )  );
#20857=EDGE_CURVE ( 'NONE', #44824, #18463, #50224, .T. ) ;
#20869=CARTESIAN_POINT ( 'NONE',  ( -0.6941636114358130660, 20.72676549290719450, 33.93677660682192965 ) ) ;
#20870=CARTESIAN_POINT ( 'NONE',  ( -1.071796769724490339, 14.43259618943233313, 26.00000000000000000 ) ) ;
#20882=ORIENTED_EDGE ( 'NONE', *, *, #32902, .F. ) ;
#20949=CARTESIAN_POINT ( 'NONE',  ( -3.756430356250001434, 14.25312499938548250, 32.16877607737301048 ) ) ;
#20954=CARTESIAN_POINT ( 'NONE',  ( -2.672702088255949472E-15, 13.51250000000000107, 26.00000000000000000 ) ) ;
#20957=FACE_OUTER_BOUND ( 'NONE', #43211, .T. ) ;
#20982=ORIENTED_EDGE ( 'NONE', *, *, #721, .F. ) ;
#20986=CARTESIAN_POINT ( 'NONE',  ( -1.878215178124999163, 19.65312499938548285, 26.74683588394047007 ) ) ;
#20988=CARTESIAN_POINT ( 'NONE',  ( -3.999999999999999556, 14.93750000000000000, 27.69059892324149175 ) ) ;
#21036=EDGE_CURVE ( 'NONE', #18562, #49631, #8308, .T. ) ;
#21068=CYLINDRICAL_SURFACE ( 'NONE', #58471, 4.000000000000000000 ) ;
#21073=CARTESIAN_POINT ( 'NONE',  ( 1.878215178124997609, 13.12812499938548427, 33.25316411605952993 ) ) ;
#21114=CARTESIAN_POINT ( 'NONE',  ( -1.878215178125001827, 13.95312499938548356, 33.25316411605952283 ) ) ;
#21139=FACE_OUTER_BOUND ( 'NONE', #31759, .T. ) ;
#21153=FACE_OUTER_BOUND ( 'NONE', #2322, .T. ) ;
#21155=ADVANCED_FACE ( 'NONE', ( #51499 ), #24128, .T. ) ;
#21163=VERTEX_POINT ( 'NONE', #45601 ) ;
#21167=CARTESIAN_POINT ( 'NONE',  ( -3.756430356250000990, 15.60312499938548392, 32.16877607737301048 ) ) ;
#21173=CARTESIAN_POINT ( 'NONE',  ( 3.756430356250000102, 18.94062499938548427, 30.00000000000000000 ) ) ;
#21183=CARTESIAN_POINT ( 'NONE',  ( -3.756430356249999214, 17.77812499938548285, 27.83122392262697531 ) ) ;
#21199=CARTESIAN_POINT ( 'NONE',  ( -8.484601909799255319E-16, 16.83124999877096784, 34.61880215351700940 ) ) ;
#21232=CARTESIAN_POINT ( 'NONE',  ( 1.878215178124997609, 19.42812499938548143, 33.25316411605952993 ) ) ;
#21246=ORIENTED_EDGE ( 'NONE', *, *, #10213, .T. ) ;
#21251=CARTESIAN_POINT ( 'NONE',  ( 4.000000000000000000, 19.28749999999999787, 27.69059892324149885 ) ) ;
#21291=ADVANCED_FACE ( 'NONE', ( #33775 ), #17498, .T. ) ;
#21295=DIRECTION ( 'NONE',  ( 0.000000000000000000, 0.000000000000000000, -1.000000000000000000 ) ) ;
#21313=EDGE_CURVE ( 'NONE', #29801, #16672, #30946, .T. ) ;
#21316=CARTESIAN_POINT ( 'NONE',  ( -3.756430356250000102, 14.21562499938548285, 30.00000000000000000 ) ) ;
#21324=CARTESIAN_POINT ( 'NONE',  ( -1.878215178124999163, 12.90312499938548463, 26.74683588394047007 ) ) ;
#21342=CARTESIAN_POINT ( 'NONE',  ( -1.626862140677534273E-15, 19.58750000000000213, 34.00000000000000000 ) ) ;
#21350=CARTESIAN_POINT ( 'NONE',  ( -7.967954043666661671E-16, 14.77812499938548463, 34.33755215474603517 ) ) ;
#21352=CARTESIAN_POINT ( 'NONE',  ( -3.999999999999999556, 18.08750000000000213, 27.69059892324149175 ) ) ;
#21400=CARTESIAN_POINT ( 'NONE',  ( -1.999999999999999112, 13.04374999877096641, 26.53589838486224650 ) ) ;
#21415=CARTESIAN_POINT ( 'NONE',  ( 5.810221930991193690E-16, 17.95624999877096428, 26.00000000000000000 ) ) ;
#21418=DIRECTION ( 'NONE',  ( -0.000000000000000000, -1.000000000000000000, -0.000000000000000000 ) ) ;
#21434=CARTESIAN_POINT ( 'NONE',  ( 3.756430356250000546, 15.94062499938548427, 27.83122392262697886 ) ) ;
#21443=CARTESIAN_POINT ( 'NONE',  ( 1.071796769724485232, 16.58615380933862937, 25.99999999999999645 ) ) ;
#21447=ORIENTED_EDGE ( 'NONE', *, *, #721, .T. ) ;
#21451=B_SPLINE_CURVE_WITH_KNOTS ( 'NONE', 1,
 ( #724, #50598 ),
 .UNSPECIFIED., .F., .F.,
 ( 2, 2 ),
 ( 0.000000000000000000, 1.000000000000000000 ),
 .UNSPECIFIED. ) ;
#21480=CARTESIAN_POINT ( 'NONE',  ( 2.655984681222220721E-16, 16.01562499938548356, 25.66244784525396483 ) ) ;
#21534=CARTESIAN_POINT ( 'NONE',  ( -3.756430356249999214, 14.62812499938548427, 27.83122392262697176 ) ) ;
#21540=CARTESIAN_POINT ( 'NONE',  ( -3.756430356250000102, 19.16562499938548214, 30.00000000000000000 ) ) ;
#21550=CARTESIAN_POINT ( 'NONE',  ( -3.756430356249999214, 17.32812499938548356, 27.83122392262697531 ) ) ;
#21567=CARTESIAN_POINT ( 'NONE',  ( 4.000000000000000000, 16.94374999877096499, 30.00000000000000000 ) ) ;
#21570=DIRECTION ( 'NONE',  ( -0.000000000000000000, -1.000000000000000000, -0.000000000000000000 ) ) ;
#21577=CARTESIAN_POINT ( 'NONE',  ( -2.000000000000001776, 16.34374999877096712, 33.46410161513775705 ) ) ;
#21629=CARTESIAN_POINT ( 'NONE',  ( 5.810221930991193690E-16, 14.80624999877096570, 26.00000000000000000 ) ) ;
#21680=CARTESIAN_POINT ( 'NONE',  ( -3.756430356249999214, 14.17812499938548498, 27.83122392262697531 ) ) ;
#21682=CARTESIAN_POINT ( 'NONE',  ( 4.898587196589412829E-16, 27.50000000000000000, 34.00000000000000000 ) ) ;
#21686=CARTESIAN_POINT ( 'NONE',  ( 4.898587196589412829E-16, 27.50000000000000000, 34.00000000000000000 ) ) ;
#21687=( BOUNDED_CURVE ( )  B_SPLINE_CURVE ( 2, ( #57300, #11881, #50333, #17761, #6705, #56933, #46226, #18123, #6337 ),
 .UNSPECIFIED., .F., .F. ) 
 B_SPLINE_CURVE_WITH_KNOTS ( ( 3, 2, 2, 2, 3 ),
 ( 0.2638888888888888951, 0.2685185185185185452, 0.2777777777777777901, 0.2870370370370370350, 0.2916666666666666852 ),
 .UNSPECIFIED. ) 
 CURVE ( )  GEOMETRIC_REPRESENTATION_ITEM ( )  RATIONAL_B_SPLINE_CURVE ( ( 0.9330127018922194093, 0.9330127018922194093, 1.000000000000000000, 0.8660254037844387076, 1.000000000000000000, 0.8660254037844387076, 1.000000000000000000, 0.9330127018922189652, 0.9330127018922194093 ) ) 
 REPRESENTATION_ITEM ( '' )  );
#21690=CARTESIAN_POINT ( 'NONE',  ( -3.756430356250000102, 13.87812499938548250, 30.00000000000000000 ) ) ;
#21716=CARTESIAN_POINT ( 'NONE',  ( 3.756430356250000102, 15.34062499938548285, 30.00000000000000000 ) ) ;
#21718=CARTESIAN_POINT ( 'NONE',  ( -3.999999999999999556, 16.73750000000000071, 27.69059892324149175 ) ) ;
#21762=CARTESIAN_POINT ( 'NONE',  ( -1.071796769724490339, 20.22634618820329777, 26.00000000000000000 ) ) ;
#21763=DIRECTION ( 'NONE',  ( -0.000000000000000000, -1.000000000000000000, -0.000000000000000000 ) ) ;
#21794=CARTESIAN_POINT ( 'NONE',  ( 5.810221930991193690E-16, 17.95624999877096784, 26.00000000000000000 ) ) ;
#21799=CARTESIAN_POINT ( 'NONE',  ( 3.756430356250000102, 15.90312499938548108, 30.00000000000000000 ) ) ;
#21845=CARTESIAN_POINT ( 'NONE',  ( 1.878215178125000495, 17.32812499938548356, 26.74683588394047007 ) ) ;
#21859=VECTOR ( 'NONE', #40734, 1000.000000000000000 ) ;
#21869=CARTESIAN_POINT ( 'NONE',  ( -1.071796769724490783, 13.66115380933863399, 34.00000000000000711 ) ) ;
#21874=CARTESIAN_POINT ( 'NONE',  ( 4.898587196589412829E-16, 27.50000000000000000, 34.00000000000000000 ) ) ;
#21905=CARTESIAN_POINT ( 'NONE',  ( 3.756430356249998770, 14.40312499938548463, 32.16877607737301759 ) ) ;
#21921=CARTESIAN_POINT ( 'NONE',  ( 2.655984681222220721E-16, 19.05312499938548143, 25.66244784525396483 ) ) ;
#21936=CARTESIAN_POINT ( 'NONE',  ( -3.999999999999999556, 17.58124999877096784, 27.69059892324149175 ) ) ;
#21940=CYLINDRICAL_SURFACE ( 'NONE', #72678, 4.000000000000000000 ) ;
#21961=CARTESIAN_POINT ( 'NONE',  ( -1.071796769724490339, 14.37634618820330168, 26.00000000000000000 ) ) ;
#22048=CARTESIAN_POINT ( 'NONE',  ( 3.756430356250000546, 14.02812499938548463, 27.83122392262697886 ) ) ;
#22059=CARTESIAN_POINT ( 'NONE',  ( -1.878215178124999163, 14.25312499938548250, 26.74683588394047007 ) ) ;
#22071=ORIENTED_EDGE ( 'NONE', *, *, #54732, .T. ) ;
#22086=CARTESIAN_POINT ( 'NONE',  ( -3.756430356250000102, 16.01562499938548356, 30.00000000000000000 ) ) ;
#22089=CARTESIAN_POINT ( 'NONE',  ( 4.000000000000000000, 16.55000000000000071, 30.00000000000000000 ) ) ;
#22152=CYLINDRICAL_SURFACE ( 'NONE', #51052, 4.000000000000000000 ) ;
#22162=FACE_OUTER_BOUND ( 'NONE', #33877, .T. ) ;
#22166=DIRECTION ( 'NONE',  ( 0.000000000000000000, 0.000000000000000000, -1.000000000000000000 ) ) ;
#22171=CARTESIAN_POINT ( 'NONE',  ( 3.756430356250000102, 16.80312499938548498, 30.00000000000000000 ) ) ;
#22214=CARTESIAN_POINT ( 'NONE',  ( 3.756430356250000546, 16.84062499938548285, 27.83122392262697886 ) ) ;
#22269=CARTESIAN_POINT ( 'NONE',  ( -1.878215178125001827, 15.64062499938548356, 33.25316411605952283 ) ) ;
#22284=CARTESIAN_POINT ( 'NONE',  ( -3.756430356249999214, 19.57812499938548001, 27.83122392262697531 ) ) ;
#22298=CARTESIAN_POINT ( 'NONE',  ( 2.000000000000000444, 17.46874999877096712, 26.53589838486224650 ) ) ;
#22301=CARTESIAN_POINT ( 'NONE',  ( 2.000000000000000444, 13.02500000000000036, 26.53589838486224650 ) ) ;
#22332=CYLINDRICAL_SURFACE ( 'NONE', #12290, 4.000000000000000000 ) ;
#22337=ORIENTED_EDGE ( 'NONE', *, *, #16156, .T. ) ;
#22387=CARTESIAN_POINT ( 'NONE',  ( 4.648177544792955741E-15, 14.58124999877096606, 33.99999999999999289 ) ) ;
#22418=CARTESIAN_POINT ( 'NONE',  ( 2.655984681222220721E-16, 14.21562499938548285, 25.66244784525396483 ) ) ;
#22424=PLANE ( 'NONE',  #43113 ) ;
#22442=EDGE_LOOP ( 'NONE', ( #35606, #63871 ) ) ;
#22448=CARTESIAN_POINT ( 'NONE',  ( 1.999999999999997335, 17.37500000000000000, 33.46410161513775705 ) ) ;
#22461=ORIENTED_EDGE ( 'NONE', *, *, #33073, .T. ) ;
#22484=CARTESIAN_POINT ( 'NONE',  ( -2.672702088255949472E-15, 13.45624999877096784, 26.00000000000000000 ) ) ;
#22509=EDGE_CURVE ( 'NONE', #57768, #60913, #67857, .T. ) ;
#22526=CARTESIAN_POINT ( 'NONE',  ( 2.393811435568372112E-14, 16.88750000000000284, 34.00000000000000000 ) ) ;
#22530=CARTESIAN_POINT ( 'NONE',  ( -3.756430356250000102, 16.57812499938548356, 30.00000000000000000 ) ) ;
#22559=EDGE_CURVE ( 'NONE', #64855, #71132, #48053, .T. ) ;
#22572=CARTESIAN_POINT ( 'NONE',  ( 2.655984681222220721E-16, 17.36562499938548498, 25.66244784525396483 ) ) ;
#22593=CARTESIAN_POINT ( 'NONE',  ( -4.000000000000000000, 19.92499999999999716, 30.00000000000000000 ) ) ;
#22622=DIRECTION ( 'NONE',  ( -0.000000000000000000, -1.000000000000000000, -0.000000000000000000 ) ) ;
#22625=CARTESIAN_POINT ( 'NONE',  ( -3.756430356250000102, 13.76562499938548356, 30.00000000000000000 ) ) ;
#22628=ORIENTED_EDGE ( 'NONE', *, *, #3547, .T. ) ;
#22641=CARTESIAN_POINT ( 'NONE',  ( 3.756430356250000102, 19.39062499938548356, 30.00000000000000000 ) ) ;
#22656=CARTESIAN_POINT ( 'NONE',  ( 4.000000000000000000, 17.43124999877096570, 27.69059892324149530 ) ) ;
#22682=CARTESIAN_POINT ( 'NONE',  ( 4.000000000000000000, 14.75000000000000178, 30.00000000000000000 ) ) ;
#22687=CARTESIAN_POINT ( 'NONE',  ( -4.000000000000000000, 20.76874999877096428, 30.00000000000000000 ) ) ;
#22688=CARTESIAN_POINT ( 'NONE',  ( 0.000000000000000000, 27.50000000000000000, 30.00000000000000000 ) ) ;
#22693=ORIENTED_EDGE ( 'NONE', *, *, #72495, .T. ) ;
#22740=( LENGTH_UNIT ( ) NAMED_UNIT ( * ) SI_UNIT ( .MILLI., .METRE. ) );
#22774=CARTESIAN_POINT ( 'NONE',  ( -1.878215178124999163, 14.70312499938548356, 26.74683588394047007 ) ) ;
#22805=CARTESIAN_POINT ( 'NONE',  ( 4.000000000000000000, 18.34999999999999787, 30.00000000000000000 ) ) ;
#22818=ORIENTED_EDGE ( 'NONE', *, *, #59834, .T. ) ;
#22878=CARTESIAN_POINT ( 'NONE',  ( 0.000000000000000000, 27.50000000000000000, 30.00000000000000000 ) ) ;
#22882=CARTESIAN_POINT ( 'NONE',  ( 1.878215178124997609, 16.72812499938548214, 33.25316411605952993 ) ) ;
#22925=CARTESIAN_POINT ( 'NONE',  ( 3.756430356250000546, 17.74062499938548143, 27.83122392262697886 ) ) ;
#22979=CARTESIAN_POINT ( 'NONE',  ( 1.138803498474273873E-14, 15.08749999999999858, 34.00000000000000000 ) ) ;
#22981=CARTESIAN_POINT ( 'NONE',  ( 2.655984681222220721E-16, 18.15312499938548285, 25.66244784525396483 ) ) ;
#22993=AXIS2_PLACEMENT_3D ( 'NONE', #11187, #22622, #23347 ) ;
#23005=AXIS2_PLACEMENT_3D ( 'NONE', #66887, #38810, #28437 ) ;
#23016=CARTESIAN_POINT ( 'NONE',  ( 4.000000000000000000, 18.29374999877096641, 30.00000000000000000 ) ) ;
#23019=CARTESIAN_POINT ( 'NONE',  ( -1.071796769724492115, 17.71115380933863293, 34.00000000000000000 ) ) ;
#23078=ORIENTED_EDGE ( 'NONE', *, *, #49537, .T. ) ;
#23100=CARTESIAN_POINT ( 'NONE',  ( 0.000000000000000000, 0.000000000000000000, 0.000000000000000000 ) ) ;
#23131=CARTESIAN_POINT ( 'NONE',  ( 4.648177544792955741E-15, 13.73749999999999716, 33.99999999999999289 ) ) ;
#23138=CARTESIAN_POINT ( 'NONE',  ( -3.756430356250000102, 15.22812499938548392, 30.00000000000000000 ) ) ;
#23169=CARTESIAN_POINT ( 'NONE',  ( 4.000000000000000000, 19.70000000000000284, 30.00000000000000000 ) ) ;
#23226=CYLINDRICAL_SURFACE ( 'NONE', #47946, 4.000000000000000000 ) ;
#23252=CARTESIAN_POINT ( 'NONE',  ( -3.756430356249999214, 18.79062499938548214, 27.83122392262697531 ) ) ;
#23292=CARTESIAN_POINT ( 'NONE',  ( -1.878215178125001827, 18.45312499938548356, 33.25316411605952283 ) ) ;
#23347=DIRECTION ( 'NONE',  ( 0.000000000000000000, 0.000000000000000000, -1.000000000000000000 ) ) ;
#23349=CARTESIAN_POINT ( 'NONE',  ( 1.878215178124997609, 16.16562499938548569, 33.25316411605952993 ) ) ;
#23379=CARTESIAN_POINT ( 'NONE',  ( -3.999999999999999556, 19.38124999877096499, 27.69059892324149175 ) ) ;
#23422=CARTESIAN_POINT ( 'NONE',  ( 2.393811435568372112E-14, 18.63124999877096855, 34.00000000000000000 ) ) ;
#23437=CARTESIAN_POINT ( 'NONE',  ( -3.999999999999999112, 18.93124999877096570, 27.69059892324149530 ) ) ;
#23441=CARTESIAN_POINT ( 'NONE',  ( 1.878215178124997609, 13.91562499938548392, 33.25316411605952993 ) ) ;
#23453=EDGE_CURVE ( 'NONE', #29842, #46076, #30512, .T. ) ;
#23502=CARTESIAN_POINT ( 'NONE',  ( 2.655984681222220721E-16, 17.36562499938548498, 25.66244784525396483 ) ) ;
#23532=CARTESIAN_POINT ( 'NONE',  ( 1.999999999999997335, 19.62500000000000000, 33.46410161513775705 ) ) ;
#23550=CIRCLE ( 'NONE', #61307, 14.99999999999999822 ) ;
#23573=CARTESIAN_POINT ( 'NONE',  ( 5.810221930991193690E-16, 14.41249999999999787, 26.00000000000000000 ) ) ;
#23615=CARTESIAN_POINT ( 'NONE',  ( 2.655984681222220721E-16, 18.71562499938548285, 25.66244784525396483 ) ) ;
#23617=CARTESIAN_POINT ( 'NONE',  ( 2.828200636599751609E-16, 13.51250000000000107, 25.38119784648299415 ) ) ;
#23655=CARTESIAN_POINT ( 'NONE',  ( -3.756430356250000102, 20.62812499938548072, 30.00000000000000000 ) ) ;
#23679=CARTESIAN_POINT ( 'NONE',  ( 1.626862140677534470E-15, 13.23124999877096819, 34.00000000000000000 ) ) ;
#23695=LINE ( 'NONE', #1918, #55121 ) ;
#23706=CARTESIAN_POINT ( 'NONE',  ( -3.756430356250000990, 17.40312499938548285, 32.16877607737301048 ) ) ;
#23729=CARTESIAN_POINT ( 'NONE',  ( -4.000000000000000888, 17.20624999877096428, 32.30940107675850470 ) ) ;
#23736=CARTESIAN_POINT ( 'NONE',  ( 2.828200636599751609E-16, 20.65624999877096712, 25.38119784648299415 ) ) ;
#23765=AXIS2_PLACEMENT_3D ( 'NONE', #23100, #68190, #46012 ) ;
#23775=VERTEX_POINT ( 'NONE', #44445 ) ;
#23799=CARTESIAN_POINT ( 'NONE',  ( 3.756430356249998770, 16.65312499938548285, 32.16877607737302469 ) ) ;
#23861=CARTESIAN_POINT ( 'NONE',  ( 2.655984681222220721E-16, 18.26562499938548356, 25.66244784525396483 ) ) ;
#23875=EDGE_CURVE ( 'NONE', #8942, #23775, #63535, .T. ) ;
#23895=CARTESIAN_POINT ( 'NONE',  ( -1.999999999999999112, 18.95000000000000284, 26.53589838486224650 ) ) ;
#23927=ORIENTED_EDGE ( 'NONE', *, *, #18114, .F. ) ;
#23958=CARTESIAN_POINT ( 'NONE',  ( 4.898850051585143718E-16, 25.54316770519903557, 34.00000000000000000 ) ) ;
#23975=CARTESIAN_POINT ( 'NONE',  ( 3.756430356250000102, 19.05312499938548143, 30.00000000000000000 ) ) ;
#23977=CARTESIAN_POINT ( 'NONE',  ( 3.756430356250000546, 20.32812499938548356, 27.83122392262697886 ) ) ;
#24013=CARTESIAN_POINT ( 'NONE',  ( 1.878215178124997609, 20.32812499938548356, 33.25316411605952993 ) ) ;
#24073=CARTESIAN_POINT ( 'NONE',  ( -1.878215178125001827, 17.89062499938548356, 33.25316411605952283 ) ) ;
#24084=CARTESIAN_POINT ( 'NONE',  ( -1.626862140677534273E-15, 15.53750000000000142, 34.00000000000000000 ) ) ;
#24102=CARTESIAN_POINT ( 'NONE',  ( -1.878215178124999163, 13.80312499938548321, 26.74683588394047007 ) ) ;
#24111=CARTESIAN_POINT ( 'NONE',  ( -2.498395430326213790E-14, 16.66250000000000497, 26.00000000000000000 ) ) ;
#24128=CYLINDRICAL_SURFACE ( 'NONE', #25724, 15.00000000000000000 ) ;
#24139=ORIENTED_EDGE ( 'NONE', *, *, #70290, .T. ) ;
#24154=EDGE_LOOP ( 'NONE', ( #31043, #69915, #17069, #60763 ) ) ;
#24163=CARTESIAN_POINT ( 'NONE',  ( 3.756430356249998770, 17.55312499938548143, 32.16877607737302469 ) ) ;
#24209=VECTOR ( 'NONE', #2362, 1000.000000000000000 ) ;
#24224=CARTESIAN_POINT ( 'NONE',  ( 1.878215178124997609, 17.62812499938548427, 33.25316411605952993 ) ) ;
#24252=LINE ( 'NONE', #39817, #50135 ) ;
#24294=ORIENTED_EDGE ( 'NONE', *, *, #25301, .F. ) ;
#24295=ORIENTED_EDGE ( 'NONE', *, *, #68559, .F. ) ;
#24336=EDGE_CURVE ( 'NONE', #18463, #44824, #60649, .T. ) ;
#24340=CARTESIAN_POINT ( 'NONE',  ( -7.967954043666661671E-16, 19.39062499938548001, 34.33755215474603517 ) ) ;
#24342=CARTESIAN_POINT ( 'NONE',  ( 1.999999999999997335, 13.77500000000000036, 33.46410161513775705 ) ) ;
#24379=CARTESIAN_POINT ( 'NONE',  ( 1.878215178125000495, 20.02812499938548285, 26.74683588394047007 ) ) ;
#24393=VECTOR ( 'NONE', #3973, 1000.000000000000000 ) ;
#24435=CARTESIAN_POINT ( 'NONE',  ( -1.878215178125001827, 16.99062499938548498, 33.25316411605952283 ) ) ;
#24466=CARTESIAN_POINT ( 'NONE',  ( -4.000000000000000000, 20.76874999877096428, 30.00000000000000000 ) ) ;
#24492=CARTESIAN_POINT ( 'NONE',  ( 0.000000000000000000, 27.50000000000000000, 30.00000000000000000 ) ) ;
#24501=CARTESIAN_POINT ( 'NONE',  ( -2.498395430326213790E-14, 16.66250000000000497, 26.00000000000000000 ) ) ;
#24522=CARTESIAN_POINT ( 'NONE',  ( -1.626862140677534273E-15, 16.83124999877096428, 34.00000000000000000 ) ) ;
#24530=CARTESIAN_POINT ( 'NONE',  ( 1.878215178125000495, 18.11562499938548498, 26.74683588394047007 ) ) ;
#24532=ORIENTED_EDGE ( 'NONE', *, *, #68559, .T. ) ;
#24547=CARTESIAN_POINT ( 'NONE',  ( -4.000000000000000888, 13.66250000000000142, 32.30940107675850470 ) ) ;
#24553=CARTESIAN_POINT ( 'NONE',  ( 2.000000000000000444, 14.76874999877096606, 26.53589838486224650 ) ) ;
#24565=ADVANCED_FACE ( 'NONE', ( #10722 ), #21068, .T. ) ;
#24584=CARTESIAN_POINT ( 'NONE',  ( -1.878215178124999163, 17.85312499938548214, 26.74683588394047007 ) ) ;
#24600=ADVANCED_FACE ( 'NONE', ( #20696 ), #3731, .T. ) ;
#24620=CARTESIAN_POINT ( 'NONE',  ( 5.810221930991193690E-16, 19.81250000000000000, 26.00000000000000000 ) ) ;
#24636=ORIENTED_EDGE ( 'NONE', *, *, #1852, .T. ) ;
#24642=EDGE_CURVE ( 'NONE', #58713, #69279, #10250, .T. ) ;
#24645=CARTESIAN_POINT ( 'NONE',  ( 4.648177544792955741E-15, 14.13124999877096499, 33.99999999999999289 ) ) ;
#24657=CARTESIAN_POINT ( 'NONE',  ( 1.999999999999997335, 18.21874999877096712, 33.46410161513775705 ) ) ;
#24666=CARTESIAN_POINT ( 'NONE',  ( 2.655984681222220721E-16, 12.75312499938548427, 25.66244784525396483 ) ) ;
#24683=CARTESIAN_POINT ( 'NONE',  ( 2.642249610956118655, 25.30481484749465793, 33.01446934944805633 ) ) ;
#24702=CARTESIAN_POINT ( 'NONE',  ( -1.878215178124999163, 17.40312499938548285, 26.74683588394047007 ) ) ;
#24704=CARTESIAN_POINT ( 'NONE',  ( -3.756430356250001434, 20.55312499938548498, 32.16877607737301048 ) ) ;
#24710=CARTESIAN_POINT ( 'NONE',  ( -4.000000000000000888, 18.16249999999999787, 32.30940107675850470 ) ) ;
#24717=VERTEX_POINT ( 'NONE', #11812 ) ;
#24742=CARTESIAN_POINT ( 'NONE',  ( -1.878215178124999163, 20.10312499938548569, 26.74683588394047007 ) ) ;
#24780=CARTESIAN_POINT ( 'NONE',  ( -2.442157805219161926, 25.33991025467384972, 33.17866654912879909 ) ) ;
#24797=CARTESIAN_POINT ( 'NONE',  ( 2.655984681222220721E-16, 20.40312499938548285, 25.66244784525396483 ) ) ;
#24826=CARTESIAN_POINT ( 'NONE',  ( -1.878215178125001827, 13.50312499938548427, 33.25316411605952283 ) ) ;
#24888=CARTESIAN_POINT ( 'NONE',  ( 1.878215178125000495, 18.56562499938548427, 26.74683588394047007 ) ) ;
#24898=CARTESIAN_POINT ( 'NONE',  ( -3.756430356249999214, 16.87812499938548427, 27.83122392262697531 ) ) ;
#24906=CARTESIAN_POINT ( 'NONE',  ( -4.000000000000000000, 13.62500000000000000, 30.00000000000000000 ) ) ;
#24913=CARTESIAN_POINT ( 'NONE',  ( 4.000000000000000000, 12.93124999877096570, 27.69059892324149530 ) ) ;
#24930=DIRECTION ( 'NONE',  ( 0.000000000000000000, 0.000000000000000000, 1.000000000000000000 ) ) ;
#24934=( GEOMETRIC_REPRESENTATION_CONTEXT ( 3 ) GLOBAL_UNCERTAINTY_ASSIGNED_CONTEXT ( ( #42491 ) ) GLOBAL_UNIT_ASSIGNED_CONTEXT ( ( #50473, #28653, #62630 ) ) REPRESENTATION_CONTEXT ( 'NONE', 'WORKASPACE' ) );
#24947=CARTESIAN_POINT ( 'NONE',  ( -1.878215178125001827, 17.10312499938548214, 33.25316411605952283 ) ) ;
#24982=CARTESIAN_POINT ( 'NONE',  ( 2.000000000000000444, 18.42500000000000071, 26.53589838486224650 ) ) ;
#25000=VERTEX_POINT ( 'NONE', #61153 ) ;
#25064=CARTESIAN_POINT ( 'NONE',  ( 3.756430356250000102, 19.95312499938548356, 30.00000000000000000 ) ) ;
#25066=CARTESIAN_POINT ( 'NONE',  ( 2.000000000000000444, 15.27500000000000036, 26.53589838486224650 ) ) ;
#25100=ORIENTED_EDGE ( 'NONE', *, *, #63479, .T. ) ;
#25103=CARTESIAN_POINT ( 'NONE',  ( 2.655984681222220721E-16, 19.61562499938548143, 25.66244784525396483 ) ) ;
#25142=CARTESIAN_POINT ( 'NONE',  ( -2.642701734113356959, 25.30472597034935944, 33.01399490227544220 ) ) ;
#25146=CARTESIAN_POINT ( 'NONE',  ( 2.000000000000000444, 15.72499999999999964, 26.53589838486224650 ) ) ;
#25158=CARTESIAN_POINT ( 'NONE',  ( 3.756430356249998770, 18.90312499938548285, 32.16877607737301759 ) ) ;
#25188=CARTESIAN_POINT ( 'NONE',  ( -4.000000000000000000, 19.86874999877096570, 30.00000000000000000 ) ) ;
#25244=CARTESIAN_POINT ( 'NONE',  ( -3.756430356249999214, 12.82812499938548534, 27.83122392262697176 ) ) ;
#25247=VECTOR ( 'NONE', #259, 1000.000000000000000 ) ;
#25252=CARTESIAN_POINT ( 'NONE',  ( 3.756430356249998770, 17.10312499938548214, 32.16877607737302469 ) ) ;
#25263=CARTESIAN_POINT ( 'NONE',  ( -1.878215178124999163, 15.94062499938548427, 26.74683588394047007 ) ) ;
#25280=FACE_OUTER_BOUND ( 'NONE', #48232, .T. ) ;
#25301=EDGE_CURVE ( 'NONE', #68959, #13783, #55134, .T. ) ;
#25315=CARTESIAN_POINT ( 'NONE',  ( 3.756430356249998770, 19.46562499938548285, 32.16877607737301759 ) ) ;
#25321=ORIENTED_EDGE ( 'NONE', *, *, #28761, .T. ) ;
#25378=CARTESIAN_POINT ( 'NONE',  ( 0.6522905807966048464, 20.75364847883808395, 33.69936292076899065 ) ) ;
#25390=ORIENTED_EDGE ( 'NONE', *, *, #5722, .T. ) ;
#25420=CARTESIAN_POINT ( 'NONE',  ( 1.999999999999997335, 13.32499999999999929, 33.46410161513775705 ) ) ;
#25439=CARTESIAN_POINT ( 'NONE',  ( 1.878215178124997609, 13.46562499938548285, 33.25316411605952993 ) ) ;
#25441=CARTESIAN_POINT ( 'NONE',  ( 4.000000000000000000, 14.75000000000000178, 30.00000000000000000 ) ) ;
#25494=DIRECTION ( 'NONE',  ( -0.000000000000000000, -1.000000000000000000, -0.000000000000000000 ) ) ;
#25496=( BOUNDED_CURVE ( )  B_SPLINE_CURVE ( 2, ( #26656, #70981, #9292, #19987, #71722, #3396, #43645, #20356, #37364 ),
 .UNSPECIFIED., .F., .F. ) 
 B_SPLINE_CURVE_WITH_KNOTS ( ( 3, 2, 2, 2, 3 ),
 ( 0.2083333333333333426, 0.2129629629629629650, 0.2222222222222222099, 0.2314814814814814825, 0.2361111111111111049 ),
 .UNSPECIFIED. ) 
 CURVE ( )  GEOMETRIC_REPRESENTATION_ITEM ( )  RATIONAL_B_SPLINE_CURVE ( ( 0.9330127018922194093, 0.9330127018922195203, 1.000000000000000000, 0.8660254037844387076, 1.000000000000000000, 0.8660254037844387076, 1.000000000000000000, 0.9330127018922194093, 0.9330127018922194093 ) ) 
 REPRESENTATION_ITEM ( '' )  );
#25517=CARTESIAN_POINT ( 'NONE',  ( -3.999940174399832848, 25.00001595349299421, 30.26464805816245729 ) ) ;
#25520=CARTESIAN_POINT ( 'NONE',  ( 3.756430356250000546, 12.79062499938548392, 27.83122392262697886 ) ) ;
#25533=CARTESIAN_POINT ( 'NONE',  ( -3.756430356250000102, 20.06562499938548072, 30.00000000000000000 ) ) ;
#25554=EDGE_CURVE ( 'NONE', #5101, #2103, #43266, .T. ) ;
#25567=CARTESIAN_POINT ( 'NONE',  ( 1.878215178124997609, 15.37812499938548427, 33.25316411605952993 ) ) ;
#25609=DIRECTION ( 'NONE',  ( 0.000000000000000000, 1.000000000000000000, 0.000000000000000000 ) ) ;
#25620=CARTESIAN_POINT ( 'NONE',  ( -1.243387493232115393E-14, 16.21250000000000213, 26.00000000000000000 ) ) ;
#25623=CARTESIAN_POINT ( 'NONE',  ( 1.878215178125000495, 13.16562499938548392, 26.74683588394047007 ) ) ;
#25626=ORIENTED_EDGE ( 'NONE', *, *, #26495, .T. ) ;
#25630=CARTESIAN_POINT ( 'NONE',  ( -1.878215178124999163, 18.64062499938548356, 26.74683588394047007 ) ) ;
#25639=CARTESIAN_POINT ( 'NONE',  ( 3.756430356250000546, 14.92812499938548321, 27.83122392262697886 ) ) ;
#25684=CARTESIAN_POINT ( 'NONE',  ( -4.000000000000000888, 18.61250000000000426, 32.30940107675850470 ) ) ;
#25685=EDGE_CURVE ( 'NONE', #72457, #29842, #45218, .T. ) ;
#25689=DIRECTION ( 'NONE',  ( 1.000000000000000000, 0.000000000000000000, 0.000000000000000000 ) ) ;
#25692=CARTESIAN_POINT ( 'NONE',  ( -3.756430356250000990, 20.66562499938548569, 32.16877607737301048 ) ) ;
#25724=AXIS2_PLACEMENT_3D ( 'NONE', #40058, #17139, #29325 ) ;
#25743=ORIENTED_EDGE ( 'NONE', *, *, #32902, .T. ) ;
#25803=CARTESIAN_POINT ( 'NONE',  ( 0.000000000000000000, 12.50000000000000000, 30.00000000000000000 ) ) ;
#25811=CARTESIAN_POINT ( 'NONE',  ( 2.655984681222220721E-16, 12.75312499938548427, 25.66244784525396483 ) ) ;
#25813=CARTESIAN_POINT ( 'NONE',  ( 3.999999999999998668, 15.16250000000000142, 32.30940107675850470 ) ) ;
#25818=CARTESIAN_POINT ( 'NONE',  ( -1.243387493232115393E-14, 16.15624999877096712, 26.00000000000000000 ) ) ;
#25894=CARTESIAN_POINT ( 'NONE',  ( -3.756430356250001434, 13.01562499938548534, 32.16877607737301048 ) ) ;
#25906=CARTESIAN_POINT ( 'NONE',  ( -1.878215178125001827, 19.69062499938548072, 33.25316411605952283 ) ) ;
#25936=CARTESIAN_POINT ( 'NONE',  ( 3.756430356250000102, 14.10312499938548392, 30.00000000000000000 ) ) ;
#25975=EDGE_CURVE ( 'NONE', #60301, #38096, #20142, .T. ) ;
#25990=CARTESIAN_POINT ( 'NONE',  ( -2.000000000000001776, 14.15000000000000036, 33.46410161513775705 ) ) ;
#25997=CARTESIAN_POINT ( 'NONE',  ( 0.6522972858965978560, 20.64114861271052348, 33.69936173848522998 ) ) ;
#26006=CARTESIAN_POINT ( 'NONE',  ( 3.756430356249998770, 15.75312499938548427, 32.16877607737302469 ) ) ;
#26021=CARTESIAN_POINT ( 'NONE',  ( -2.000000000000001776, 16.34374999877096712, 33.46410161513775705 ) ) ;
#26025=ORIENTED_EDGE ( 'NONE', *, *, #65868, .T. ) ;
#26051=CARTESIAN_POINT ( 'NONE',  ( -1.071796769724490783, 12.81740381056766864, 34.00000000000000711 ) ) ;
#26054=CARTESIAN_POINT ( 'NONE',  ( -3.756430356250000990, 19.76562499938548356, 32.16877607737301048 ) ) ;
#26071=ORIENTED_EDGE ( 'NONE', *, *, #57999, .T. ) ;
#26083=ORIENTED_EDGE ( 'NONE', *, *, #72649, .F. ) ;
#26086=CARTESIAN_POINT ( 'NONE',  ( 4.898587196589412829E-16, 27.50000000000000000, 34.00000000000000000 ) ) ;
#26087=ADVANCED_FACE ( 'NONE', ( #44376 ), #54713, .T. ) ;
#26091=CARTESIAN_POINT ( 'NONE',  ( -1.071796769724490339, 17.97634618820330132, 26.00000000000000000 ) ) ;
#26108=CARTESIAN_POINT ( 'NONE',  ( -4.000000000000000888, 19.06250000000000000, 32.30940107675850470 ) ) ;
#26115=DIRECTION ( 'NONE',  ( -0.9848086006944722914, -4.896307315423231436E-06, 0.1736433700842670569 ) ) ;
#26135=CARTESIAN_POINT ( 'NONE',  ( 3.756430356250000102, 12.64062499938548356, 30.00000000000000000 ) ) ;
#26173=CARTESIAN_POINT ( 'NONE',  ( -3.756430356249999214, 12.82812499938548534, 27.83122392262697531 ) ) ;
#26175=CARTESIAN_POINT ( 'NONE',  ( 4.000000000000000000, 14.78750000000000142, 27.69059892324149530 ) ) ;
#26260=CARTESIAN_POINT ( 'NONE',  ( -3.756430356249999214, 14.74062499938548498, 27.83122392262697531 ) ) ;
#26271=CARTESIAN_POINT ( 'NONE',  ( -3.756430356249999214, 20.02812499938548285, 27.83122392262697176 ) ) ;
#26302=CARTESIAN_POINT ( 'NONE',  ( -3.756430356250000102, 14.32812499938548356, 30.00000000000000000 ) ) ;
#26372=CARTESIAN_POINT ( 'NONE',  ( -3.756430356249999214, 16.42812499938548143, 27.83122392262697531 ) ) ;
#26388=CARTESIAN_POINT ( 'NONE',  ( -2.000000000000001776, 16.79374999877096641, 33.46410161513775705 ) ) ;
#26421=CARTESIAN_POINT ( 'NONE',  ( -7.967954043666661671E-16, 20.29062499938548569, 34.33755215474603517 ) ) ;
#26458=CARTESIAN_POINT ( 'NONE',  ( -1.071796769724492115, 19.56740381056766509, 34.00000000000000000 ) ) ;
#26459=CARTESIAN_POINT ( 'NONE',  ( -1.626862140677534273E-15, 18.18124999877096215, 34.00000000000000000 ) ) ;
#26476=CARTESIAN_POINT ( 'NONE',  ( -1.999999999999999112, 18.95000000000000284, 26.53589838486224650 ) ) ;
#26495=EDGE_CURVE ( 'NONE', #43576, #12632, #40465, .T. ) ;
#26506=CARTESIAN_POINT ( 'NONE',  ( -3.756430356250001434, 13.35312499938548392, 32.16877607737301048 ) ) ;
#26513=EDGE_CURVE ( 'NONE', #29218, #71220, #68662, .T. ) ;
#26520=CARTESIAN_POINT ( 'NONE',  ( -4.000000000000000000, 16.77499999999999858, 30.00000000000000000 ) ) ;
#26544=CARTESIAN_POINT ( 'NONE',  ( 0.6522972858965978560, 20.75364861271052419, 33.69936173848522998 ) ) ;
#26546=CARTESIAN_POINT ( 'NONE',  ( 2.828200636599751609E-16, 15.76249999999999751, 25.38119784648299415 ) ) ;
#26597=DIRECTION ( 'NONE',  ( -0.000000000000000000, -1.000000000000000000, -0.000000000000000000 ) ) ;
#26624=CARTESIAN_POINT ( 'NONE',  ( -1.071796769724496334, 15.78259618943233455, 26.00000000000000355 ) ) ;
#26628=CARTESIAN_POINT ( 'NONE',  ( -1.626862140677534273E-15, 17.73124999877096641, 34.00000000000000000 ) ) ;
#26633=CARTESIAN_POINT ( 'NONE',  ( -1.878215178124999163, 13.35312499938548392, 26.74683588394047007 ) ) ;
#26642=CARTESIAN_POINT ( 'NONE',  ( 1.138803498474273873E-14, 16.38124999877096499, 34.00000000000000000 ) ) ;
#26656=CARTESIAN_POINT ( 'NONE',  ( 4.648177544792955741E-15, 14.58124999877096606, 33.99999999999999289 ) ) ;
#26678=CARTESIAN_POINT ( 'NONE',  ( 3.756430356250000102, 15.45312499938548356, 30.00000000000000000 ) ) ;
#26730=CARTESIAN_POINT ( 'NONE',  ( 3.756430356250000546, 15.37812499938548427, 27.83122392262697886 ) ) ;
#26737=CARTESIAN_POINT ( 'NONE',  ( -3.756430356250000102, 19.61562499938548143, 30.00000000000000000 ) ) ;
#26747=CARTESIAN_POINT ( 'NONE',  ( -1.878215178124999163, 19.54062499938548214, 26.74683588394047007 ) ) ;
#26763=CARTESIAN_POINT ( 'NONE',  ( -4.000000000000000000, 15.36874999877096570, 30.00000000000000000 ) ) ;
#26772=CARTESIAN_POINT ( 'NONE',  ( -1.999999999999999112, 16.19374999877096499, 26.53589838486224650 ) ) ;
#26794=CARTESIAN_POINT ( 'NONE',  ( 1.878215178125000495, 19.12812499938548427, 26.74683588394047007 ) ) ;
#26804=CARTESIAN_POINT ( 'NONE',  ( 0.000000000000000000, 27.50000000000000000, 26.00000000000000000 ) ) ;
#26810=( BOUNDED_CURVE ( )  B_SPLINE_CURVE ( 2, ( #33757, #56653, #45583, #11951, #17831, #34476, #57004, #40392, #1241 ),
 .UNSPECIFIED., .F., .F. ) 
 B_SPLINE_CURVE_WITH_KNOTS ( ( 3, 2, 2, 2, 3 ),
 ( 0.4305555555555555802, 0.4351851851851851749, 0.4444444444444444198, 0.4537037037037037202, 0.4583333333333333703 ),
 .UNSPECIFIED. ) 
 CURVE ( )  GEOMETRIC_REPRESENTATION_ITEM ( )  RATIONAL_B_SPLINE_CURVE ( ( 0.9330127018922194093, 0.9330127018922197424, 1.000000000000000000, 0.8660254037844387076, 1.000000000000000000, 0.8660254037844387076, 1.000000000000000000, 0.9330127018922189652, 0.9330127018922194093 ) ) 
 REPRESENTATION_ITEM ( '' )  );
#26827=CARTESIAN_POINT ( 'NONE',  ( -1.999999999999999112, 14.84374999877096712, 26.53589838486224650 ) ) ;
#26879=CARTESIAN_POINT ( 'NONE',  ( -7.967954043666661671E-16, 13.42812499938548321, 34.33755215474603517 ) ) ;
#26885=CARTESIAN_POINT ( 'NONE',  ( -2.498395430326213790E-14, 20.26249999999999929, 26.00000000000000000 ) ) ;
#26918=CARTESIAN_POINT ( 'NONE',  ( -7.967954043666661671E-16, 15.22812499938548214, 34.33755215474603517 ) ) ;
#26920=CARTESIAN_POINT ( 'NONE',  ( 1.999999999999997335, 16.92500000000000071, 33.46410161513775705 ) ) ;
#26971=EDGE_CURVE ( 'NONE', #49631, #9585, #60794, .T. ) ;
#26993=CARTESIAN_POINT ( 'NONE',  ( -1.999999999999999112, 15.80000000000000071, 26.53589838486224650 ) ) ;
#27001=CARTESIAN_POINT ( 'NONE',  ( -3.756430356250001434, 14.81562499938548250, 32.16877607737301048 ) ) ;
#27043=CARTESIAN_POINT ( 'NONE',  ( -1.878215178124999163, 16.05312499938548143, 26.74683588394047007 ) ) ;
#27096=CARTESIAN_POINT ( 'NONE',  ( 3.756430356249998770, 15.75312499938548427, 32.16877607737301759 ) ) ;
#27102=CARTESIAN_POINT ( 'NONE',  ( 1.878215178124997609, 19.76562499938548356, 33.25316411605952993 ) ) ;
#27111=CARTESIAN_POINT ( 'NONE',  ( 1.878215178124997609, 17.51562499938548356, 33.25316411605952993 ) ) ;
#27126=CARTESIAN_POINT ( 'NONE',  ( 4.000000000000000000, 16.53124999877096712, 27.69059892324149530 ) ) ;
#27129=CARTESIAN_POINT ( 'NONE',  ( -1.626862140677534273E-15, 17.73124999877096641, 34.00000000000000000 ) ) ;
#27170=CARTESIAN_POINT ( 'NONE',  ( 0.000000000000000000, 27.50000000000000000, 26.00000000000000000 ) ) ;
#27178=CARTESIAN_POINT ( 'NONE',  ( -1.626862140677534273E-15, 19.13749999999999929, 34.00000000000000000 ) ) ;
#27236=EDGE_CURVE ( 'NONE', #50521, #59214, #35271, .T. ) ;
#27239=CARTESIAN_POINT ( 'NONE',  ( 2.655984681222220721E-16, 13.20312499938548534, 25.66244784525396483 ) ) ;
#27243=ADVANCED_FACE ( 'NONE', ( #22162 ), #32159, .T. ) ;
#27250=CARTESIAN_POINT ( 'NONE',  ( -3.756430356249999214, 15.19062499938548427, 27.83122392262697176 ) ) ;
#27263=VERTEX_POINT ( 'NONE', #16608 ) ;
#27278=CARTESIAN_POINT ( 'NONE',  ( -1.878215178125001827, 13.84062499938548285, 33.25316411605952283 ) ) ;
#27280=CARTESIAN_POINT ( 'NONE',  ( 2.000000000000000444, 16.62500000000000000, 26.53589838486224650 ) ) ;
#27292=ORIENTED_EDGE ( 'NONE', *, *, #26513, .T. ) ;
#27298=CARTESIAN_POINT ( 'NONE',  ( 4.000000000000000000, 20.09374999877096712, 30.00000000000000000 ) ) ;
#27323=ORIENTED_EDGE ( 'NONE', *, *, #39141, .F. ) ;
#27325=CARTESIAN_POINT ( 'NONE',  ( -4.000000000000000000, 13.11874999877096570, 30.00000000000000000 ) ) ;
#27356=CARTESIAN_POINT ( 'NONE',  ( 1.999999999999997335, 17.76874999877096428, 33.46410161513775705 ) ) ;
#27361=CARTESIAN_POINT ( 'NONE',  ( 1.878215178125000495, 16.42812499938548143, 26.74683588394047007 ) ) ;
#27370=CARTESIAN_POINT ( 'NONE',  ( 4.000000000000000000, 16.53124999877096712, 27.69059892324149885 ) ) ;
#27405=CARTESIAN_POINT ( 'NONE',  ( -3.756430356250000102, 18.37812499938548427, 30.00000000000000000 ) ) ;
#27422=CYLINDRICAL_SURFACE ( 'NONE', #14924, 4.000000000000000000 ) ;
#27449=CYLINDRICAL_SURFACE ( 'NONE', #18356, 4.000000000000000000 ) ;
#27451=ORIENTED_EDGE ( 'NONE', *, *, #2787, .T. ) ;
#27461=CARTESIAN_POINT ( 'NONE',  ( 1.878215178125000495, 15.86562499938548321, 26.74683588394047007 ) ) ;
#27476=CARTESIAN_POINT ( 'NONE',  ( 1.878215178125000495, 18.56562499938548427, 26.74683588394047007 ) ) ;
#27490=CARTESIAN_POINT ( 'NONE',  ( -4.000000000000000888, 19.00624999877096499, 32.30940107675850470 ) ) ;
#27522=FACE_OUTER_BOUND ( 'NONE', #50737, .T. ) ;
#27542=VERTEX_POINT ( 'NONE', #9544 ) ;
#27593=ORIENTED_EDGE ( 'NONE', *, *, #41247, .T. ) ;
#27605=CARTESIAN_POINT ( 'NONE',  ( -3.756430356250000102, 13.31562499938548427, 30.00000000000000000 ) ) ;
#27612=CARTESIAN_POINT ( 'NONE',  ( 3.756430356250000546, 13.69062499938548250, 27.83122392262697886 ) ) ;
#27632=CARTESIAN_POINT ( 'NONE',  ( 3.999999999999998668, 19.66249999999999787, 32.30940107675850470 ) ) ;
#27639=CARTESIAN_POINT ( 'NONE',  ( -1.878215178125001827, 15.64062499938548356, 33.25316411605952283 ) ) ;
#27642=CARTESIAN_POINT ( 'NONE',  ( -3.999999999999999556, 17.63749999999999929, 27.69059892324149175 ) ) ;
#27718=AXIS2_PLACEMENT_3D ( 'NONE', #58655, #52764, #8790 ) ;
#27725=CARTESIAN_POINT ( 'NONE',  ( 3.756430356249998770, 14.96562499938548108, 32.16877607737302469 ) ) ;
#27769=CARTESIAN_POINT ( 'NONE',  ( -1.878215178124999163, 17.40312499938548285, 26.74683588394047007 ) ) ;
#27829=CARTESIAN_POINT ( 'NONE',  ( -3.756430356250000990, 14.25312499938548250, 32.16877607737301048 ) ) ;
#27846=CARTESIAN_POINT ( 'NONE',  ( 3.756430356250000546, 18.07812499938548711, 27.83122392262697886 ) ) ;
#27860=CARTESIAN_POINT ( 'NONE',  ( -3.999999999999999556, 18.48124999877096997, 27.69059892324149175 ) ) ;
#27890=CARTESIAN_POINT ( 'NONE',  ( -2.000000000000001776, 14.59999999999999964, 33.46410161513775705 ) ) ;
#27979=CARTESIAN_POINT ( 'NONE',  ( 3.756430356250000102, 14.10312499938548392, 30.00000000000000000 ) ) ;
#27980=CARTESIAN_POINT ( 'NONE',  ( -4.000000000000000000, 15.36874999877096570, 30.00000000000000000 ) ) ;
#28011=CARTESIAN_POINT ( 'NONE',  ( -2.000000000000001776, 18.19999999999999929, 33.46410161513775705 ) ) ;
#28043=ORIENTED_EDGE ( 'NONE', *, *, #25975, .F. ) ;
#28091=CARTESIAN_POINT ( 'NONE',  ( 1.878215178125000495, 15.97812499938548392, 26.74683588394047007 ) ) ;
#28097=CARTESIAN_POINT ( 'NONE',  ( 0.000000000000000000, 27.50000000000000000, 26.00000000000000000 ) ) ;
#28134=CARTESIAN_POINT ( 'NONE',  ( -1.878215178125001827, 17.55312499938548498, 33.25316411605952283 ) ) ;
#28173=CARTESIAN_POINT ( 'NONE',  ( -1.999999999999999112, 15.74374999877096570, 26.53589838486224650 ) ) ;
#28188=CARTESIAN_POINT ( 'NONE',  ( 3.756430356249998770, 15.30312499938548321, 32.16877607737301759 ) ) ;
#28204=CARTESIAN_POINT ( 'NONE',  ( -3.756430356250001434, 18.75312499938548427, 32.16877607737301048 ) ) ;
#28218=CARTESIAN_POINT ( 'NONE',  ( 4.000000000000000000, 19.19374999877096499, 30.00000000000000000 ) ) ;
#28243=DIRECTION ( 'NONE',  ( 0.000000000000000000, 0.000000000000000000, -1.000000000000000000 ) ) ;
#28248=CARTESIAN_POINT ( 'NONE',  ( 0.000000000000000000, 27.50000000000000000, 26.00000000000000000 ) ) ;
#28257=DIRECTION ( 'NONE',  ( 0.000000000000000000, 0.000000000000000000, -1.000000000000000000 ) ) ;
#28319=( BOUNDED_CURVE ( )  B_SPLINE_CURVE ( 2, ( #11420, #21762, #39869, #33219, #17661, #44323, #67935, #61650, #33577 ),
 .UNSPECIFIED., .F., .F. ) 
 B_SPLINE_CURVE_WITH_KNOTS ( ( 3, 2, 2, 2, 3 ),
 ( 0.9027777777777777901, 0.9074074074074074403, 0.9166666666666666297, 0.9259259259259259300, 0.9305555555555555802 ),
 .UNSPECIFIED. ) 
 CURVE ( )  GEOMETRIC_REPRESENTATION_ITEM ( )  RATIONAL_B_SPLINE_CURVE ( ( 0.9330127018922194093, 0.9330127018922194093, 1.000000000000000000, 0.8660254037844387076, 1.000000000000000000, 0.8660254037844387076, 1.000000000000000000, 0.9330127018922194093, 0.9330127018922194093 ) ) 
 REPRESENTATION_ITEM ( '' )  );
#28328=CARTESIAN_POINT ( 'NONE',  ( 1.878215178124997609, 14.47812499938548214, 33.25316411605952993 ) ) ;
#28334=CARTESIAN_POINT ( 'NONE',  ( 4.898587196589412829E-16, 27.50000000000000000, 34.00000000000000000 ) ) ;
#28354=ORIENTED_EDGE ( 'NONE', *, *, #60834, .F. ) ;
#28360=CARTESIAN_POINT ( 'NONE',  ( 4.000000000000000000, 17.44999999999999929, 30.00000000000000000 ) ) ;
#28424=AXIS2_PLACEMENT_3D ( 'NONE', #25803, #71602, #48341 ) ;
#28437=DIRECTION ( 'NONE',  ( 0.000000000000000000, 0.000000000000000000, 1.000000000000000000 ) ) ;
#28442=CARTESIAN_POINT ( 'NONE',  ( 3.756430356249998770, 15.86562499938548321, 32.16877607737302469 ) ) ;
#28483=CARTESIAN_POINT ( 'NONE',  ( -3.756430356250000102, 17.47812499938548214, 30.00000000000000000 ) ) ;
#28541=CARTESIAN_POINT ( 'NONE',  ( -3.756430356250000990, 16.95312499938548356, 32.16877607737301048 ) ) ;
#28566=CARTESIAN_POINT ( 'NONE',  ( -2.498395430326213790E-14, 17.05624999877096926, 26.00000000000000000 ) ) ;
#28572=CARTESIAN_POINT ( 'NONE',  ( -8.484601909799255319E-16, 17.73124999877096641, 34.61880215351700940 ) ) ;
#28623=ORIENTED_EDGE ( 'NONE', *, *, #40237, .T. ) ;
#28631=VERTEX_POINT ( 'NONE', #17971 ) ;
#28653=( NAMED_UNIT ( * ) PLANE_ANGLE_UNIT ( ) SI_UNIT ( $, .RADIAN. ) );
#28682=CARTESIAN_POINT ( 'NONE',  ( 3.999999999999998668, 13.81250000000000000, 32.30940107675850470 ) ) ;
#28688=CARTESIAN_POINT ( 'NONE',  ( 1.878215178125000495, 13.72812499938548392, 26.74683588394047007 ) ) ;
#28702=EDGE_LOOP ( 'NONE', ( #47065, #53365, #32443, #43587 ) ) ;
#28719=CARTESIAN_POINT ( 'NONE',  ( -8.484601909799255319E-16, 19.13750000000000284, 34.61880215351700940 ) ) ;
#28761=EDGE_CURVE ( 'NONE', #53784, #58713, #24252, .T. ) ;
#28800=CARTESIAN_POINT ( 'NONE',  ( -1.878215178124999163, 17.85312499938548214, 26.74683588394047007 ) ) ;
#28811=CARTESIAN_POINT ( 'NONE',  ( -4.000000000000000888, 16.36250000000000071, 32.30940107675850470 ) ) ;
#28842=CARTESIAN_POINT ( 'NONE',  ( -7.967954043666661671E-16, 18.49062499938548143, 34.33755215474603517 ) ) ;
#28888=ORIENTED_EDGE ( 'NONE', *, *, #34930, .T. ) ;
#28899=CARTESIAN_POINT ( 'NONE',  ( 2.655984681222220721E-16, 16.35312499938548569, 25.66244784525396483 ) ) ;
#28933=CARTESIAN_POINT ( 'NONE',  ( 1.999999999999997335, 18.66874999877096641, 33.46410161513775705 ) ) ;
#28992=CARTESIAN_POINT ( 'NONE',  ( -1.071796769724502107, 18.87634618820330346, 26.00000000000000711 ) ) ;
#28996=CARTESIAN_POINT ( 'NONE',  ( -3.756430356250001434, 14.70312499938548179, 32.16877607737301048 ) ) ;
#28998=ORIENTED_EDGE ( 'NONE', *, *, #23453, .T. ) ;
#29058=CARTESIAN_POINT ( 'NONE',  ( 3.756430356250000546, 17.74062499938548498, 27.83122392262697886 ) ) ;
#29062=CARTESIAN_POINT ( 'NONE',  ( 0.6522972858965978560, 20.64114861271052348, 33.69936173848522998 ) ) ;
#29068=ORIENTED_EDGE ( 'NONE', *, *, #22509, .T. ) ;
#29090=CARTESIAN_POINT ( 'NONE',  ( -3.999999999999999556, 19.88749999999999929, 27.69059892324149175 ) ) ;
#29110=LINE ( 'NONE', #63800, #66939 ) ;
#29128=DIRECTION ( 'NONE',  ( -0.000000000000000000, -1.000000000000000000, -0.000000000000000000 ) ) ;
#29171=CARTESIAN_POINT ( 'NONE',  ( -1.878215178125001827, 18.45312499938548356, 33.25316411605952283 ) ) ;
#29173=CARTESIAN_POINT ( 'NONE',  ( 2.000000000000000444, 13.47500000000000142, 26.53589838486224650 ) ) ;
#29209=CARTESIAN_POINT ( 'NONE',  ( 3.756430356249998770, 20.36562499938548143, 32.16877607737302469 ) ) ;
#29218=VERTEX_POINT ( 'NONE', #68468 ) ;
#29242=( BOUNDED_CURVE ( )  B_SPLINE_CURVE ( 2, ( #27178, #54881, #49712, #4287, #71878, #21251, #43804, #11641, #1282 ),
 .UNSPECIFIED., .F., .F. ) 
 B_SPLINE_CURVE_WITH_KNOTS ( ( 3, 2, 2, 2, 3 ),
 ( 0.8194444444444444198, 0.8240740740740740700, 0.8333333333333333703, 0.8425925925925925597, 0.8472222222222222099 ),
 .UNSPECIFIED. ) 
 CURVE ( )  GEOMETRIC_REPRESENTATION_ITEM ( )  RATIONAL_B_SPLINE_CURVE ( ( 0.9330127018922194093, 0.9330127018922194093, 1.000000000000000000, 0.8660254037844387076, 1.000000000000000000, 0.8660254037844387076, 1.000000000000000000, 0.9330127018922194093, 0.9330127018922194093 ) ) 
 REPRESENTATION_ITEM ( '' )  );
#29268=CARTESIAN_POINT ( 'NONE',  ( -3.756430356249999214, 17.32812499938548356, 27.83122392262697176 ) ) ;
#29297=CARTESIAN_POINT ( 'NONE',  ( -3.756430356249999214, 13.39062499938548179, 27.83122392262697531 ) ) ;
#29325=DIRECTION ( 'NONE',  ( 0.000000000000000000, 0.000000000000000000, 1.000000000000000000 ) ) ;
#29358=CARTESIAN_POINT ( 'NONE',  ( -7.967954043666661671E-16, 16.12812499938548427, 34.33755215474603517 ) ) ;
#29388=CARTESIAN_POINT ( 'NONE',  ( 1.626862140677534470E-15, 13.68124999877096748, 34.00000000000000000 ) ) ;
#29408=EDGE_CURVE ( 'NONE', #16877, #57346, #10057, .T. ) ;
#29419=CARTESIAN_POINT ( 'NONE',  ( -3.756430356249999214, 17.89062499938548356, 27.83122392262697176 ) ) ;
#29448=CARTESIAN_POINT ( 'NONE',  ( -3.999999999999999556, 19.43750000000000000, 27.69059892324149175 ) ) ;
#29459=( BOUNDED_CURVE ( )  B_SPLINE_CURVE ( 2, ( #30367, #2655, #66081, #65715, #15101, #54634, #7465, #64338, #24084 ),
 .UNSPECIFIED., .F., .F. ) 
 B_SPLINE_CURVE_WITH_KNOTS ( ( 3, 2, 2, 2, 3 ),
 ( 0.3472222222222222654, 0.3518518518518518601, 0.3611111111111111049, 0.3703703703703703498, 0.3750000000000000000 ),
 .UNSPECIFIED. ) 
 CURVE ( )  GEOMETRIC_REPRESENTATION_ITEM ( )  RATIONAL_B_SPLINE_CURVE ( ( 0.9330127018922194093, 0.9330127018922197424, 1.000000000000000000, 0.8660254037844387076, 1.000000000000000000, 0.8660254037844387076, 1.000000000000000000, 0.9330127018922194093, 0.9330127018922194093 ) ) 
 REPRESENTATION_ITEM ( '' )  );
#29463=ORIENTED_EDGE ( 'NONE', *, *, #40217, .F. ) ;
#29513=CARTESIAN_POINT ( 'NONE',  ( 0.000000000000000000, 25.54316770519903557, 26.00000000000000000 ) ) ;
#29530=CARTESIAN_POINT ( 'NONE',  ( 2.655984681222220721E-16, 18.26562499938548356, 25.66244784525396483 ) ) ;
#29532=CARTESIAN_POINT ( 'NONE',  ( -1.999999999999999112, 12.65000000000000213, 26.53589838486224650 ) ) ;
#29539=CARTESIAN_POINT ( 'NONE',  ( -4.000000000000000000, 19.47499999999999787, 30.00000000000000000 ) ) ;
#29564=VERTEX_POINT ( 'NONE', #22526 ) ;
#29567=CARTESIAN_POINT ( 'NONE',  ( -1.878215178124999163, 19.20312499938548356, 26.74683588394047007 ) ) ;
#29568=ADVANCED_FACE ( 'NONE', ( #50260 ), #6268, .T. ) ;
#29607=CARTESIAN_POINT ( 'NONE',  ( -2.000000000000001776, 15.89374999877096784, 33.46410161513775705 ) ) ;
#29612=ORIENTED_EDGE ( 'NONE', *, *, #24336, .T. ) ;
#29623=CARTESIAN_POINT ( 'NONE',  ( -3.756430356249999214, 17.77812499938548285, 27.83122392262697176 ) ) ;
#29652=CARTESIAN_POINT ( 'NONE',  ( 2.000000000000000444, 19.71874999877096712, 26.53589838486224650 ) ) ;
#29678=CARTESIAN_POINT ( 'NONE',  ( -4.000000000000000000, 14.46874999877096712, 30.00000000000000000 ) ) ;
#29700=ORIENTED_EDGE ( 'NONE', *, *, #23453, .F. ) ;
#29708=CARTESIAN_POINT ( 'NONE',  ( -1.999999999999999112, 18.89374999877096784, 26.53589838486224650 ) ) ;
#29713=CARTESIAN_POINT ( 'NONE',  ( 3.756430356250000102, 16.24062499938548143, 30.00000000000000000 ) ) ;
#29715=VERTEX_POINT ( 'NONE', #35012 ) ;
#29739=CARTESIAN_POINT ( 'NONE',  ( 0.000000000000000000, 27.50000000000000000, 30.00000000000000000 ) ) ;
#29773=CARTESIAN_POINT ( 'NONE',  ( 3.756430356250000546, 17.29062499938548214, 27.83122392262697886 ) ) ;
#29801=VERTEX_POINT ( 'NONE', #1412 ) ;
#29808=CARTESIAN_POINT ( 'NONE',  ( 4.000000000000000000, 18.83749999999999858, 27.69059892324149530 ) ) ;
#29842=VERTEX_POINT ( 'NONE', #51649 ) ;
#29845=CARTESIAN_POINT ( 'NONE',  ( 3.999999999999998668, 14.26250000000000107, 32.30940107675850470 ) ) ;
#29870=CARTESIAN_POINT ( 'NONE',  ( 3.974238962994274260, 25.00693170370651686, 29.47568919947315180 ) ) ;
#29887=CARTESIAN_POINT ( 'NONE',  ( 1.878215178124997609, 17.62812499938548427, 33.25316411605952993 ) ) ;
#29889=CARTESIAN_POINT ( 'NONE',  ( 1.999999999999997335, 12.87500000000000178, 33.46410161513775705 ) ) ;
#29926=CARTESIAN_POINT ( 'NONE',  ( -1.878215178124999163, 19.65312499938548285, 26.74683588394047007 ) ) ;
#29935=ORIENTED_EDGE ( 'NONE', *, *, #41750, .T. ) ;
#29963=CARTESIAN_POINT ( 'NONE',  ( -0.5230845267916411911, 25.53603409863758955, 33.97449076415956171 ) ) ;
#29980=CARTESIAN_POINT ( 'NONE',  ( -3.756430356249999214, 18.22812499938548214, 27.83122392262697176 ) ) ;
#29987=DIRECTION ( 'NONE',  ( -0.000000000000000000, -1.000000000000000000, -0.000000000000000000 ) ) ;
#30001=CARTESIAN_POINT ( 'NONE',  ( 1.071796769724500997, 18.65134618820329848, 33.99999999999999289 ) ) ;
#30006=ORIENTED_EDGE ( 'NONE', *, *, #45894, .T. ) ;
#30010=CARTESIAN_POINT ( 'NONE',  ( -1.878215178124999163, 13.35312499938548392, 26.74683588394047007 ) ) ;
#30036=CARTESIAN_POINT ( 'NONE',  ( -2.000000000000001776, 13.25000000000000178, 33.46410161513775705 ) ) ;
#30040=ADVANCED_FACE ( 'NONE', ( #31291 ), #65636, .T. ) ;
#30075=CARTESIAN_POINT ( 'NONE',  ( 3.756430356250000546, 16.72812499938548214, 27.83122392262697886 ) ) ;
#30077=ORIENTED_EDGE ( 'NONE', *, *, #54489, .T. ) ;
#30101=CARTESIAN_POINT ( 'NONE',  ( 2.828200636599751609E-16, 13.00624999877096677, 25.38119784648299415 ) ) ;
#30116=VECTOR ( 'NONE', #31365, 1000.000000000000000 ) ;
#30137=CARTESIAN_POINT ( 'NONE',  ( -7.967954043666661671E-16, 17.14062499938548356, 34.33755215474603517 ) ) ;
#30191=CARTESIAN_POINT ( 'NONE',  ( -1.626862140677534273E-15, 19.53124999877096357, 34.00000000000000000 ) ) ;
#30218=CARTESIAN_POINT ( 'NONE',  ( 3.756430356250000546, 12.67812499938548143, 27.83122392262697886 ) ) ;
#30254=CARTESIAN_POINT ( 'NONE',  ( 3.756430356250000546, 19.54062499938548214, 27.83122392262697886 ) ) ;
#30256=CARTESIAN_POINT ( 'NONE',  ( 1.878215178124997609, 20.21562499938548285, 33.25316411605952993 ) ) ;
#30285=ADVANCED_BREP_SHAPE_REPRESENTATION ( '', ( #20659, #23765 ), #24934 ) ;
#30295=CARTESIAN_POINT ( 'NONE',  ( -7.967954043666661671E-16, 19.84062499938548285, 34.33755215474603517 ) ) ;
#30314=( BOUNDED_CURVE ( )  B_SPLINE_CURVE ( 2, ( #57906, #35024, #7315, #29845, #69385, #1424, #35383, #68295, #23573 ),
 .UNSPECIFIED., .F., .F. ) 
 B_SPLINE_CURVE_WITH_KNOTS ( ( 3, 2, 2, 2, 3 ),
 ( 0.2083333333333333426, 0.2129629629629629650, 0.2222222222222222099, 0.2314814814814814825, 0.2361111111111111049 ),
 .UNSPECIFIED. ) 
 CURVE ( )  GEOMETRIC_REPRESENTATION_ITEM ( )  RATIONAL_B_SPLINE_CURVE ( ( 0.9330127018922194093, 0.9330127018922195203, 1.000000000000000000, 0.8660254037844387076, 1.000000000000000000, 0.8660254037844387076, 1.000000000000000000, 0.9330127018922194093, 0.9330127018922194093 ) ) 
 REPRESENTATION_ITEM ( '' )  );
#30338=CARTESIAN_POINT ( 'NONE',  ( -0.2655188809381071047, 25.54316770519904267, 26.00000000000000355 ) ) ;
#30353=CARTESIAN_POINT ( 'NONE',  ( 3.756430356250000102, 20.29062499938548569, 30.00000000000000000 ) ) ;
#30367=CARTESIAN_POINT ( 'NONE',  ( -1.243387493232115393E-14, 15.31250000000000000, 26.00000000000000000 ) ) ;
#30384=CARTESIAN_POINT ( 'NONE',  ( -3.756430356250001434, 13.46562499938548285, 32.16877607737301048 ) ) ;
#30437=CARTESIAN_POINT ( 'NONE',  ( 5.000000000000000000, 39.99999999999999289, 45.00000000000000000 ) ) ;
#30445=CARTESIAN_POINT ( 'NONE',  ( -1.878215178124999163, 18.19062499938548427, 26.74683588394047007 ) ) ;
#30455=CARTESIAN_POINT ( 'NONE',  ( 1.878215178125000495, 17.21562499938548285, 26.74683588394047007 ) ) ;
#30462=CARTESIAN_POINT ( 'NONE',  ( -3.999999999999999112, 14.93750000000000355, 27.69059892324149530 ) ) ;
#30469=CYLINDRICAL_SURFACE ( 'NONE', #68202, 4.000000000000000000 ) ;
#30472=CARTESIAN_POINT ( 'NONE',  ( 1.999999999999997335, 19.11874999877096570, 33.46410161513775705 ) ) ;
#30502=CARTESIAN_POINT ( 'NONE',  ( 2.655984681222220721E-16, 16.91562499938548214, 25.66244784525396483 ) ) ;
#30512=LINE ( 'NONE', #64116, #53656 ) ;
#30551=ADVANCED_FACE ( 'NONE', ( #52294 ), #1695, .F. ) ;
#30554=ORIENTED_EDGE ( 'NONE', *, *, #60483, .T. ) ;
#30562=CARTESIAN_POINT ( 'NONE',  ( 0.6522972858965978560, 20.64114861271052348, 33.69936173848522998 ) ) ;
#30584=CARTESIAN_POINT ( 'NONE',  ( -3.756430356249999214, 12.82812499938548534, 27.83122392262697531 ) ) ;
#30616=CARTESIAN_POINT ( 'NONE',  ( -1.878215178124999163, 20.10312499938548569, 26.74683588394047007 ) ) ;
#30618=CARTESIAN_POINT ( 'NONE',  ( 2.750808005852812599, 20.68304698139313658, 33.32934212547041142 ) ) ;
#30628=CYLINDRICAL_SURFACE ( 'NONE', #51316, 15.00000000000000000 ) ;
#30629=EDGE_LOOP ( 'NONE', ( #6752, #48827, #30006, #13414 ) ) ;
#30655=CARTESIAN_POINT ( 'NONE',  ( 3.756430356250000546, 19.09062499938548640, 27.83122392262697886 ) ) ;
#30693=CARTESIAN_POINT ( 'NONE',  ( -2.007927870956448313, 25.40597574392634428, 26.53059533024969241 ) ) ;
#30708=CARTESIAN_POINT ( 'NONE',  ( 1.878215178125000495, 18.56562499938548427, 26.74683588394047007 ) ) ;
#30741=CARTESIAN_POINT ( 'NONE',  ( -4.000000000000000000, 20.31874999877096499, 30.00000000000000000 ) ) ;
#30749=CARTESIAN_POINT ( 'NONE',  ( 1.999999999999997335, 18.72499999999999787, 33.46410161513775705 ) ) ;
#30797=CARTESIAN_POINT ( 'NONE',  ( -2.000000000000001776, 16.79374999877096641, 33.46410161513775705 ) ) ;
#30804=CARTESIAN_POINT ( 'NONE',  ( 3.756430356250000546, 17.62812499938548427, 27.83122392262697886 ) ) ;
#30813=CARTESIAN_POINT ( 'NONE',  ( 2.655984681222220721E-16, 15.00312499938548427, 25.66244784525396483 ) ) ;
#30828=CARTESIAN_POINT ( 'NONE',  ( 4.000000000000000000, 13.34374999877096712, 30.00000000000000000 ) ) ;
#30859=CARTESIAN_POINT ( 'NONE',  ( 1.878215178125000495, 18.67812499938548143, 26.74683588394047007 ) ) ;
#30875=CARTESIAN_POINT ( 'NONE',  ( 0.6945846161026939525, 20.50052346155192495, 33.93923243933046763 ) ) ;
#30946=( BOUNDED_CURVE ( )  B_SPLINE_CURVE ( 2, ( #46315, #62573, #11969, #40411, #22682, #34493, #534, #6427, #68486 ),
 .UNSPECIFIED., .F., .F. ) 
 B_SPLINE_CURVE_WITH_KNOTS ( ( 3, 2, 2, 2, 3 ),
 ( 0.2638888888888888951, 0.2685185185185185452, 0.2777777777777777901, 0.2870370370370370350, 0.2916666666666666852 ),
 .UNSPECIFIED. ) 
 CURVE ( )  GEOMETRIC_REPRESENTATION_ITEM ( )  RATIONAL_B_SPLINE_CURVE ( ( 0.9330127018922194093, 0.9330127018922194093, 1.000000000000000000, 0.8660254037844387076, 1.000000000000000000, 0.8660254037844387076, 1.000000000000000000, 0.9330127018922189652, 0.9330127018922194093 ) ) 
 REPRESENTATION_ITEM ( '' )  );
#30961=CARTESIAN_POINT ( 'NONE',  ( 1.294081214890646203, 25.48735787228381255, 26.20605842228508564 ) ) ;
#30981=CARTESIAN_POINT ( 'NONE',  ( 2.655984681222220721E-16, 20.06562499938548427, 25.66244784525396483 ) ) ;
#30983=CARTESIAN_POINT ( 'NONE',  ( -2.000000000000001776, 14.59999999999999964, 33.46410161513775705 ) ) ;
#31016=CARTESIAN_POINT ( 'NONE',  ( -4.000000000000000888, 17.71249999999999858, 32.30940107675850470 ) ) ;
#31043=ORIENTED_EDGE ( 'NONE', *, *, #58697, .F. ) ;
#31057=CARTESIAN_POINT ( 'NONE',  ( -3.870849190549275232, 25.03400442039527007, 31.04151046405775105 ) ) ;
#31060=FACE_OUTER_BOUND ( 'NONE', #30629, .T. ) ;
#31073=CARTESIAN_POINT ( 'NONE',  ( -1.878215178124999163, 19.09062499938548285, 26.74683588394047007 ) ) ;
#31092=ORIENTED_EDGE ( 'NONE', *, *, #10308, .F. ) ;
#31093=CARTESIAN_POINT ( 'NONE',  ( 0.000000000000000000, 12.50000000000000000, 26.00000000000000000 ) ) ;
#31104=CARTESIAN_POINT ( 'NONE',  ( 1.878215178125000495, 15.07812499938548179, 26.74683588394047007 ) ) ;
#31130=CARTESIAN_POINT ( 'NONE',  ( 3.999999999999998668, 16.00624999877096499, 32.30940107675850470 ) ) ;
#31133=CARTESIAN_POINT ( 'NONE',  ( -3.486133158594716510E-16, 13.00624999877096855, 26.00000000000000355 ) ) ;
#31159=CARTESIAN_POINT ( 'NONE',  ( 3.756430356250000546, 13.12812499938548427, 27.83122392262697886 ) ) ;
#31166=CARTESIAN_POINT ( 'NONE',  ( 1.878215178124997609, 18.41562499938548214, 33.25316411605952993 ) ) ;
#31175=CARTESIAN_POINT ( 'NONE',  ( 1.878215178124997609, 16.16562499938548569, 33.25316411605952993 ) ) ;
#31193=CARTESIAN_POINT ( 'NONE',  ( -2.000000000000001776, 14.09374999877096535, 33.46410161513775705 ) ) ;
#31218=CARTESIAN_POINT ( 'NONE',  ( -3.999999999999999112, 18.53749999999999432, 27.69059892324149530 ) ) ;
#31226=CARTESIAN_POINT ( 'NONE',  ( 1.878215178124997609, 18.52812499938548285, 33.25316411605952993 ) ) ;
#31235=CYLINDRICAL_SURFACE ( 'NONE', #2637, 4.000000000000000000 ) ;
#31236=CARTESIAN_POINT ( 'NONE',  ( -2.498395430326213790E-14, 17.05624999877096926, 26.00000000000000000 ) ) ;
#31252=CARTESIAN_POINT ( 'NONE',  ( 4.648177544792955741E-15, 14.13124999877096322, 33.99999999999999289 ) ) ;
#31259=CARTESIAN_POINT ( 'NONE',  ( -4.000000000000000888, 14.95624999877096428, 32.30940107675850470 ) ) ;
#31282=LINE ( 'NONE', #7295, #68618 ) ;
#31291=FACE_OUTER_BOUND ( 'NONE', #2659, .T. ) ;
#31319=DIRECTION ( 'NONE',  ( -0.000000000000000000, -1.000000000000000000, -0.000000000000000000 ) ) ;
#31351=CARTESIAN_POINT ( 'NONE',  ( -3.756430356250001434, 13.80312499938548321, 32.16877607737301048 ) ) ;
#31353=CARTESIAN_POINT ( 'NONE',  ( -2.000000000000001776, 15.05000000000000071, 33.46410161513775705 ) ) ;
#31365=DIRECTION ( 'NONE',  ( -0.000000000000000000, -1.000000000000000000, -0.000000000000000000 ) ) ;
#31435=CARTESIAN_POINT ( 'NONE',  ( 2.655984681222220721E-16, 14.21562499938548463, 25.66244784525396483 ) ) ;
#31446=CARTESIAN_POINT ( 'NONE',  ( 1.878215178124997609, 18.86562499938548143, 33.25316411605952993 ) ) ;
#31478=CARTESIAN_POINT ( 'NONE',  ( -1.878215178124999163, 15.60312499938548392, 26.74683588394047007 ) ) ;
#31531=CARTESIAN_POINT ( 'NONE',  ( -4.000000000000000888, 16.75624999877096499, 32.30940107675850470 ) ) ;
#31541=CARTESIAN_POINT ( 'NONE',  ( -3.756430356250001434, 20.10312499938548214, 32.16877607737301048 ) ) ;
#31550=CARTESIAN_POINT ( 'NONE',  ( -1.878215178125001827, 16.99062499938548498, 33.25316411605952283 ) ) ;
#31565=CARTESIAN_POINT ( 'NONE',  ( -3.999999999999999556, 17.13124999877096855, 27.69059892324149175 ) ) ;
#31600=CARTESIAN_POINT ( 'NONE',  ( 3.756430356250000102, 19.95312499938548356, 30.00000000000000000 ) ) ;
#31609=DIRECTION ( 'NONE',  ( -0.000000000000000000, -1.000000000000000000, -0.000000000000000000 ) ) ;
#31639=CARTESIAN_POINT ( 'NONE',  ( -2.000000000000001776, 18.14374999877096428, 33.46410161513775705 ) ) ;
#31691=CARTESIAN_POINT ( 'NONE',  ( -7.967954043666661671E-16, 13.09062499938548285, 34.33755215474603517 ) ) ;
#31718=CARTESIAN_POINT ( 'NONE',  ( 2.655984681222220721E-16, 20.51562499938548356, 25.66244784525396483 ) ) ;
#31720=CARTESIAN_POINT ( 'NONE',  ( -1.999999999999999112, 14.90000000000000036, 26.53589838486224650 ) ) ;
#31732=CARTESIAN_POINT ( 'NONE',  ( 5.000000000000000000, 39.99999999999999289, 30.00000000000000000 ) ) ;
#31757=CARTESIAN_POINT ( 'NONE',  ( -1.071796769724490339, 17.58259618943233349, 26.00000000000000000 ) ) ;
#31759=EDGE_LOOP ( 'NONE', ( #2626, #62075, #48034, #26025 ) ) ;
#31791=LINE ( 'NONE', #60574, #70742 ) ;
#31799=CARTESIAN_POINT ( 'NONE',  ( 1.071796769724491227, 17.93615380933863079, 26.00000000000000000 ) ) ;
#31803=CARTESIAN_POINT ( 'NONE',  ( -1.878215178124999163, 14.70312499938548356, 26.74683588394047007 ) ) ;
#31814=CARTESIAN_POINT ( 'NONE',  ( -1.878215178125001827, 19.24062499938548143, 33.25316411605952283 ) ) ;
#31816=VERTEX_POINT ( 'NONE', #70134 ) ;
#31846=CARTESIAN_POINT ( 'NONE',  ( 1.878215178125000495, 14.62812499938548427, 26.74683588394047007 ) ) ;
#31870=CARTESIAN_POINT ( 'NONE',  ( 1.071796769724485232, 16.13615380933863008, 25.99999999999999645 ) ) ;
#31887=CARTESIAN_POINT ( 'NONE',  ( 0.000000000000000000, 27.50000000000000000, 30.00000000000000000 ) ) ;
#31906=CARTESIAN_POINT ( 'NONE',  ( 2.655984681222220721E-16, 20.40312499938548285, 25.66244784525396483 ) ) ;
#31916=CARTESIAN_POINT ( 'NONE',  ( 3.756430356250000546, 15.82812499938548179, 27.83122392262697886 ) ) ;
#31930=CARTESIAN_POINT ( 'NONE',  ( -8.484601909799255319E-16, 16.38124999877096499, 34.61880215351700940 ) ) ;
#31939=CARTESIAN_POINT ( 'NONE',  ( -4.000000000000000888, 16.30624999877096570, 32.30940107675850470 ) ) ;
#31961=CARTESIAN_POINT ( 'NONE',  ( -3.756430356249999214, 18.79062499938548214, 27.83122392262697176 ) ) ;
#31971=CARTESIAN_POINT ( 'NONE',  ( 2.417052323292336544E-14, 20.48749999999999716, 34.00000000000000000 ) ) ;
#31995=CARTESIAN_POINT ( 'NONE',  ( -3.999999999999999112, 14.88124999877096677, 27.69059892324149530 ) ) ;
#32046=CARTESIAN_POINT ( 'NONE',  ( 3.756430356250000102, 14.44062499938548250, 30.00000000000000000 ) ) ;
#32056=CARTESIAN_POINT ( 'NONE',  ( 2.000000000000000444, 17.07499999999999929, 26.53589838486224650 ) ) ;
#32082=CARTESIAN_POINT ( 'NONE',  ( 3.756430356249998770, 20.36562499938548143, 32.16877607737302469 ) ) ;
#32084=CARTESIAN_POINT ( 'NONE',  ( -2.000000000000001776, 15.50000000000000000, 33.46410161513775705 ) ) ;
#32096=EDGE_LOOP ( 'NONE', ( #72700, #40045, #22628, #24139 ) ) ;
#32108=CARTESIAN_POINT ( 'NONE',  ( 4.000000000000000000, 18.74374999877096570, 30.00000000000000000 ) ) ;
#32146=DIRECTION ( 'NONE',  ( -0.000000000000000000, -1.000000000000000000, -0.000000000000000000 ) ) ;
#32148=ADVANCED_FACE ( 'NONE', ( #34227 ), #22424, .F. ) ;
#32152=DIRECTION ( 'NONE',  ( 1.000000000000000000, 0.000000000000000000, 0.000000000000000000 ) ) ;
#32159=CYLINDRICAL_SURFACE ( 'NONE', #72581, 4.000000000000000000 ) ;
#32163=DIRECTION ( 'NONE',  ( -0.000000000000000000, -1.000000000000000000, -0.000000000000000000 ) ) ;
#32168=CARTESIAN_POINT ( 'NONE',  ( -3.756430356250001434, 14.36562499938548143, 32.16877607737301048 ) ) ;
#32210=CARTESIAN_POINT ( 'NONE',  ( -3.756430356249999214, 15.64062499938548179, 27.83122392262697531 ) ) ;
#32263=CARTESIAN_POINT ( 'NONE',  ( -1.878215178124999163, 13.69062499938548427, 26.74683588394047007 ) ) ;
#32265=CARTESIAN_POINT ( 'NONE',  ( -2.498395430326213790E-14, 18.46250000000000213, 26.00000000000000000 ) ) ;
#32279=CARTESIAN_POINT ( 'NONE',  ( -1.878215178125001827, 19.69062499938548072, 33.25316411605952283 ) ) ;
#32294=CARTESIAN_POINT ( 'NONE',  ( -4.000000000000000000, 15.81874999877096499, 30.00000000000000000 ) ) ;
#32298=EDGE_LOOP ( 'NONE', ( #60979, #45524, #38900, #16708 ) ) ;
#32303=CARTESIAN_POINT ( 'NONE',  ( -3.999999999999999112, 16.23124999877096641, 27.69059892324149530 ) ) ;
#32305=EDGE_CURVE ( 'NONE', #18562, #15973, #62315, .T. ) ;
#32325=CARTESIAN_POINT ( 'NONE',  ( -1.878215178125001827, 20.25312499938548072, 33.25316411605952283 ) ) ;
#32326=CARTESIAN_POINT ( 'NONE',  ( -4.000000000000000888, 14.56250000000000000, 32.30940107675850470 ) ) ;
#32361=CARTESIAN_POINT ( 'NONE',  ( 5.810221930991193690E-16, 14.35624999877096464, 26.00000000000000000 ) ) ;
#32409=CARTESIAN_POINT ( 'NONE',  ( -3.756430356250000102, 13.76562499938548356, 30.00000000000000000 ) ) ;
#32416=CARTESIAN_POINT ( 'NONE',  ( -1.999999999999999112, 18.44374999877096499, 26.53589838486224650 ) ) ;
#32430=ORIENTED_EDGE ( 'NONE', *, *, #4064, .F. ) ;
#32443=ORIENTED_EDGE ( 'NONE', *, *, #19369, .T. ) ;
#32448=CARTESIAN_POINT ( 'NONE',  ( 3.756430356249998770, 15.75312499938548427, 32.16877607737302469 ) ) ;
#32450=CARTESIAN_POINT ( 'NONE',  ( 2.000000000000000444, 14.37500000000000000, 26.53589838486224650 ) ) ;
#32451=CARTESIAN_POINT ( 'NONE',  ( -1.071796769724492115, 17.31740381056766864, 34.00000000000000000 ) ) ;
#32460=VECTOR ( 'NONE', #65613, 1000.000000000000000 ) ;
#32518=DIRECTION ( 'NONE',  ( 0.000000000000000000, 0.000000000000000000, -1.000000000000000000 ) ) ;
#32534=CARTESIAN_POINT ( 'NONE',  ( -3.756430356249999214, 16.09062499938548285, 27.83122392262697531 ) ) ;
#32542=CARTESIAN_POINT ( 'NONE',  ( 1.999999999999997335, 16.41874999877096641, 33.46410161513775705 ) ) ;
#32577=CARTESIAN_POINT ( 'NONE',  ( 1.878215178124997609, 15.82812499938548356, 33.25316411605952993 ) ) ;
#32630=CARTESIAN_POINT ( 'NONE',  ( -3.756430356250000990, 13.80312499938548321, 32.16877607737301048 ) ) ;
#32636=CARTESIAN_POINT ( 'NONE',  ( -3.756430356249999214, 20.02812499938548285, 27.83122392262697531 ) ) ;
#32645=CARTESIAN_POINT ( 'NONE',  ( -7.967954043666661671E-16, 17.47812499938548214, 34.33755215474603517 ) ) ;
#32662=CARTESIAN_POINT ( 'NONE',  ( -1.999999999999999112, 15.74374999877096570, 26.53589838486224650 ) ) ;
#32672=CARTESIAN_POINT ( 'NONE',  ( -1.071796769724486120, 16.36115380933863150, 34.00000000000000000 ) ) ;
#32692=CIRCLE ( 'NONE', #51581, 14.99999999999999822 ) ;
#32707=DIRECTION ( 'NONE',  ( 0.000000000000000000, 0.000000000000000000, -1.000000000000000000 ) ) ;
#32715=VERTEX_POINT ( 'NONE', #31236 ) ;
#32749=CARTESIAN_POINT ( 'NONE',  ( -1.071796769724502107, 18.93259618943233491, 26.00000000000000711 ) ) ;
#32777=CARTESIAN_POINT ( 'NONE',  ( -1.878215178125001827, 12.94062499938548427, 33.25316411605952283 ) ) ;
#32812=CARTESIAN_POINT ( 'NONE',  ( 1.878215178125000495, 15.41562499938548392, 26.74683588394047007 ) ) ;
#32814=CARTESIAN_POINT ( 'NONE',  ( 2.000000000000000444, 17.52499999999999858, 26.53589838486224650 ) ) ;
#32815=CARTESIAN_POINT ( 'NONE',  ( -4.000000000000000888, 17.26249999999999929, 32.30940107675850470 ) ) ;
#32857=( BOUNDED_CURVE ( )  B_SPLINE_CURVE ( 2, ( #14223, #19759, #60377, #31218, #36759, #25684, #54492, #71485, #8686 ),
 .UNSPECIFIED., .F., .F. ) 
 B_SPLINE_CURVE_WITH_KNOTS ( ( 3, 2, 2, 2, 3 ),
 ( 0.7361111111111111605, 0.7407407407407406996, 0.7500000000000000000, 0.7592592592592593004, 0.7638888888888889506 ),
 .UNSPECIFIED. ) 
 CURVE ( )  GEOMETRIC_REPRESENTATION_ITEM ( )  RATIONAL_B_SPLINE_CURVE ( ( 0.9330127018922192983, 0.9330127018922200755, 1.000000000000000000, 0.8660254037844387076, 1.000000000000000000, 0.8660254037844387076, 1.000000000000000000, 0.9330127018922185211, 0.9330127018922192983 ) ) 
 REPRESENTATION_ITEM ( '' )  );
#32895=CARTESIAN_POINT ( 'NONE',  ( -1.878215178125001827, 15.30312499938548321, 33.25316411605952283 ) ) ;
#32902=EDGE_CURVE ( 'NONE', #70914, #68959, #65954, .T. ) ;
#32926=ORIENTED_EDGE ( 'NONE', *, *, #71109, .F. ) ;
#32939=CARTESIAN_POINT ( 'NONE',  ( 1.878215178124997609, 16.72812499938548214, 33.25316411605952993 ) ) ;
#32992=CARTESIAN_POINT ( 'NONE',  ( 1.878215178125000495, 14.51562499938548356, 26.74683588394047007 ) ) ;
#32998=CARTESIAN_POINT ( 'NONE',  ( -1.878215178124999163, 20.44062499938548072, 26.74683588394047007 ) ) ;
#33007=CARTESIAN_POINT ( 'NONE',  ( 3.756430356250000102, 18.04062499938548214, 30.00000000000000000 ) ) ;
#33023=CARTESIAN_POINT ( 'NONE',  ( -3.999999999999999556, 15.78124999877096535, 27.69059892324149175 ) ) ;
#33026=CARTESIAN_POINT ( 'NONE',  ( 0.000000000000000000, 27.50000000000000000, 30.00000000000000000 ) ) ;
#33045=EDGE_CURVE ( 'NONE', #49855, #5101, #4226, .T. ) ;
#33061=ORIENTED_EDGE ( 'NONE', *, *, #15468, .T. ) ;
#33073=EDGE_CURVE ( 'NONE', #44824, #60913, #55245, .T. ) ;
#33089=CARTESIAN_POINT ( 'NONE',  ( 4.000000000000000000, 17.43124999877096570, 27.69059892324149885 ) ) ;
#33136=CARTESIAN_POINT ( 'NONE',  ( 3.756430356250000102, 13.99062499938548498, 30.00000000000000000 ) ) ;
#33145=CARTESIAN_POINT ( 'NONE',  ( 2.655984681222220721E-16, 14.66562499938548214, 25.66244784525396483 ) ) ;
#33173=CARTESIAN_POINT ( 'NONE',  ( -3.756430356250000102, 14.21562499938548285, 30.00000000000000000 ) ) ;
#33175=CARTESIAN_POINT ( 'NONE',  ( -2.000000000000001776, 16.85000000000000142, 33.46410161513775705 ) ) ;
#33219=CARTESIAN_POINT ( 'NONE',  ( -3.999999999999999112, 20.28124999877096712, 27.69059892324149530 ) ) ;
#33232=CARTESIAN_POINT ( 'NONE',  ( 4.000000000000000000, 20.18750000000000000, 27.69059892324149885 ) ) ;
#33250=CARTESIAN_POINT ( 'NONE',  ( -4.000000000000000000, 15.87500000000000000, 30.00000000000000000 ) ) ;
#33259=CARTESIAN_POINT ( 'NONE',  ( -3.756430356250000102, 15.67812499938548143, 30.00000000000000000 ) ) ;
#33266=DIRECTION ( 'NONE',  ( -0.000000000000000000, -1.000000000000000000, -0.000000000000000000 ) ) ;
#33287=( BOUNDED_CURVE ( )  B_SPLINE_CURVE ( 2, ( #48963, #20870, #4271, #64474, #65945, #32326, #27890, #183, #4631 ),
 .UNSPECIFIED., .F., .F. ) 
 B_SPLINE_CURVE_WITH_KNOTS ( ( 3, 2, 2, 2, 3 ),
 ( 0.2361111111111111049, 0.2407407407407407274, 0.2500000000000000000, 0.2592592592592592449, 0.2638888888888888951 ),
 .UNSPECIFIED. ) 
 CURVE ( )  GEOMETRIC_REPRESENTATION_ITEM ( )  RATIONAL_B_SPLINE_CURVE ( ( 0.9330127018922194093, 0.9330127018922194093, 1.000000000000000000, 0.8660254037844387076, 1.000000000000000000, 0.8660254037844387076, 1.000000000000000000, 0.9330127018922194093, 0.9330127018922194093 ) ) 
 REPRESENTATION_ITEM ( '' )  );
#33302=CARTESIAN_POINT ( 'NONE',  ( -3.756430356250001434, 16.61562499938548143, 32.16877607737301048 ) ) ;
#33356=CARTESIAN_POINT ( 'NONE',  ( -3.756430356250000990, 14.70312499938548179, 32.16877607737301048 ) ) ;
#33372=CARTESIAN_POINT ( 'NONE',  ( 3.756430356249998770, 19.35312499938548214, 32.16877607737302469 ) ) ;
#33386=CARTESIAN_POINT ( 'NONE',  ( -8.484601909799255319E-16, 19.53124999877096712, 34.61880215351700940 ) ) ;
#33389=CARTESIAN_POINT ( 'NONE',  ( 1.071796769724489673, 13.04240381056766829, 26.00000000000000000 ) ) ;
#33445=CARTESIAN_POINT ( 'NONE',  ( 3.756430356250000102, 12.75312499938548427, 30.00000000000000000 ) ) ;
#33498=CARTESIAN_POINT ( 'NONE',  ( -3.756430356250000990, 14.81562499938548427, 32.16877607737301048 ) ) ;
#33527=CARTESIAN_POINT ( 'NONE',  ( -1.878215178125001827, 14.29062499938548392, 33.25316411605952283 ) ) ;
#33530=CARTESIAN_POINT ( 'NONE',  ( 4.000000000000000000, 17.89999999999999858, 30.00000000000000000 ) ) ;
#33550=CARTESIAN_POINT ( 'NONE',  ( 4.000000000000000000, 20.13124999877096499, 27.69059892324149885 ) ) ;
#33577=CARTESIAN_POINT ( 'NONE',  ( -1.626862140677534273E-15, 20.43124999877096570, 34.00000000000000000 ) ) ;
#33615=CARTESIAN_POINT ( 'NONE',  ( -3.756430356250000102, 16.12812499938548427, 30.00000000000000000 ) ) ;
#33659=CARTESIAN_POINT ( 'NONE',  ( -3.756430356250000102, 16.57812499938548356, 30.00000000000000000 ) ) ;
#33717=CARTESIAN_POINT ( 'NONE',  ( 1.878215178124997609, 14.81562499938548427, 33.25316411605952993 ) ) ;
#33733=CARTESIAN_POINT ( 'NONE',  ( 1.878215178125000495, 18.11562499938548498, 26.74683588394047007 ) ) ;
#33747=CARTESIAN_POINT ( 'NONE',  ( -4.000000000000000888, 18.55624999877096570, 32.30940107675850470 ) ) ;
#33757=CARTESIAN_POINT ( 'NONE',  ( 1.138803498474273873E-14, 15.98750000000000249, 34.00000000000000000 ) ) ;
#33769=( BOUNDED_CURVE ( )  B_SPLINE_CURVE ( 2, ( #66403, #37956, #8787, #70847, #60476, #54956, #32056, #20220, #42775 ),
 .UNSPECIFIED., .F., .F. ) 
 B_SPLINE_CURVE_WITH_KNOTS ( ( 3, 2, 2, 2, 3 ),
 ( 0.5416666666666667407, 0.5462962962962962798, 0.5555555555555555802, 0.5648148148148147696, 0.5694444444444444198 ),
 .UNSPECIFIED. ) 
 CURVE ( )  GEOMETRIC_REPRESENTATION_ITEM ( )  RATIONAL_B_SPLINE_CURVE ( ( 0.9330127018922192983, 0.9330127018922200755, 1.000000000000000000, 0.8660254037844387076, 1.000000000000000000, 0.8660254037844387076, 1.000000000000000000, 0.9330127018922194093, 0.9330127018922194093 ) ) 
 REPRESENTATION_ITEM ( '' )  );
#33775=FACE_OUTER_BOUND ( 'NONE', #37795, .T. ) ;
#33829=DIRECTION ( 'NONE',  ( -0.000000000000000000, -1.000000000000000000, -0.000000000000000000 ) ) ;
#33859=EDGE_CURVE ( 'NONE', #55447, #16877, #52580, .T. ) ;
#33864=CARTESIAN_POINT ( 'NONE',  ( -3.756430356249999214, 15.64062499938548356, 27.83122392262697176 ) ) ;
#33865=CARTESIAN_POINT ( 'NONE',  ( -1.243387493232115393E-14, 15.25624999877096677, 26.00000000000000000 ) ) ;
#33877=EDGE_LOOP ( 'NONE', ( #50649, #17523, #33061, #197 ) ) ;
#33894=CARTESIAN_POINT ( 'NONE',  ( -1.999999999999999112, 18.50000000000000000, 26.53589838486224650 ) ) ;
#33938=CARTESIAN_POINT ( 'NONE',  ( -4.000000000000000888, 13.15624999877096535, 32.30940107675850470 ) ) ;
#33976=CARTESIAN_POINT ( 'NONE',  ( 1.878215178124997609, 17.17812499938548498, 33.25316411605952993 ) ) ;
#33989=CARTESIAN_POINT ( 'NONE',  ( 3.756430356250000102, 12.75312499938548427, 30.00000000000000000 ) ) ;
#34019=CARTESIAN_POINT ( 'NONE',  ( -3.756430356249999214, 17.44062499938548427, 27.83122392262697531 ) ) ;
#34071=CARTESIAN_POINT ( 'NONE',  ( 3.756430356250000546, 18.07812499938548711, 27.83122392262697886 ) ) ;
#34073=DIRECTION ( 'NONE',  ( 0.000000000000000000, 0.000000000000000000, -1.000000000000000000 ) ) ;
#34104=CARTESIAN_POINT ( 'NONE',  ( -1.999999999999999112, 17.54374999877096641, 26.53589838486224650 ) ) ;
#34178=EDGE_CURVE ( 'NONE', #54204, #38333, #53686, .T. ) ;
#34221=CARTESIAN_POINT ( 'NONE',  ( 3.756430356250000102, 13.65312499938548285, 30.00000000000000000 ) ) ;
#34227=FACE_OUTER_BOUND ( 'NONE', #274, .T. ) ;
#34231=ORIENTED_EDGE ( 'NONE', *, *, #51961, .T. ) ;
#34252=CARTESIAN_POINT ( 'NONE',  ( -2.000000000000001776, 16.40000000000000213, 33.46410161513775705 ) ) ;
#34265=ORIENTED_EDGE ( 'NONE', *, *, #61021, .F. ) ;
#34272=ADVANCED_FACE ( 'NONE', ( #21153 ), #20418, .T. ) ;
#34334=CARTESIAN_POINT ( 'NONE',  ( 3.756430356250000546, 18.64062499938548001, 27.83122392262697886 ) ) ;
#34344=CARTESIAN_POINT ( 'NONE',  ( -1.243387493232115393E-14, 16.21250000000000213, 26.00000000000000000 ) ) ;
#34375=CARTESIAN_POINT ( 'NONE',  ( 2.655984681222220721E-16, 18.26562499938548356, 25.66244784525396483 ) ) ;
#34382=COLOUR_RGB ( '',0.8941176470588234615, 0.8941176470588234615, 0.8941176470588234615 ) ;
#34391=DIRECTION ( 'NONE',  ( 0.000000000000000000, 0.000000000000000000, -1.000000000000000000 ) ) ;
#34405=CARTESIAN_POINT ( 'NONE',  ( 4.000000000000000000, 13.34374999877096712, 30.00000000000000000 ) ) ;
#34435=CARTESIAN_POINT ( 'NONE',  ( -7.967954043666661671E-16, 16.12812499938548427, 34.33755215474603517 ) ) ;
#34466=CARTESIAN_POINT ( 'NONE',  ( -2.000000000000001776, 19.04374999877096641, 33.46410161513775705 ) ) ;
#34476=CARTESIAN_POINT ( 'NONE',  ( 4.000000000000000000, 16.13749999999999929, 27.69059892324149885 ) ) ;
#34493=CARTESIAN_POINT ( 'NONE',  ( 4.000000000000000000, 14.78749999999999964, 27.69059892324149885 ) ) ;
#34513=ORIENTED_EDGE ( 'NONE', *, *, #72602, .T. ) ;
#34586=CARTESIAN_POINT ( 'NONE',  ( -1.878215178124999163, 16.05312499938548143, 26.74683588394047007 ) ) ;
#34599=ORIENTED_EDGE ( 'NONE', *, *, #49494, .T. ) ;
#34616=CARTESIAN_POINT ( 'NONE',  ( 3.999999999999998668, 19.66249999999999787, 32.30940107675850470 ) ) ;
#34630=CARTESIAN_POINT ( 'NONE',  ( -2.672702088255949472E-15, 13.90624999877096890, 26.00000000000000000 ) ) ;
#34654=EDGE_LOOP ( 'NONE', ( #44898, #210, #1919, #8018 ) ) ;
#34656=FACE_OUTER_BOUND ( 'NONE', #54791, .T. ) ;
#34692=AXIS2_PLACEMENT_3D ( 'NONE', #41315, #6238, #63825 ) ;
#34700=CARTESIAN_POINT ( 'NONE',  ( -3.756430356249999214, 18.34062499938548640, 27.83122392262697531 ) ) ;
#34702=CARTESIAN_POINT ( 'NONE',  ( 1.999999999999997335, 13.32499999999999929, 33.46410161513775705 ) ) ;
#34749=ORIENTED_EDGE ( 'NONE', *, *, #40081, .F. ) ;
#34795=CARTESIAN_POINT ( 'NONE',  ( 4.898587196589412829E-16, 27.50000000000000000, 34.00000000000000000 ) ) ;
#34797=CARTESIAN_POINT ( 'NONE',  ( 2.655984681222220721E-16, 17.25312499938548072, 25.66244784525396483 ) ) ;
#34799=AXIS2_PLACEMENT_3D ( 'NONE', #43470, #54913, #9845 ) ;
#34831=CARTESIAN_POINT ( 'NONE',  ( -4.000000000000000888, 19.45624999877097139, 32.30940107675850470 ) ) ;
#34891=CARTESIAN_POINT ( 'NONE',  ( -1.878215178124999163, 14.14062499938548356, 26.74683588394047007 ) ) ;
#34930=EDGE_CURVE ( 'NONE', #23775, #45011, #51872, .T. ) ;
#34954=CARTESIAN_POINT ( 'NONE',  ( 1.878215178124997609, 16.27812499938548285, 33.25316411605952993 ) ) ;
#34966=ORIENTED_EDGE ( 'NONE', *, *, #41247, .F. ) ;
#34988=CARTESIAN_POINT ( 'NONE',  ( -4.000000000000000000, 19.92499999999999716, 30.00000000000000000 ) ) ;
#35012=CARTESIAN_POINT ( 'NONE',  ( 1.138803498474273873E-14, 15.48124999877096641, 34.00000000000000000 ) ) ;
#35022=ORIENTED_EDGE ( 'NONE', *, *, #5433, .T. ) ;
#35024=CARTESIAN_POINT ( 'NONE',  ( 1.071796769724491893, 14.20759618943233527, 34.00000000000000000 ) ) ;
#35034=CARTESIAN_POINT ( 'NONE',  ( 1.071796769724488785, 17.80759618943233491, 34.00000000000000000 ) ) ;
#35062=DIRECTION ( 'NONE',  ( 0.000000000000000000, 0.000000000000000000, -1.000000000000000000 ) ) ;
#35065=EDGE_CURVE ( 'NONE', #9585, #47310, #58983, .T. ) ;
#35070=CARTESIAN_POINT ( 'NONE',  ( -1.878215178125001827, 17.55312499938548498, 33.25316411605952283 ) ) ;
#35072=CARTESIAN_POINT ( 'NONE',  ( -3.756430356250000102, 20.51562499938548356, 30.00000000000000000 ) ) ;
#35090=EDGE_CURVE ( 'NONE', #41056, #54204, #1830, .T. ) ;
#35108=CARTESIAN_POINT ( 'NONE',  ( 1.878215178124997609, 19.87812499938548072, 33.25316411605952993 ) ) ;
#35134=CARTESIAN_POINT ( 'NONE',  ( 1.071796769724489673, 13.43615380933863435, 26.00000000000000000 ) ) ;
#35147=ORIENTED_EDGE ( 'NONE', *, *, #65184, .F. ) ;
#35165=CARTESIAN_POINT ( 'NONE',  ( 2.655984681222220721E-16, 17.70312499938548356, 25.66244784525396483 ) ) ;
#35193=CARTESIAN_POINT ( 'NONE',  ( 3.756430356250000546, 13.69062499938548250, 27.83122392262697886 ) ) ;
#35220=CARTESIAN_POINT ( 'NONE',  ( 0.000000000000000000, 27.50000000000000000, 26.00000000000000000 ) ) ;
#35254=CARTESIAN_POINT ( 'NONE',  ( -3.756430356250001434, 17.85312499938548214, 32.16877607737301048 ) ) ;
#35271=( BOUNDED_CURVE ( )  B_SPLINE_CURVE ( 2, ( #66137, #26624, #26993, #49161, #33250, #65771, #43615, #71692, #55426 ),
 .UNSPECIFIED., .F., .F. ) 
 B_SPLINE_CURVE_WITH_KNOTS ( ( 3, 2, 2, 2, 3 ),
 ( 0.4027777777777777901, 0.4074074074074073848, 0.4166666666666666852, 0.4259259259259259300, 0.4305555555555555802 ),
 .UNSPECIFIED. ) 
 CURVE ( )  GEOMETRIC_REPRESENTATION_ITEM ( )  RATIONAL_B_SPLINE_CURVE ( ( 0.9330127018922194093, 0.9330127018922197424, 1.000000000000000000, 0.8660254037844387076, 1.000000000000000000, 0.8660254037844387076, 1.000000000000000000, 0.9330127018922189652, 0.9330127018922194093 ) ) 
 REPRESENTATION_ITEM ( '' )  );
#35279=CARTESIAN_POINT ( 'NONE',  ( -8.484601909799255319E-16, 13.68124999877096748, 34.61880215351700940 ) ) ;
#35282=CARTESIAN_POINT ( 'NONE',  ( -2.498395430326213790E-14, 19.30624999877096926, 26.00000000000000000 ) ) ;
#35283=ORIENTED_EDGE ( 'NONE', *, *, #72649, .T. ) ;
#35313=CARTESIAN_POINT ( 'NONE',  ( -3.756430356250000990, 17.06562499938548072, 32.16877607737301048 ) ) ;
#35360=VERTEX_POINT ( 'NONE', #4893 ) ;
#35383=CARTESIAN_POINT ( 'NONE',  ( 2.000000000000000444, 14.37500000000000000, 26.53589838486224650 ) ) ;
#35409=CARTESIAN_POINT ( 'NONE',  ( 3.871028493210608712, 25.03395833444976404, 31.04107391399921312 ) ) ;
#35426=CARTESIAN_POINT ( 'NONE',  ( -1.878215178125001827, 19.35312499938548214, 33.25316411605952283 ) ) ;
#35428=CARTESIAN_POINT ( 'NONE',  ( -1.878215178125001827, 20.14062499938548356, 33.25316411605952283 ) ) ;
#35466=CARTESIAN_POINT ( 'NONE',  ( 3.756430356249998770, 19.46562499938548285, 32.16877607737302469 ) ) ;
#35492=DIRECTION ( 'NONE',  ( -0.000000000000000000, -1.000000000000000000, -0.000000000000000000 ) ) ;
#35524=CARTESIAN_POINT ( 'NONE',  ( -1.878215178125001827, 17.44062499938548072, 33.25316411605952283 ) ) ;
#35553=CARTESIAN_POINT ( 'NONE',  ( -3.756430356250000102, 13.42812499938548321, 30.00000000000000000 ) ) ;
#35563=ADVANCED_FACE ( 'NONE', ( #12600 ), #57657, .T. ) ;
#35592=EDGE_LOOP ( 'NONE', ( #68093, #64811, #46064, #52243 ) ) ;
#35606=ORIENTED_EDGE ( 'NONE', *, *, #20857, .F. ) ;
#35615=CARTESIAN_POINT ( 'NONE',  ( -7.967954043666661671E-16, 16.57812499938548356, 34.33755215474603517 ) ) ;
#35633=CARTESIAN_POINT ( 'NONE',  ( 1.999999999999997335, 17.37500000000000000, 33.46410161513775705 ) ) ;
#35639=CARTESIAN_POINT ( 'NONE',  ( 4.000000000000000000, 13.38124999877096677, 27.69059892324149530 ) ) ;
#35672=CARTESIAN_POINT ( 'NONE',  ( 3.756430356249998770, 17.66562499938548214, 32.16877607737301759 ) ) ;
#35676=ORIENTED_EDGE ( 'NONE', *, *, #49591, .F. ) ;
#35707=CARTESIAN_POINT ( 'NONE',  ( -4.000000000000000000, 19.02499999999999858, 30.00000000000000000 ) ) ;
#35710=CARTESIAN_POINT ( 'NONE',  ( -3.999999999999999112, 19.38124999877096144, 27.69059892324149530 ) ) ;
#35771=CARTESIAN_POINT ( 'NONE',  ( 1.292354794015584840, 25.48750161887817711, 33.79447915781519640 ) ) ;
#35786=CARTESIAN_POINT ( 'NONE',  ( 1.878215178124997609, 18.52812499938548285, 33.25316411605952993 ) ) ;
#35788=CARTESIAN_POINT ( 'NONE',  ( 3.756430356250000546, 19.87812499938548427, 27.83122392262697886 ) ) ;
#35800=ORIENTED_EDGE ( 'NONE', *, *, #4284, .F. ) ;
#35825=CARTESIAN_POINT ( 'NONE',  ( 3.756430356250000102, 19.95312499938548356, 30.00000000000000000 ) ) ;
#35841=( BOUNDED_CURVE ( )  B_SPLINE_CURVE ( 2, ( #21629, #48261, #26827, #31995, #65607, #31259, #44187, #37532, #49361 ),
 .UNSPECIFIED., .F., .F. ) 
 B_SPLINE_CURVE_WITH_KNOTS ( ( 3, 2, 2, 2, 3 ),
 ( 0.2361111111111111049, 0.2407407407407407274, 0.2500000000000000000, 0.2592592592592592449, 0.2638888888888888951 ),
 .UNSPECIFIED. ) 
 CURVE ( )  GEOMETRIC_REPRESENTATION_ITEM ( )  RATIONAL_B_SPLINE_CURVE ( ( 0.9330127018922194093, 0.9330127018922194093, 1.000000000000000000, 0.8660254037844387076, 1.000000000000000000, 0.8660254037844387076, 1.000000000000000000, 0.9330127018922194093, 0.9330127018922194093 ) ) 
 REPRESENTATION_ITEM ( '' )  );
#35865=CARTESIAN_POINT ( 'NONE',  ( -3.974286678381309112, 25.00691767267703725, 29.47675606540910209 ) ) ;
#35880=CARTESIAN_POINT ( 'NONE',  ( 2.655984681222220721E-16, 19.95312499938548356, 25.66244784525396483 ) ) ;
#35912=CARTESIAN_POINT ( 'NONE',  ( 4.000000000000000000, 20.09374999877096712, 30.00000000000000000 ) ) ;
#35958=VECTOR ( 'NONE', #17439, 1000.000000000000000 ) ;
#35979=CARTESIAN_POINT ( 'NONE',  ( -1.878215178125001827, 16.99062499938548498, 33.25316411605952283 ) ) ;
#36002=CARTESIAN_POINT ( 'NONE',  ( 2.828200636599751609E-16, 13.90624999877096535, 25.38119784648299415 ) ) ;
#36023=VECTOR ( 'NONE', #57605, 1000.000000000000000 ) ;
#36038=CARTESIAN_POINT ( 'NONE',  ( 3.756430356249998770, 16.31562499938548427, 32.16877607737301759 ) ) ;
#36078=CARTESIAN_POINT ( 'NONE',  ( -4.000000000000000000, 19.41874999877096641, 30.00000000000000000 ) ) ;
#36082=( BOUNDED_CURVE ( )  B_SPLINE_CURVE ( 2, ( #53183, #31757, #48385, #60175, #42838, #31016, #2580, #71648, #54294 ),
 .UNSPECIFIED., .F., .F. ) 
 B_SPLINE_CURVE_WITH_KNOTS ( ( 3, 2, 2, 2, 3 ),
 ( 0.6250000000000000000, 0.6296296296296296502, 0.6388888888888888395, 0.6481481481481481399, 0.6527777777777777901 ),
 .UNSPECIFIED. ) 
 CURVE ( )  GEOMETRIC_REPRESENTATION_ITEM ( )  RATIONAL_B_SPLINE_CURVE ( ( 0.9330127018922194093, 0.9330127018922194093, 1.000000000000000000, 0.8660254037844387076, 1.000000000000000000, 0.8660254037844387076, 1.000000000000000000, 0.9330127018922194093, 0.9330127018922194093 ) ) 
 REPRESENTATION_ITEM ( '' )  );
#36093=CARTESIAN_POINT ( 'NONE',  ( 5.810221930991193690E-16, 19.75624999877096499, 26.00000000000000000 ) ) ;
#36112=CARTESIAN_POINT ( 'NONE',  ( 4.000000000000000000, 18.29374999877096641, 30.00000000000000000 ) ) ;
#36142=CARTESIAN_POINT ( 'NONE',  ( 3.470266163325922193, 25.13317678729335114, 27.99341696106071353 ) ) ;
#36158=CARTESIAN_POINT ( 'NONE',  ( 1.878215178124997609, 13.01562499938548356, 33.25316411605952993 ) ) ;
#36160=CARTESIAN_POINT ( 'NONE',  ( -4.000000000000000000, 12.72499999999999964, 30.00000000000000000 ) ) ;
#36172=VECTOR ( 'NONE', #25494, 1000.000000000000000 ) ;
#36240=CARTESIAN_POINT ( 'NONE',  ( -1.774630419999661868, 25.43662396648353408, 33.59426316867342166 ) ) ;
#36256=CARTESIAN_POINT ( 'NONE',  ( 0.6522972858965978560, 20.64114861271052348, 33.69936173848522998 ) ) ;
#36288=CARTESIAN_POINT ( 'NONE',  ( 1.999999999999997335, 20.01874999877096428, 33.46410161513775705 ) ) ;
#36300=VERTEX_POINT ( 'NONE', #37320 ) ;
#36311=CARTESIAN_POINT ( 'NONE',  ( -2.498395430326213790E-14, 20.26249999999999929, 26.00000000000000000 ) ) ;
#36312=CARTESIAN_POINT ( 'NONE',  ( 4.000000000000000000, 16.04374999877096641, 30.00000000000000000 ) ) ;
#36350=CARTESIAN_POINT ( 'NONE',  ( 1.878215178124997609, 17.06562499938548072, 33.25316411605952993 ) ) ;
#36359=CARTESIAN_POINT ( 'NONE',  ( 2.655984681222220721E-16, 15.90312499938548108, 25.66244784525396483 ) ) ;
#36372=FACE_OUTER_BOUND ( 'NONE', #70627, .T. ) ;
#36375=CARTESIAN_POINT ( 'NONE',  ( 3.999999999999998668, 19.15624999877096712, 32.30940107675850470 ) ) ;
#36408=CARTESIAN_POINT ( 'NONE',  ( 3.756430356250000102, 19.05312499938548143, 30.00000000000000000 ) ) ;
#36446=CARTESIAN_POINT ( 'NONE',  ( -1.626862140677534273E-15, 19.53124999877096357, 34.00000000000000000 ) ) ;
#36466=CARTESIAN_POINT ( 'NONE',  ( 5.000000000000000000, 39.99999999999999289, 45.00000000000000000 ) ) ;
#36498=CYLINDRICAL_SURFACE ( 'NONE', #27718, 4.000000000000000000 ) ;
#36504=CARTESIAN_POINT ( 'NONE',  ( 3.492397243767003889, 25.12859708874951892, 32.01989049841399293 ) ) ;
#36521=CARTESIAN_POINT ( 'NONE',  ( -1.878215178125001827, 12.94062499938548427, 33.25316411605952283 ) ) ;
#36523=CARTESIAN_POINT ( 'NONE',  ( 2.000000000000000444, 15.72499999999999964, 26.53589838486224650 ) ) ;
#36590=CARTESIAN_POINT ( 'NONE',  ( 4.000000000000000000, 20.54374999877096641, 30.00000000000000000 ) ) ;
#36600=CARTESIAN_POINT ( 'NONE',  ( -4.000059620491343892, 24.99998410120267778, 29.73716349952571392 ) ) ;
#36603=CARTESIAN_POINT ( 'NONE',  ( -1.878215178125001827, 13.05312499938548321, 33.25316411605952283 ) ) ;
#36646=CARTESIAN_POINT ( 'NONE',  ( -3.999999999999999556, 20.28124999877096712, 27.69059892324149175 ) ) ;
#36700=CARTESIAN_POINT ( 'NONE',  ( 3.756430356250000102, 12.64062499938548356, 30.00000000000000000 ) ) ;
#36707=CARTESIAN_POINT ( 'NONE',  ( -3.756430356249999214, 18.22812499938548214, 27.83122392262697531 ) ) ;
#36716=CARTESIAN_POINT ( 'NONE',  ( -3.756430356250000102, 16.01562499938548356, 30.00000000000000000 ) ) ;
#36732=CARTESIAN_POINT ( 'NONE',  ( 1.999999999999997335, 13.71874999877096535, 33.46410161513775705 ) ) ;
#36759=CARTESIAN_POINT ( 'NONE',  ( -4.000000000000000000, 18.57500000000000284, 30.00000000000000000 ) ) ;
#36765=CARTESIAN_POINT ( 'NONE',  ( -4.000000000000000888, 12.76250000000000107, 32.30940107675850470 ) ) ;
#36768=CARTESIAN_POINT ( 'NONE',  ( 2.655984681222220721E-16, 19.16562499938548214, 25.66244784525396483 ) ) ;
#36831=CARTESIAN_POINT ( 'NONE',  ( 2.411242101361345515E-14, 20.88124999877096499, 34.00000000000000000 ) ) ;
#36887=CARTESIAN_POINT ( 'NONE',  ( -1.878215178125001827, 20.25312499938548072, 33.25316411605952283 ) ) ;
#36889=CARTESIAN_POINT ( 'NONE',  ( 1.999999999999997335, 15.12500000000000000, 33.46410161513775705 ) ) ;
#36924=EDGE_LOOP ( 'NONE', ( #59760, #32430, #47460, #65732 ) ) ;
#36957=CARTESIAN_POINT ( 'NONE',  ( -1.626862140677534273E-15, 16.43750000000000000, 34.00000000000000000 ) ) ;
#36969=CARTESIAN_POINT ( 'NONE',  ( 1.878215178124997609, 14.47812499938548214, 33.25316411605952993 ) ) ;
#36980=CARTESIAN_POINT ( 'NONE',  ( 2.655984681222220721E-16, 18.60312499938548925, 25.66244784525396483 ) ) ;
#37011=CARTESIAN_POINT ( 'NONE',  ( 3.756430356249998770, 14.06562499938548250, 32.16877607737302469 ) ) ;
#37062=CARTESIAN_POINT ( 'NONE',  ( -1.071796769724496334, 16.62634618820329990, 26.00000000000000355 ) ) ;
#37065=CARTESIAN_POINT ( 'NONE',  ( -1.878215178125001827, 13.39062499938548356, 33.25316411605952283 ) ) ;
#37073=CARTESIAN_POINT ( 'NONE',  ( -3.756430356249999214, 19.57812499938548001, 27.83122392262697531 ) ) ;
#37082=CARTESIAN_POINT ( 'NONE',  ( -1.878215178124999163, 16.39062499938548356, 26.74683588394047007 ) ) ;
#37090=CARTESIAN_POINT ( 'NONE',  ( 1.071796769724488785, 17.35759618943233562, 34.00000000000000000 ) ) ;
#37096=CARTESIAN_POINT ( 'NONE',  ( 4.000000000000000000, 15.18124999877096570, 27.69059892324149530 ) ) ;
#37100=ORIENTED_EDGE ( 'NONE', *, *, #33859, .F. ) ;
#37118=AXIS2_PLACEMENT_3D ( 'NONE', #24492, #69571, #11966 ) ;
#37128=CARTESIAN_POINT ( 'NONE',  ( 2.655984681222220721E-16, 18.71562499938548285, 25.66244784525396483 ) ) ;
#37136=LINE ( 'NONE', #20498, #40747 ) ;
#37138=CARTESIAN_POINT ( 'NONE',  ( 5.810221930991193690E-16, 17.11249999999999716, 26.00000000000000000 ) ) ;
#37175=ADVANCED_FACE ( 'NONE', ( #19863 ), #36498, .T. ) ;
#37204=VECTOR ( 'NONE', #21763, 1000.000000000000000 ) ;
#37225=CARTESIAN_POINT ( 'NONE',  ( 3.756430356249998770, 13.16562499938548392, 32.16877607737301759 ) ) ;
#37239=ORIENTED_EDGE ( 'NONE', *, *, #42756, .T. ) ;
#37255=CARTESIAN_POINT ( 'NONE',  ( 3.756430356250000546, 20.44062499938547717, 27.83122392262697886 ) ) ;
#37257=CARTESIAN_POINT ( 'NONE',  ( 4.000000000000000000, 13.85000000000000142, 30.00000000000000000 ) ) ;
#37293=ORIENTED_EDGE ( 'NONE', *, *, #70290, .F. ) ;
#37320=CARTESIAN_POINT ( 'NONE',  ( -1.243387493232115393E-14, 15.25624999877096499, 26.00000000000000000 ) ) ;
#37341=CARTESIAN_POINT ( 'NONE',  ( 1.878215178124997609, 14.02812499938548285, 33.25316411605952993 ) ) ;
#37347=ADVANCED_FACE ( 'NONE', ( #14686 ), #42049, .T. ) ;
#37353=CARTESIAN_POINT ( 'NONE',  ( -7.967954043666661671E-16, 19.27812499938548640, 34.33755215474603517 ) ) ;
#37364=CARTESIAN_POINT ( 'NONE',  ( 5.810221930991193690E-16, 14.80624999877096570, 26.00000000000000000 ) ) ;
#37371=ORIENTED_EDGE ( 'NONE', *, *, #64830, .F. ) ;
#37384=CARTESIAN_POINT ( 'NONE',  ( 1.878215178124997609, 16.27812499938548285, 33.25316411605952993 ) ) ;
#37424=DIRECTION ( 'NONE',  ( -0.000000000000000000, -1.000000000000000000, -0.000000000000000000 ) ) ;
#37439=CARTESIAN_POINT ( 'NONE',  ( 3.756430356250000102, 13.54062499938548392, 30.00000000000000000 ) ) ;
#37446=CARTESIAN_POINT ( 'NONE',  ( -1.878215178125001827, 18.79062499938548214, 33.25316411605952283 ) ) ;
#37456=CARTESIAN_POINT ( 'NONE',  ( 3.756430356250000102, 17.14062499938548356, 30.00000000000000000 ) ) ;
#37470=CARTESIAN_POINT ( 'NONE',  ( -8.484601909799255319E-16, 15.03124999877096535, 34.61880215351700940 ) ) ;
#37501=CARTESIAN_POINT ( 'NONE',  ( 2.655984681222220721E-16, 20.06562499938548427, 25.66244784525396483 ) ) ;
#37526=CARTESIAN_POINT ( 'NONE',  ( 1.999999999999997335, 14.16874999877096641, 33.46410161513775705 ) ) ;
#37532=CARTESIAN_POINT ( 'NONE',  ( -1.071796769724492115, 15.01115380933863186, 34.00000000000000000 ) ) ;
#37582=CARTESIAN_POINT ( 'NONE',  ( -7.967954043666661671E-16, 14.77812499938548463, 34.33755215474603517 ) ) ;
#37592=CARTESIAN_POINT ( 'NONE',  ( 1.878215178125000495, 13.27812499938548285, 26.74683588394047007 ) ) ;
#37617=CARTESIAN_POINT ( 'NONE',  ( -0.6941602726958887581, 20.72676555956768851, 33.93677853444431491 ) ) ;
#37619=CARTESIAN_POINT ( 'NONE',  ( -4.000000000000000888, 15.91249999999999964, 32.30940107675850470 ) ) ;
#37620=CARTESIAN_POINT ( 'NONE',  ( 5.810221930991193690E-16, 17.11249999999999716, 26.00000000000000000 ) ) ;
#37624=LINE ( 'NONE', #60147, #55046 ) ;
#37699=CARTESIAN_POINT ( 'NONE',  ( 3.756430356249998770, 13.61562499938548498, 32.16877607737302469 ) ) ;
#37739=ORIENTED_EDGE ( 'NONE', *, *, #67048, .F. ) ;
#37743=CARTESIAN_POINT ( 'NONE',  ( -1.878215178124999163, 14.25312499938548250, 26.74683588394047007 ) ) ;
#37745=EDGE_CURVE ( 'NONE', #68118, #29564, #67429, .T. ) ;
#37795=EDGE_LOOP ( 'NONE', ( #67986, #50223, #10482, #25626 ) ) ;
#37799=CARTESIAN_POINT ( 'NONE',  ( -1.071796769724489229, 14.16740381056766473, 34.00000000000000000 ) ) ;
#37806=CARTESIAN_POINT ( 'NONE',  ( 3.756430356250000546, 19.87812499938548427, 27.83122392262697886 ) ) ;
#37816=CARTESIAN_POINT ( 'NONE',  ( 1.878215178124997609, 15.26562499938548179, 33.25316411605952993 ) ) ;
#37831=CARTESIAN_POINT ( 'NONE',  ( 3.999999999999998668, 15.55624999877096748, 32.30940107675850470 ) ) ;
#37860=VECTOR ( 'NONE', #71968, 1000.000000000000000 ) ;
#37861=( BOUNDED_CURVE ( )  B_SPLINE_CURVE ( 2, ( #13206, #40575, #69018, #47203, #6954, #63463, #41304, #46118, #58266 ),
 .UNSPECIFIED., .F., .F. ) 
 B_SPLINE_CURVE_WITH_KNOTS ( ( 3, 2, 2, 2, 3 ),
 ( 0.3194444444444444753, 0.3240740740740740700, 0.3333333333333333148, 0.3425925925925926152, 0.3472222222222222654 ),
 .UNSPECIFIED. ) 
 CURVE ( )  GEOMETRIC_REPRESENTATION_ITEM ( )  RATIONAL_B_SPLINE_CURVE ( ( 0.9330127018922194093, 0.9330127018922197424, 1.000000000000000000, 0.8660254037844387076, 1.000000000000000000, 0.8660254037844387076, 1.000000000000000000, 0.9330127018922189652, 0.9330127018922194093 ) ) 
 REPRESENTATION_ITEM ( '' )  );
#37865=CARTESIAN_POINT ( 'NONE',  ( -7.967954043666661671E-16, 18.49062499938548143, 34.33755215474603517 ) ) ;
#37887=( BOUNDED_CURVE ( )  B_SPLINE_CURVE ( 2, ( #51305, #35034, #18030, #1435, #40586, #63106, #52032, #58277, #69397 ),
 .UNSPECIFIED., .F., .F. ) 
 B_SPLINE_CURVE_WITH_KNOTS ( ( 3, 2, 2, 2, 3 ),
 ( 0.6527777777777777901, 0.6574074074074074403, 0.6666666666666666297, 0.6759259259259259300, 0.6805555555555555802 ),
 .UNSPECIFIED. ) 
 CURVE ( )  GEOMETRIC_REPRESENTATION_ITEM ( )  RATIONAL_B_SPLINE_CURVE ( ( 0.9330127018922194093, 0.9330127018922194093, 1.000000000000000000, 0.8660254037844387076, 1.000000000000000000, 0.8660254037844387076, 1.000000000000000000, 0.9330127018922194093, 0.9330127018922194093 ) ) 
 REPRESENTATION_ITEM ( '' )  );
#37895=STYLED_ITEM('',(#73144),#20659);
#37947=CARTESIAN_POINT ( 'NONE',  ( 3.756430356250000102, 13.09062499938548463, 30.00000000000000000 ) ) ;
#37953=CARTESIAN_POINT ( 'NONE',  ( 0.000000000000000000, 27.50000000000000000, 26.00000000000000000 ) ) ;
#37956=CARTESIAN_POINT ( 'NONE',  ( 1.071796769724500997, 16.90759618943233633, 33.99999999999999289 ) ) ;
#37957=CARTESIAN_POINT ( 'NONE',  ( -1.071796769724491671, 13.92634618820330061, 26.00000000000000355 ) ) ;
#37982=CARTESIAN_POINT ( 'NONE',  ( 1.878215178124997609, 15.26562499938548179, 33.25316411605952993 ) ) ;
#37984=CARTESIAN_POINT ( 'NONE',  ( 4.000000000000000000, 15.65000000000000036, 30.00000000000000000 ) ) ;
#38031=VERTEX_POINT ( 'NONE', #63027 ) ;
#38066=CARTESIAN_POINT ( 'NONE',  ( 1.878215178125000495, 12.82812499938548356, 26.74683588394047007 ) ) ;
#38076=CARTESIAN_POINT ( 'NONE',  ( 1.071796769724495002, 16.40134618820330203, 34.00000000000000000 ) ) ;
#38096=VERTEX_POINT ( 'NONE', #29062 ) ;
#38110=CARTESIAN_POINT ( 'NONE',  ( -1.878215178124999163, 15.15312499938548285, 26.74683588394047007 ) ) ;
#38133=CARTESIAN_POINT ( 'NONE',  ( 5.000000000000000000, 39.99999999999999289, 30.00000000000000000 ) ) ;
#38163=CARTESIAN_POINT ( 'NONE',  ( -7.967954043666661671E-16, 15.67812499938548143, 34.33755215474603517 ) ) ;
#38169=CARTESIAN_POINT ( 'NONE',  ( -3.756430356250000102, 18.71562499938548285, 30.00000000000000000 ) ) ;
#38178=CARTESIAN_POINT ( 'NONE',  ( 3.756430356250000102, 18.94062499938548427, 30.00000000000000000 ) ) ;
#38187=CARTESIAN_POINT ( 'NONE',  ( 1.071796769724495002, 15.10759618943233562, 34.00000000000000000 ) ) ;
#38188=LINE ( 'NONE', #10125, #19331 ) ;
#38193=CARTESIAN_POINT ( 'NONE',  ( 2.000000000000000444, 16.11874999877096570, 26.53589838486224650 ) ) ;
#38236=FACE_OUTER_BOUND ( 'NONE', #9222, .T. ) ;
#38301=CARTESIAN_POINT ( 'NONE',  ( -2.498395430326213790E-14, 17.05624999877096926, 26.00000000000000000 ) ) ;
#38312=CARTESIAN_POINT ( 'NONE',  ( 1.878215178124997609, 13.91562499938548392, 33.25316411605952993 ) ) ;
#38322=CARTESIAN_POINT ( 'NONE',  ( -3.756430356250000990, 13.01562499938548534, 32.16877607737301048 ) ) ;
#38333=VERTEX_POINT ( 'NONE', #57117 ) ;
#38340=CARTESIAN_POINT ( 'NONE',  ( 4.000000000000000000, 19.73749999999999716, 27.69059892324149885 ) ) ;
#38350=CARTESIAN_POINT ( 'NONE',  ( 2.655984681222220721E-16, 14.10312499938548392, 25.66244784525396483 ) ) ;
#38352=CARTESIAN_POINT ( 'NONE',  ( 3.999999999999998668, 16.96249999999999858, 32.30940107675850470 ) ) ;
#38401=CARTESIAN_POINT ( 'NONE',  ( 4.898587196589412829E-16, 27.50000000000000000, 34.00000000000000000 ) ) ;
#38439=CARTESIAN_POINT ( 'NONE',  ( 3.756430356250000546, 15.04062499938548392, 27.83122392262697886 ) ) ;
#38452=VECTOR ( 'NONE', #31319, 1000.000000000000000 ) ;
#38484=CARTESIAN_POINT ( 'NONE',  ( 3.756430356250000102, 18.15312499938548285, 30.00000000000000000 ) ) ;
#38541=CARTESIAN_POINT ( 'NONE',  ( 3.756430356250000102, 14.44062499938548250, 30.00000000000000000 ) ) ;
#38548=CARTESIAN_POINT ( 'NONE',  ( 2.655984681222220721E-16, 19.95312499938548356, 25.66244784525396483 ) ) ;
#38557=CARTESIAN_POINT ( 'NONE',  ( 3.756430356249998770, 18.45312499938548001, 32.16877607737302469 ) ) ;
#38573=CARTESIAN_POINT ( 'NONE',  ( -4.000000000000000888, 15.40624999877096535, 32.30940107675850470 ) ) ;
#38577=ORIENTED_EDGE ( 'NONE', *, *, #20103, .T. ) ;
#38583=CARTESIAN_POINT ( 'NONE',  ( -1.243387493232115393E-14, 16.15624999877096712, 26.00000000000000000 ) ) ;
#38613=ORIENTED_EDGE ( 'NONE', *, *, #71856, .T. ) ;
#38642=CARTESIAN_POINT ( 'NONE',  ( 3.999999999999998668, 17.35624999877096641, 32.30940107675850470 ) ) ;
#38671=AXIS2_PLACEMENT_3D ( 'NONE', #4688, #26115, #54558 ) ;
#38693=CARTESIAN_POINT ( 'NONE',  ( -1.878215178125001827, 14.74062499938548321, 33.25316411605952283 ) ) ;
#38695=CARTESIAN_POINT ( 'NONE',  ( -1.626862140677534273E-15, 17.73124999877096641, 34.00000000000000000 ) ) ;
#38701=CARTESIAN_POINT ( 'NONE',  ( 1.878215178124997609, 15.37812499938548427, 33.25316411605952993 ) ) ;
#38702=CARTESIAN_POINT ( 'NONE',  ( -3.999999999999999112, 13.98124999877096641, 27.69059892324149530 ) ) ;
#38729=CARTESIAN_POINT ( 'NONE',  ( -3.756430356250000102, 15.11562499938548321, 30.00000000000000000 ) ) ;
#38731=CARTESIAN_POINT ( 'NONE',  ( 3.999999999999998668, 16.51249999999999929, 32.30940107675850470 ) ) ;
#38750=CARTESIAN_POINT ( 'NONE',  ( 2.000000000000000444, 20.16874999877096641, 26.53589838486224650 ) ) ;
#38789=DIRECTION ( 'NONE',  ( 0.000000000000000000, 0.000000000000000000, -1.000000000000000000 ) ) ;
#38809=CARTESIAN_POINT ( 'NONE',  ( 0.000000000000000000, 27.50000000000000000, 30.00000000000000000 ) ) ;
#38810=DIRECTION ( 'NONE',  ( 0.000000000000000000, 1.000000000000000000, 0.000000000000000000 ) ) ;
#38814=CARTESIAN_POINT ( 'NONE',  ( 3.756430356249998770, 16.76562499938548356, 32.16877607737302469 ) ) ;
#38857=CARTESIAN_POINT ( 'NONE',  ( 1.878215178124997609, 17.62812499938548427, 33.25316411605952993 ) ) ;
#38864=CARTESIAN_POINT ( 'NONE',  ( 5.000000000000000000, 39.99999999999999289, 15.00000000000000178 ) ) ;
#38878=CARTESIAN_POINT ( 'NONE',  ( -4.000000000000000888, 19.96250000000000213, 32.30940107675850470 ) ) ;
#38898=DIRECTION ( 'NONE',  ( 0.000000000000000000, 0.000000000000000000, -1.000000000000000000 ) ) ;
#38900=ORIENTED_EDGE ( 'NONE', *, *, #10308, .T. ) ;
#38909=CARTESIAN_POINT ( 'NONE',  ( 2.655984681222220721E-16, 15.45312499938548356, 25.66244784525396483 ) ) ;
#38924=CARTESIAN_POINT ( 'NONE',  ( -1.878215178124999163, 19.09062499938548285, 26.74683588394047007 ) ) ;
#38940=CARTESIAN_POINT ( 'NONE',  ( 2.000000000000000444, 19.26874999877096784, 26.53589838486224650 ) ) ;
#38961=APPLICATION_CONTEXT ( 'automotive_design' ) ;
#38962=( BOUNDED_CURVE ( )  B_SPLINE_CURVE ( 2, ( #36957, #59479, #3360, #62578, #13048, #69579, #68857, #62934, #24501 ),
 .UNSPECIFIED., .F., .F. ) 
 B_SPLINE_CURVE_WITH_KNOTS ( ( 3, 2, 2, 2, 3 ),
 ( 0.4861111111111111049, 0.4907407407407407551, 0.5000000000000000000, 0.5092592592592593004, 0.5138888888888889506 ),
 .UNSPECIFIED. ) 
 CURVE ( )  GEOMETRIC_REPRESENTATION_ITEM ( )  RATIONAL_B_SPLINE_CURVE ( ( 0.9330127018922194093, 0.9330127018922194093, 1.000000000000000000, 0.8660254037844387076, 1.000000000000000000, 0.8660254037844387076, 1.000000000000000000, 0.9330127018922185211, 0.9330127018922192983 ) ) 
 REPRESENTATION_ITEM ( '' )  );
#38974=CARTESIAN_POINT ( 'NONE',  ( 0.6522905807966048464, 20.75364847883808395, 33.69936292076899065 ) ) ;
#39008=CARTESIAN_POINT ( 'NONE',  ( 2.000000000000000444, 17.46874999877096712, 26.53589838486224650 ) ) ;
#39009=CARTESIAN_POINT ( 'NONE',  ( 0.6945855708053418898, 20.89427347822356751, 33.93923227099254802 ) ) ;
#39052=CARTESIAN_POINT ( 'NONE',  ( 3.756430356249998770, 13.05312499938548321, 32.16877607737302469 ) ) ;
#39060=CARTESIAN_POINT ( 'NONE',  ( 1.878215178125000495, 14.17812499938548321, 26.74683588394047007 ) ) ;
#39088=CARTESIAN_POINT ( 'NONE',  ( -3.756430356250001434, 15.15312499938548463, 32.16877607737301048 ) ) ;
#39091=CARTESIAN_POINT ( 'NONE',  ( -4.000000000000000888, 16.36250000000000071, 32.30940107675850470 ) ) ;
#39109=CARTESIAN_POINT ( 'NONE',  ( 1.999999999999997335, 20.01874999877096428, 33.46410161513775705 ) ) ;
#39141=EDGE_CURVE ( 'NONE', #16877, #29218, #37136, .T. ) ;
#39172=CARTESIAN_POINT ( 'NONE',  ( 1.878215178124997609, 16.27812499938548285, 33.25316411605952993 ) ) ;
#39183=CARTESIAN_POINT ( 'NONE',  ( 1.999999999999997335, 18.27499999999999858, 33.46410161513775705 ) ) ;
#39219=CARTESIAN_POINT ( 'NONE',  ( -1.878215178124999163, 18.30312499938548143, 26.74683588394047007 ) ) ;
#39271=DIRECTION ( 'NONE',  ( -0.000000000000000000, -1.000000000000000000, -0.000000000000000000 ) ) ;
#39274=CARTESIAN_POINT ( 'NONE',  ( -1.878215178124999163, 15.94062499938548427, 26.74683588394047007 ) ) ;
#39289=CARTESIAN_POINT ( 'NONE',  ( -3.756430356250000102, 19.16562499938548214, 30.00000000000000000 ) ) ;
#39305=CARTESIAN_POINT ( 'NONE',  ( 2.000000000000000444, 18.36874999877096570, 26.53589838486224650 ) ) ;
#39347=DIRECTION ( 'NONE',  ( 1.000000000000000000, 0.000000000000000000, 0.000000000000000000 ) ) ;
#39387=FILL_AREA_STYLE_COLOUR ( '', #34382 ) ;
#39422=CARTESIAN_POINT ( 'NONE',  ( -1.878215178125001827, 15.75312499938548427, 33.25316411605952283 ) ) ;
#39452=CARTESIAN_POINT ( 'NONE',  ( 3.999999999999998668, 18.31250000000000000, 32.30940107675850470 ) ) ;
#39518=( NAMED_UNIT ( * ) SI_UNIT ( $, .STERADIAN. ) SOLID_ANGLE_UNIT ( ) );
#39536=CARTESIAN_POINT ( 'NONE',  ( -7.967954043666661671E-16, 17.14062499938548356, 34.33755215474603517 ) ) ;
#39580=CARTESIAN_POINT ( 'NONE',  ( 1.878215178125000495, 16.87812499938548072, 26.74683588394047007 ) ) ;
#39640=CARTESIAN_POINT ( 'NONE',  ( -1.878215178124999163, 14.14062499938548356, 26.74683588394047007 ) ) ;
#39664=CARTESIAN_POINT ( 'NONE',  ( -1.999999999999999112, 17.09374999877096712, 26.53589838486224650 ) ) ;
#39671=CARTESIAN_POINT ( 'NONE',  ( 4.000000000000000000, 17.39374999877096428, 30.00000000000000000 ) ) ;
#39758=( NAMED_UNIT ( * ) PLANE_ANGLE_UNIT ( ) SI_UNIT ( $, .RADIAN. ) );
#39792=CARTESIAN_POINT ( 'NONE',  ( 3.756430356250000546, 14.59062499938548463, 27.83122392262697886 ) ) ;
#39817=CARTESIAN_POINT ( 'NONE',  ( 4.898587196589412829E-16, 27.50000000000000000, 34.00000000000000000 ) ) ;
#39825=CARTESIAN_POINT ( 'NONE',  ( -4.000000000000000888, 17.71249999999999858, 32.30940107675850470 ) ) ;
#39869=CARTESIAN_POINT ( 'NONE',  ( -1.999999999999999112, 20.24374999877096570, 26.53589838486224650 ) ) ;
#39905=CARTESIAN_POINT ( 'NONE',  ( -1.878215178124999163, 16.05312499938548143, 26.74683588394047007 ) ) ;
#39945=CARTESIAN_POINT ( 'NONE',  ( 2.655984681222220721E-16, 17.81562499938548427, 25.66244784525396483 ) ) ;
#39959=FACE_OUTER_BOUND ( 'NONE', #19285, .T. ) ;
#39982=ORIENTED_EDGE ( 'NONE', *, *, #33073, .F. ) ;
#39998=CARTESIAN_POINT ( 'NONE',  ( -3.756430356250000990, 16.05312499938548143, 32.16877607737301048 ) ) ;
#40031=CARTESIAN_POINT ( 'NONE',  ( 1.999999999999997335, 17.31874999877096499, 33.46410161513775705 ) ) ;
#40041=CYLINDRICAL_SURFACE ( 'NONE', #16769, 4.000000000000000000 ) ;
#40045=ORIENTED_EDGE ( 'NONE', *, *, #19955, .F. ) ;
#40058=CARTESIAN_POINT ( 'NONE',  ( 5.000000000000000000, 39.99999999999999289, 30.00000000000000000 ) ) ;
#40081=EDGE_CURVE ( 'NONE', #50521, #8942, #56628, .T. ) ;
#40118=CARTESIAN_POINT ( 'NONE',  ( 4.000000000000000000, 12.53749999999999964, 27.69059892324149885 ) ) ;
#40149=CARTESIAN_POINT ( 'NONE',  ( 3.756430356249998770, 15.41562499938548392, 32.16877607737301759 ) ) ;
#40180=CARTESIAN_POINT ( 'NONE',  ( 2.828200636599751609E-16, 19.36250000000000426, 25.38119784648299415 ) ) ;
#40215=CARTESIAN_POINT ( 'NONE',  ( -1.626862140677534273E-15, 18.18124999877096215, 34.00000000000000000 ) ) ;
#40217=EDGE_CURVE ( 'NONE', #50573, #15973, #10880, .T. ) ;
#40233=CARTESIAN_POINT ( 'NONE',  ( 1.626862140677534470E-15, 13.28750000000000142, 34.00000000000000000 ) ) ;
#40237=EDGE_CURVE ( 'NONE', #29801, #8994, #43589, .T. ) ;
#40259=CARTESIAN_POINT ( 'NONE',  ( -7.967954043666661671E-16, 17.59062499938548285, 34.33755215474603517 ) ) ;
#40261=CARTESIAN_POINT ( 'NONE',  ( -4.000000000000000000, 13.17500000000000071, 30.00000000000000000 ) ) ;
#40297=CARTESIAN_POINT ( 'NONE',  ( 3.756430356249998770, 19.01562499938548356, 32.16877607737302469 ) ) ;
#40352=CARTESIAN_POINT ( 'NONE',  ( 3.756430356250000102, 17.14062499938548356, 30.00000000000000000 ) ) ;
#40382=CARTESIAN_POINT ( 'NONE',  ( -1.999999999999999112, 17.99374999877096570, 26.53589838486224650 ) ) ;
#40392=CARTESIAN_POINT ( 'NONE',  ( 1.071796769724485232, 16.19240381056766509, 25.99999999999999645 ) ) ;
#40411=CARTESIAN_POINT ( 'NONE',  ( 3.999999999999998668, 14.71250000000000213, 32.30940107675850470 ) ) ;
#40414=CARTESIAN_POINT ( 'NONE',  ( 4.000000000000000000, 12.50000000000000000, 30.00000000000000000 ) ) ;
#40431=VERTEX_POINT ( 'NONE', #341 ) ;
#40445=CARTESIAN_POINT ( 'NONE',  ( 3.756430356250000102, 14.44062499938548250, 30.00000000000000000 ) ) ;
#40465=( BOUNDED_CURVE ( )  B_SPLINE_CURVE ( 2, ( #58599, #19433, #13170, #35710, #36078, #41994, #64514, #13907, #36446 ),
 .UNSPECIFIED., .F., .F. ) 
 B_SPLINE_CURVE_WITH_KNOTS ( ( 3, 2, 2, 2, 3 ),
 ( 0.7916666666666667407, 0.7962962962962962798, 0.8055555555555555802, 0.8148148148148147696, 0.8194444444444444198 ),
 .UNSPECIFIED. ) 
 CURVE ( )  GEOMETRIC_REPRESENTATION_ITEM ( )  RATIONAL_B_SPLINE_CURVE ( ( 0.9330127018922192983, 0.9330127018922200755, 1.000000000000000000, 0.8660254037844387076, 1.000000000000000000, 0.8660254037844387076, 1.000000000000000000, 0.9330127018922194093, 0.9330127018922194093 ) ) 
 REPRESENTATION_ITEM ( '' )  );
#40470=FILL_AREA_STYLE ('',( #39387 ) ) ;
#40485=ADVANCED_FACE ( 'NONE', ( #12858 ), #57916, .T. ) ;
#40508=CARTESIAN_POINT ( 'NONE',  ( 3.756430356250000546, 18.19062499938548427, 27.83122392262697886 ) ) ;
#40528=CARTESIAN_POINT ( 'NONE',  ( 4.898850051585143718E-16, 25.54316770519903557, 34.00000000000000000 ) ) ;
#40539=CARTESIAN_POINT ( 'NONE',  ( -8.484601909799255319E-16, 19.58749999999999858, 34.61880215351700940 ) ) ;
#40575=CARTESIAN_POINT ( 'NONE',  ( 1.071796769724495002, 15.50134618820330168, 34.00000000000000000 ) ) ;
#40586=CARTESIAN_POINT ( 'NONE',  ( 4.000000000000000000, 17.89999999999999858, 30.00000000000000000 ) ) ;
#40622=CARTESIAN_POINT ( 'NONE',  ( 1.878215178125000495, 18.22812499938548214, 26.74683588394047007 ) ) ;
#40624=CARTESIAN_POINT ( 'NONE',  ( 0.6522896842281029617, 20.64114846093740852, 33.69936307885641469 ) ) ;
#40659=CARTESIAN_POINT ( 'NONE',  ( -0.6941636114358130660, 20.72676549290719450, 33.93677660682192965 ) ) ;
#40688=CARTESIAN_POINT ( 'NONE',  ( 1.071796769724490561, 13.25134618820330168, 34.00000000000000000 ) ) ;
#40719=CARTESIAN_POINT ( 'NONE',  ( -1.878215178125001827, 16.09062499938548285, 33.25316411605952283 ) ) ;
#40734=DIRECTION ( 'NONE',  ( -0.000000000000000000, -1.000000000000000000, -0.000000000000000000 ) ) ;
#40747=VECTOR ( 'NONE', #42688, 1000.000000000000000 ) ;
#40751=CARTESIAN_POINT ( 'NONE',  ( 1.878215178124997609, 13.57812499938548356, 33.25316411605952993 ) ) ;
#40814=CARTESIAN_POINT ( 'NONE',  ( -3.756430356250001434, 18.30312499938548143, 32.16877607737301048 ) ) ;
#40835=VECTOR ( 'NONE', #43874, 1000.000000000000000 ) ;
#40841=CARTESIAN_POINT ( 'NONE',  ( -3.999999999999999556, 13.08124999877096606, 27.69059892324149175 ) ) ;
#40845=ORIENTED_EDGE ( 'NONE', *, *, #62835, .T. ) ;
#40875=CARTESIAN_POINT ( 'NONE',  ( -7.967954043666661671E-16, 16.24062499938548143, 34.33755215474603517 ) ) ;
#40911=CARTESIAN_POINT ( 'NONE',  ( 2.929172373741449675, 20.54242198200764946, 33.54521906142198162 ) ) ;
#40990=CARTESIAN_POINT ( 'NONE',  ( 2.655984681222220721E-16, 19.16562499938548214, 25.66244784525396483 ) ) ;
#40992=CARTESIAN_POINT ( 'NONE',  ( -3.999999999999999556, 13.58750000000000213, 27.69059892324149175 ) ) ;
#41029=CARTESIAN_POINT ( 'NONE',  ( -7.967954043666661671E-16, 19.39062499938548001, 34.33755215474603517 ) ) ;
#41033=ADVANCED_FACE ( 'NONE', ( #43131 ), #3477, .T. ) ;
#41054=DIRECTION ( 'NONE',  ( 0.000000000000000000, 0.000000000000000000, -1.000000000000000000 ) ) ;
#41056=VERTEX_POINT ( 'NONE', #24620 ) ;
#41058=CARTESIAN_POINT ( 'NONE',  ( 4.898587196589412829E-16, 27.50000000000000000, 34.00000000000000000 ) ) ;
#41086=CARTESIAN_POINT ( 'NONE',  ( 3.756430356249998770, 18.00312499938548427, 32.16877607737301759 ) ) ;
#41094=( BOUNDED_CURVE ( )  B_SPLINE_CURVE ( 2, ( #62859, #57317, #65780, #42885, #3373, #71701, #25146, #54701, #64679 ),
 .UNSPECIFIED., .F., .F. ) 
 B_SPLINE_CURVE_WITH_KNOTS ( ( 3, 2, 2, 2, 3 ),
 ( 0.3750000000000000000, 0.3796296296296296502, 0.3888888888888888951, 0.3981481481481481399, 0.4027777777777777901 ),
 .UNSPECIFIED. ) 
 CURVE ( )  GEOMETRIC_REPRESENTATION_ITEM ( )  RATIONAL_B_SPLINE_CURVE ( ( 0.9330127018922194093, 0.9330127018922194093, 1.000000000000000000, 0.8660254037844387076, 1.000000000000000000, 0.8660254037844387076, 1.000000000000000000, 0.9330127018922189652, 0.9330127018922194093 ) ) 
 REPRESENTATION_ITEM ( '' )  );
#41108=CARTESIAN_POINT ( 'NONE',  ( 1.071796769724479237, 18.83615380933863293, 25.99999999999999645 ) ) ;
#41115=CARTESIAN_POINT ( 'NONE',  ( -3.756430356249999214, 13.84062499938548463, 27.83122392262697531 ) ) ;
#41141=CARTESIAN_POINT ( 'NONE',  ( -4.000000000000000000, 13.17500000000000071, 30.00000000000000000 ) ) ;
#41142=CARTESIAN_POINT ( 'NONE',  ( 0.000000000000000000, 27.50000000000000000, 30.00000000000000000 ) ) ;
#41149=CARTESIAN_POINT ( 'NONE',  ( 0.6945855708053418898, 20.89427347822356751, 33.93923227099254092 ) ) ;
#41177=CARTESIAN_POINT ( 'NONE',  ( -3.756430356249999214, 16.87812499938548427, 27.83122392262697531 ) ) ;
#41195=CARTESIAN_POINT ( 'NONE',  ( 4.000000000000000000, 17.44999999999999929, 30.00000000000000000 ) ) ;
#41201=CARTESIAN_POINT ( 'NONE',  ( 4.000000000000000000, 14.69374999877096677, 30.00000000000000000 ) ) ;
#41218=DIRECTION ( 'NONE',  ( 1.000000000000000000, 0.000000000000000000, -0.000000000000000000 ) ) ;
#41232=CARTESIAN_POINT ( 'NONE',  ( 1.878215178125000495, 17.32812499938548356, 26.74683588394047007 ) ) ;
#41247=EDGE_CURVE ( 'NONE', #69279, #58357, #5707, .T. ) ;
#41304=CARTESIAN_POINT ( 'NONE',  ( 2.000000000000000444, 15.66874999877096464, 26.53589838486224650 ) ) ;
#41315=CARTESIAN_POINT ( 'NONE',  ( 0.000000000000000000, 27.50000000000000000, 30.00000000000000000 ) ) ;
#41348=CARTESIAN_POINT ( 'NONE',  ( 2.655984681222220721E-16, 17.81562499938548427, 25.66244784525396483 ) ) ;
#41350=CARTESIAN_POINT ( 'NONE',  ( -1.878215178124999163, 20.44062499938548072, 26.74683588394047007 ) ) ;
#41356=CYLINDRICAL_SURFACE ( 'NONE', #64641, 4.000000000000000000 ) ;
#41386=CARTESIAN_POINT ( 'NONE',  ( -1.878215178124999163, 20.55312499938548143, 26.74683588394047007 ) ) ;
#41441=CARTESIAN_POINT ( 'NONE',  ( -3.756430356249999214, 19.12812499938548427, 27.83122392262697176 ) ) ;
#41443=ORIENTED_EDGE ( 'NONE', *, *, #7791, .T. ) ;
#41469=CARTESIAN_POINT ( 'NONE',  ( -0.7391736788420463222, 20.86739049229268161, 34.19204003105966905 ) ) ;
#41478=( BOUNDED_CURVE ( )  B_SPLINE_CURVE ( 2, ( #9394, #38187, #49288, #72181, #66641, #65536, #43007, #60712, #20827 ),
 .UNSPECIFIED., .F., .F. ) 
 B_SPLINE_CURVE_WITH_KNOTS ( ( 3, 2, 2, 2, 3 ),
 ( 0.3194444444444444753, 0.3240740740740740700, 0.3333333333333333148, 0.3425925925925926152, 0.3472222222222222654 ),
 .UNSPECIFIED. ) 
 CURVE ( )  GEOMETRIC_REPRESENTATION_ITEM ( )  RATIONAL_B_SPLINE_CURVE ( ( 0.9330127018922194093, 0.9330127018922197424, 1.000000000000000000, 0.8660254037844387076, 1.000000000000000000, 0.8660254037844387076, 1.000000000000000000, 0.9330127018922189652, 0.9330127018922194093 ) ) 
 REPRESENTATION_ITEM ( '' )  );
#41500=CARTESIAN_POINT ( 'NONE',  ( 5.000000000000000000, 39.99999999999999289, 30.00000000000000000 ) ) ;
#41522=LINE ( 'NONE', #30437, #24209 ) ;
#41530=CARTESIAN_POINT ( 'NONE',  ( -1.878215178125001827, 17.89062499938548356, 33.25316411605952283 ) ) ;
#41547=( BOUNDED_CURVE ( )  B_SPLINE_CURVE ( 2, ( #23679, #40688, #44794, #56581, #34405, #68400, #57659, #35134, #68765 ),
 .UNSPECIFIED., .F., .F. ) 
 B_SPLINE_CURVE_WITH_KNOTS ( ( 3, 2, 2, 2, 3 ),
 ( 0.04166666666666667129, 0.04629629629629629373, 0.05555555555555555247, 0.06481481481481481122, 0.06944444444444444753 ),
 .UNSPECIFIED. ) 
 CURVE ( )  GEOMETRIC_REPRESENTATION_ITEM ( )  RATIONAL_B_SPLINE_CURVE ( ( 0.9330127018922192983, 0.9330127018922194093, 1.000000000000000000, 0.8660254037844387076, 1.000000000000000000, 0.8660254037844387076, 1.000000000000000000, 0.9330127018922191873, 0.9330127018922192983 ) ) 
 REPRESENTATION_ITEM ( '' )  );
#41549=CARTESIAN_POINT ( 'NONE',  ( 4.000000000000000000, 17.48750000000000071, 27.69059892324149885 ) ) ;
#41555=CARTESIAN_POINT ( 'NONE',  ( -4.000000000000000888, 14.05624999877096570, 32.30940107675850470 ) ) ;
#41566=VECTOR ( 'NONE', #71753, 1000.000000000000000 ) ;
#41580=CARTESIAN_POINT ( 'NONE',  ( 5.810221930991193690E-16, 13.96249999999999858, 26.00000000000000000 ) ) ;
#41587=CARTESIAN_POINT ( 'NONE',  ( 3.756430356250000102, 17.70312499938548356, 30.00000000000000000 ) ) ;
#41622=CARTESIAN_POINT ( 'NONE',  ( 3.999999999999998668, 18.76250000000000284, 32.30940107675850470 ) ) ;
#41637=ORIENTED_EDGE ( 'NONE', *, *, #26513, .F. ) ;
#41639=CARTESIAN_POINT ( 'NONE',  ( 2.000000000000000444, 19.71874999877096712, 26.53589838486224650 ) ) ;
#41656=ORIENTED_EDGE ( 'NONE', *, *, #56762, .F. ) ;
#41660=DIRECTION ( 'NONE',  ( 0.000000000000000000, 0.000000000000000000, -1.000000000000000000 ) ) ;
#41700=CARTESIAN_POINT ( 'NONE',  ( 3.756430356249998770, 18.11562499938547788, 32.16877607737302469 ) ) ;
#41702=CARTESIAN_POINT ( 'NONE',  ( 3.999999999999998668, 12.91249999999999964, 32.30940107675850470 ) ) ;
#41707=CARTESIAN_POINT ( 'NONE',  ( -3.999999999999999112, 18.08749999999999858, 27.69059892324149530 ) ) ;
#41713=DIRECTION ( 'NONE',  ( 0.000000000000000000, 0.000000000000000000, 1.000000000000000000 ) ) ;
#41739=CARTESIAN_POINT ( 'NONE',  ( -3.756430356249999214, 20.59062499938548640, 27.83122392262697531 ) ) ;
#41750=EDGE_CURVE ( 'NONE', #7096, #19771, #51024, .T. ) ;
#41778=CARTESIAN_POINT ( 'NONE',  ( -2.008609180075752842, 25.40587078878261096, 33.46894003088245029 ) ) ;
#41794=CARTESIAN_POINT ( 'NONE',  ( -1.878215178124999163, 20.44062499938548072, 26.74683588394047007 ) ) ;
#41824=CARTESIAN_POINT ( 'NONE',  ( -1.999999999999999112, 20.69374999877096499, 26.53589838486224650 ) ) ;
#41840=AXIS2_PLACEMENT_3D ( 'NONE', #7695, #1810, #69406 ) ;
#41869=AXIS2_PLACEMENT_3D ( 'NONE', #38133, #54406, #61034 ) ;
#41883=CARTESIAN_POINT ( 'NONE',  ( 2.655984681222220721E-16, 12.75312499938548427, 25.66244784525396483 ) ) ;
#41890=CARTESIAN_POINT ( 'NONE',  ( -3.756430356249999214, 16.42812499938548143, 27.83122392262697531 ) ) ;
#41900=CARTESIAN_POINT ( 'NONE',  ( 3.756430356250000102, 15.34062499938548285, 30.00000000000000000 ) ) ;
#41916=CARTESIAN_POINT ( 'NONE',  ( 2.828200636599751609E-16, 14.80624999877096570, 25.38119784648299415 ) ) ;
#41920=VERTEX_POINT ( 'NONE', #55993 ) ;
#41938=AXIS2_PLACEMENT_3D ( 'NONE', #18656, #24930, #41218 ) ;
#41953=CARTESIAN_POINT ( 'NONE',  ( 2.655984681222220721E-16, 16.46562499938548285, 25.66244784525396483 ) ) ;
#41958=ORIENTED_EDGE ( 'NONE', *, *, #26495, .F. ) ;
#41970=VERTEX_POINT ( 'NONE', #32361 ) ;
#41991=CARTESIAN_POINT ( 'NONE',  ( -3.999999999999999112, 18.03124999877096712, 27.69059892324149530 ) ) ;
#41994=CARTESIAN_POINT ( 'NONE',  ( -4.000000000000000888, 19.45624999877097139, 32.30940107675850470 ) ) ;
#42008=LINE ( 'NONE', #63796, #13121 ) ;
#42049=CYLINDRICAL_SURFACE ( 'NONE', #41840, 4.000000000000000000 ) ;
#42055=CARTESIAN_POINT ( 'NONE',  ( 4.000000000000000000, 13.43750000000000000, 27.69059892324149885 ) ) ;
#42073=CARTESIAN_POINT ( 'NONE',  ( 1.878215178125000495, 12.71562499938548463, 26.74683588394047007 ) ) ;
#42075=CARTESIAN_POINT ( 'NONE',  ( -4.000000000000000888, 14.11249999999999893, 32.30940107675850470 ) ) ;
#42081=CARTESIAN_POINT ( 'NONE',  ( 5.810221930991193690E-16, 20.20624999877096428, 26.00000000000000000 ) ) ;
#42152=CARTESIAN_POINT ( 'NONE',  ( -3.756430356250000102, 13.42812499938548321, 30.00000000000000000 ) ) ;
#42166=CARTESIAN_POINT ( 'NONE',  ( -3.756430356250000102, 20.51562499938548356, 30.00000000000000000 ) ) ;
#42198=CARTESIAN_POINT ( 'NONE',  ( -4.000000000000000888, 20.80624999877096570, 32.30940107675850470 ) ) ;
#42252=CARTESIAN_POINT ( 'NONE',  ( 3.756430356249998770, 13.05312499938548321, 32.16877607737301759 ) ) ;
#42259=CARTESIAN_POINT ( 'NONE',  ( -1.878215178124999163, 17.74062499938548498, 26.74683588394047007 ) ) ;
#42268=CARTESIAN_POINT ( 'NONE',  ( -3.756430356250000102, 15.56562499938548427, 30.00000000000000000 ) ) ;
#42275=CARTESIAN_POINT ( 'NONE',  ( -1.071796769724496334, 14.88259618943233598, 26.00000000000000355 ) ) ;
#42283=CARTESIAN_POINT ( 'NONE',  ( 2.828200636599751609E-16, 13.45624999877096606, 25.38119784648299415 ) ) ;
#42309=EDGE_CURVE ( 'NONE', #18463, #7096, #68869, .T. ) ;
#42314=CARTESIAN_POINT ( 'NONE',  ( -1.071796769724490561, 12.63259618943233598, 26.00000000000000000 ) ) ;
#42317=CARTESIAN_POINT ( 'NONE',  ( 1.878215178125000495, 20.02812499938548285, 26.74683588394047007 ) ) ;
#42318=FACE_OUTER_BOUND ( 'NONE', #6816, .T. ) ;
#42344=CARTESIAN_POINT ( 'NONE',  ( 5.810221930991193690E-16, 14.35624999877096464, 26.00000000000000000 ) ) ;
#42414=DIRECTION ( 'NONE',  ( -0.000000000000000000, -1.000000000000000000, -0.000000000000000000 ) ) ;
#42439=CARTESIAN_POINT ( 'NONE',  ( 3.756430356249998770, 13.50312499938548250, 32.16877607737302469 ) ) ;
#42441=CARTESIAN_POINT ( 'NONE',  ( -4.000000000000000000, 14.07500000000000107, 30.00000000000000000 ) ) ;
#42491=UNCERTAINTY_MEASURE_WITH_UNIT (LENGTH_MEASURE( 1.000000000000000082E-05 ), #50473, 'distance_accuracy_value', 'NONE');
#42494=CARTESIAN_POINT ( 'NONE',  ( 4.000000000000000000, 12.89374999877096606, 30.00000000000000000 ) ) ;
#42506=CARTESIAN_POINT ( 'NONE',  ( 2.000000000000000444, 20.61874999877096570, 26.53589838486224650 ) ) ;
#42518=CARTESIAN_POINT ( 'NONE',  ( 3.756430356250000546, 14.14062499938548356, 27.83122392262697886 ) ) ;
#42529=CARTESIAN_POINT ( 'NONE',  ( -3.756430356249999214, 18.67812499938548143, 27.83122392262697176 ) ) ;
#42559=CARTESIAN_POINT ( 'NONE',  ( -7.967954043666661671E-16, 16.24062499938548143, 34.33755215474603517 ) ) ;
#42580=ADVANCED_FACE ( 'NONE', ( #66231 ), #59950, .T. ) ;
#42605=DIRECTION ( 'NONE',  ( 0.000000000000000000, 0.000000000000000000, -1.000000000000000000 ) ) ;
#42613=CARTESIAN_POINT ( 'NONE',  ( -1.243387493232115393E-14, 16.60624999877096641, 26.00000000000000000 ) ) ;
#42623=CARTESIAN_POINT ( 'NONE',  ( -7.967954043666661671E-16, 19.27812499938548640, 34.33755215474603517 ) ) ;
#42632=CARTESIAN_POINT ( 'NONE',  ( 3.756430356250000102, 16.69062499938548427, 30.00000000000000000 ) ) ;
#42648=CARTESIAN_POINT ( 'NONE',  ( -3.999999999999999556, 16.23124999877096641, 27.69059892324149175 ) ) ;
#42681=CARTESIAN_POINT ( 'NONE',  ( -1.878215178125001827, 19.80312499938548143, 33.25316411605952283 ) ) ;
#42688=DIRECTION ( 'NONE',  ( 0.000000000000000000, 1.000000000000000000, 0.000000000000000000 ) ) ;
#42714=LINE ( 'NONE', #59316, #19177 ) ;
#42745=DIRECTION ( 'NONE',  ( -0.000000000000000000, -1.000000000000000000, -0.000000000000000000 ) ) ;
#42752=ORIENTED_EDGE ( 'NONE', *, *, #21036, .F. ) ;
#42756=EDGE_CURVE ( 'NONE', #49222, #38333, #15607, .T. ) ;
#42775=CARTESIAN_POINT ( 'NONE',  ( 5.810221930991193690E-16, 17.11249999999999716, 26.00000000000000000 ) ) ;
#42792=CYLINDRICAL_SURFACE ( 'NONE', #49690, 4.000000000000000000 ) ;
#42800=CARTESIAN_POINT ( 'NONE',  ( -7.967954043666661671E-16, 19.84062499938548285, 34.33755215474603517 ) ) ;
#42802=CARTESIAN_POINT ( 'NONE',  ( -8.484601909799255319E-16, 14.63750000000000107, 34.61880215351700940 ) ) ;
#42838=CARTESIAN_POINT ( 'NONE',  ( -4.000000000000000000, 17.67500000000000071, 30.00000000000000000 ) ) ;
#42851=ORIENTED_EDGE ( 'NONE', *, *, #68253, .T. ) ;
#42857=CARTESIAN_POINT ( 'NONE',  ( 4.000000000000000000, 12.93124999877096393, 27.69059892324149885 ) ) ;
#42885=CARTESIAN_POINT ( 'NONE',  ( 3.999999999999998668, 15.61250000000000249, 32.30940107675850470 ) ) ;
#42896=CARTESIAN_POINT ( 'NONE',  ( -3.756430356249999214, 19.57812499938548356, 27.83122392262697176 ) ) ;
#42927=CARTESIAN_POINT ( 'NONE',  ( -3.756430356250000102, 14.77812499938548463, 30.00000000000000000 ) ) ;
#42950=CARTESIAN_POINT ( 'NONE',  ( 1.071796769724488785, 20.05759618943233491, 34.00000000000000000 ) ) ;
#42973=( BOUNDED_CURVE ( )  B_SPLINE_CURVE ( 2, ( #15378, #32749, #26476, #15741, #50109, #26108, #4681, #65628, #44208 ),
 .UNSPECIFIED., .F., .F. ) 
 B_SPLINE_CURVE_WITH_KNOTS ( ( 3, 2, 2, 2, 3 ),
 ( 0.7916666666666667407, 0.7962962962962962798, 0.8055555555555555802, 0.8148148148148147696, 0.8194444444444444198 ),
 .UNSPECIFIED. ) 
 CURVE ( )  GEOMETRIC_REPRESENTATION_ITEM ( )  RATIONAL_B_SPLINE_CURVE ( ( 0.9330127018922192983, 0.9330127018922200755, 1.000000000000000000, 0.8660254037844387076, 1.000000000000000000, 0.8660254037844387076, 1.000000000000000000, 0.9330127018922194093, 0.9330127018922194093 ) ) 
 REPRESENTATION_ITEM ( '' )  );
#42980=CARTESIAN_POINT ( 'NONE',  ( -3.756430356250000102, 12.86562499938548321, 30.00000000000000000 ) ) ;
#42987=CARTESIAN_POINT ( 'NONE',  ( -1.878215178125001827, 19.24062499938548143, 33.25316411605952283 ) ) ;
#42997=CARTESIAN_POINT ( 'NONE',  ( 1.878215178124997609, 17.06562499938548072, 33.25316411605952993 ) ) ;
#43007=CARTESIAN_POINT ( 'NONE',  ( 2.000000000000000444, 15.27500000000000036, 26.53589838486224650 ) ) ;
#43014=CARTESIAN_POINT ( 'NONE',  ( -8.484601909799255319E-16, 17.28124999877096712, 34.61880215351700940 ) ) ;
#43043=( BOUNDED_CURVE ( )  B_SPLINE_CURVE ( 2, ( #44735, #67269, #39183, #61698, #11097, #56169, #24982, #71153, #70056 ),
 .UNSPECIFIED., .F., .F. ) 
 B_SPLINE_CURVE_WITH_KNOTS ( ( 3, 2, 2, 2, 3 ),
 ( 0.7083333333333333703, 0.7129629629629629095, 0.7222222222222222099, 0.7314814814814815103, 0.7361111111111111605 ),
 .UNSPECIFIED. ) 
 CURVE ( )  GEOMETRIC_REPRESENTATION_ITEM ( )  RATIONAL_B_SPLINE_CURVE ( ( 0.9330127018922192983, 0.9330127018922200755, 1.000000000000000000, 0.8660254037844387076, 1.000000000000000000, 0.8660254037844387076, 1.000000000000000000, 0.9330127018922185211, 0.9330127018922192983 ) ) 
 REPRESENTATION_ITEM ( '' )  );
#43047=CARTESIAN_POINT ( 'NONE',  ( -3.756430356250000990, 18.41562499938548214, 32.16877607737301048 ) ) ;
#43058=CARTESIAN_POINT ( 'NONE',  ( -3.999999999999999112, 20.33749999999999858, 27.69059892324149530 ) ) ;
#43074=CARTESIAN_POINT ( 'NONE',  ( 2.000000000000000444, 14.31874999877096499, 26.53589838486224650 ) ) ;
#43113=AXIS2_PLACEMENT_3D ( 'NONE', #6165, #51601, #45699 ) ;
#43118=ORIENTED_EDGE ( 'NONE', *, *, #52890, .F. ) ;
#43123=CARTESIAN_POINT ( 'NONE',  ( 3.999999999999998668, 16.90624999877096712, 32.30940107675850470 ) ) ;
#43131=FACE_OUTER_BOUND ( 'NONE', #44641, .T. ) ;
#43137=ADVANCED_FACE ( 'NONE', ( #72503 ), #27449, .T. ) ;
#43141=CARTESIAN_POINT ( 'NONE',  ( -1.878215178125001827, 13.50312499938548427, 33.25316411605952283 ) ) ;
#43174=CARTESIAN_POINT ( 'NONE',  ( 1.878215178125000495, 13.61562499938548321, 26.74683588394047007 ) ) ;
#43176=CARTESIAN_POINT ( 'NONE',  ( -4.000000000000000000, 15.42500000000000071, 30.00000000000000000 ) ) ;
#43189=EDGE_LOOP ( 'NONE', ( #4205, #49067, #66619, #44739 ) ) ;
#43211=EDGE_LOOP ( 'NONE', ( #37371, #57641, #50808, #11853 ) ) ;
#43259=CARTESIAN_POINT ( 'NONE',  ( -7.967954043666661671E-16, 13.09062499938548285, 34.33755215474603517 ) ) ;
#43266=( BOUNDED_CURVE ( )  B_SPLINE_CURVE ( 2, ( #18606, #51886, #18236 ),
 .UNSPECIFIED., .F., .F. ) 
 B_SPLINE_CURVE_WITH_KNOTS ( ( 3, 3 ),
 ( 0.9861111111111111605, 0.9876227234888749207 ),
 .UNSPECIFIED. ) 
 CURVE ( )  GEOMETRIC_REPRESENTATION_ITEM ( )  RATIONAL_B_SPLINE_CURVE ( ( 0.9330127018922194093, 0.9330127018922196314, 0.9401540605060327849 ) ) 
 REPRESENTATION_ITEM ( '' )  );
#43301=AXIS2_PLACEMENT_3D ( 'NONE', #8042, #7316, #41660 ) ;
#43303=CARTESIAN_POINT ( 'NONE',  ( 3.756430356250000546, 15.04062499938548392, 27.83122392262697886 ) ) ;
#43327=CARTESIAN_POINT ( 'NONE',  ( -1.999999999999999112, 13.49374999877096570, 26.53589838486224650 ) ) ;
#43357=CARTESIAN_POINT ( 'NONE',  ( 5.810221930991193690E-16, 13.96249999999999858, 26.00000000000000000 ) ) ;
#43364=CARTESIAN_POINT ( 'NONE',  ( -3.756430356249999214, 20.47812499938548214, 27.83122392262697531 ) ) ;
#43373=CARTESIAN_POINT ( 'NONE',  ( -1.878215178124999163, 17.29062499938548214, 26.74683588394047007 ) ) ;
#43388=CARTESIAN_POINT ( 'NONE',  ( -4.000000000000000888, 16.75624999877096855, 32.30940107675850470 ) ) ;
#43422=CARTESIAN_POINT ( 'NONE',  ( -3.756430356250000102, 18.82812499938548356, 30.00000000000000000 ) ) ;
#43423=DIRECTION ( 'NONE',  ( -0.000000000000000000, -1.000000000000000000, -0.000000000000000000 ) ) ;
#43439=ORIENTED_EDGE ( 'NONE', *, *, #72495, .F. ) ;
#43457=CARTESIAN_POINT ( 'NONE',  ( -2.000000000000001776, 19.54999999999999716, 33.46410161513775705 ) ) ;
#43470=CARTESIAN_POINT ( 'NONE',  ( -5.000000000000000000, 39.99999999999999289, 30.00000000000000000 ) ) ;
#43502=CARTESIAN_POINT ( 'NONE',  ( 3.756430356250000546, 13.12812499938548250, 27.83122392262697886 ) ) ;
#43535=ORIENTED_EDGE ( 'NONE', *, *, #60834, .T. ) ;
#43539=CARTESIAN_POINT ( 'NONE',  ( -7.967954043666661671E-16, 13.87812499938548250, 34.33755215474603517 ) ) ;
#43541=CARTESIAN_POINT ( 'NONE',  ( 2.000000000000000444, 16.17500000000000071, 26.53589838486224650 ) ) ;
#43576=VERTEX_POINT ( 'NONE', #58391 ) ;
#43587=ORIENTED_EDGE ( 'NONE', *, *, #48200, .T. ) ;
#43589=LINE ( 'NONE', #38401, #37204 ) ;
#43615=CARTESIAN_POINT ( 'NONE',  ( -2.000000000000001776, 15.94999999999999929, 33.46410161513775705 ) ) ;
#43624=CARTESIAN_POINT ( 'NONE',  ( -3.756430356250000102, 14.32812499938548356, 30.00000000000000000 ) ) ;
#43645=CARTESIAN_POINT ( 'NONE',  ( 2.000000000000000444, 14.76874999877096606, 26.53589838486224650 ) ) ;
#43653=ORIENTED_EDGE ( 'NONE', *, *, #72942, .T. ) ;
#43667=CARTESIAN_POINT ( 'NONE',  ( -7.967954043666661671E-16, 14.89062499938548179, 34.33755215474603517 ) ) ;
#43691=DIRECTION ( 'NONE',  ( 0.000000000000000000, 0.000000000000000000, -1.000000000000000000 ) ) ;
#43707=DIRECTION ( 'NONE',  ( 0.000000000000000000, 0.000000000000000000, -1.000000000000000000 ) ) ;
#43710=CARTESIAN_POINT ( 'NONE',  ( -4.000000000000000888, 19.90624999877096712, 32.30940107675850470 ) ) ;
#43720=CARTESIAN_POINT ( 'NONE',  ( 3.756430356250000546, 14.92812499938548321, 27.83122392262697886 ) ) ;
#43723=ORIENTED_EDGE ( 'NONE', *, *, #29408, .T. ) ;
#43726=CARTESIAN_POINT ( 'NONE',  ( -3.756430356250001434, 19.65312499938548640, 32.16877607737301048 ) ) ;
#43735=CARTESIAN_POINT ( 'NONE',  ( 1.878215178124997609, 17.96562499938548285, 33.25316411605952993 ) ) ;
#43751=CARTESIAN_POINT ( 'NONE',  ( 4.000000000000000000, 15.59374999877096535, 30.00000000000000000 ) ) ;
#43763=EDGE_CURVE ( 'NONE', #25000, #50521, #41094, .T. ) ;
#43784=CARTESIAN_POINT ( 'NONE',  ( -1.878215178124999163, 18.75312499938548427, 26.74683588394047007 ) ) ;
#43785=CYLINDRICAL_SURFACE ( 'NONE', #64176, 4.000000000000000000 ) ;
#43795=ADVANCED_FACE ( 'NONE', ( #31060 ), #17975, .T. ) ;
#43804=CARTESIAN_POINT ( 'NONE',  ( 2.000000000000000444, 19.32500000000000284, 26.53589838486224650 ) ) ;
#43864=( BOUNDED_CURVE ( )  B_SPLINE_CURVE ( 2, ( #38583, #65921, #26772, #32303, #60360, #31939, #21577, #32672, #4606 ),
 .UNSPECIFIED., .F., .F. ) 
 B_SPLINE_CURVE_WITH_KNOTS ( ( 3, 2, 2, 2, 3 ),
 ( 0.4027777777777777901, 0.4074074074074073848, 0.4166666666666666852, 0.4259259259259259300, 0.4305555555555555802 ),
 .UNSPECIFIED. ) 
 CURVE ( )  GEOMETRIC_REPRESENTATION_ITEM ( )  RATIONAL_B_SPLINE_CURVE ( ( 0.9330127018922194093, 0.9330127018922197424, 1.000000000000000000, 0.8660254037844387076, 1.000000000000000000, 0.8660254037844387076, 1.000000000000000000, 0.9330127018922189652, 0.9330127018922194093 ) ) 
 REPRESENTATION_ITEM ( '' )  );
#43869=CARTESIAN_POINT ( 'NONE',  ( 1.878215178124997609, 13.46562499938548285, 33.25316411605952993 ) ) ;
#43874=DIRECTION ( 'NONE',  ( -0.000000000000000000, -1.000000000000000000, -0.000000000000000000 ) ) ;
#43877=CARTESIAN_POINT ( 'NONE',  ( -3.756430356249999214, 12.94062499938548427, 27.83122392262697176 ) ) ;
#43890=ORIENTED_EDGE ( 'NONE', *, *, #59196, .F. ) ;
#43907=CARTESIAN_POINT ( 'NONE',  ( -1.878215178124999163, 15.49062499938548321, 26.74683588394047007 ) ) ;
#43909=CARTESIAN_POINT ( 'NONE',  ( -3.999999999999999556, 16.28749999999999787, 27.69059892324149175 ) ) ;
#43956=CARTESIAN_POINT ( 'NONE',  ( -3.486133158594716510E-16, 13.00624999877096855, 26.00000000000000355 ) ) ;
#43970=LINE ( 'NONE', #9976, #61862 ) ;
#43972=CARTESIAN_POINT ( 'NONE',  ( 0.000000000000000000, 27.50000000000000000, 30.00000000000000000 ) ) ;
#43986=CARTESIAN_POINT ( 'NONE',  ( 2.000000000000000444, 17.91874999877096641, 26.53589838486224650 ) ) ;
#43991=CARTESIAN_POINT ( 'NONE',  ( 3.756430356250000102, 15.00312499938548427, 30.00000000000000000 ) ) ;
#44033=CARTESIAN_POINT ( 'NONE',  ( -3.756430356250001434, 14.81562499938548250, 32.16877607737301048 ) ) ;
#44089=CARTESIAN_POINT ( 'NONE',  ( 1.878215178124997609, 15.26562499938548179, 33.25316411605952993 ) ) ;
#44095=CARTESIAN_POINT ( 'NONE',  ( -1.878215178124999163, 19.54062499938548214, 26.74683588394047007 ) ) ;
#44105=CARTESIAN_POINT ( 'NONE',  ( -3.756430356250001434, 17.40312499938548285, 32.16877607737301048 ) ) ;
#44121=CARTESIAN_POINT ( 'NONE',  ( 4.000000000000000000, 16.98124999877096641, 27.69059892324149530 ) ) ;
#44171=EDGE_CURVE ( 'NONE', #65514, #50573, #11823, .T. ) ;
#44187=CARTESIAN_POINT ( 'NONE',  ( -2.000000000000001776, 14.99374999877096570, 33.46410161513775705 ) ) ;
#44208=CARTESIAN_POINT ( 'NONE',  ( -1.626862140677534273E-15, 19.13749999999999929, 34.00000000000000000 ) ) ;
#44237=CARTESIAN_POINT ( 'NONE',  ( -3.756430356250001434, 12.90312499938548463, 32.16877607737301048 ) ) ;
#44243=CARTESIAN_POINT ( 'NONE',  ( 2.393811435568372112E-14, 18.63124999877096855, 34.00000000000000000 ) ) ;
#44246=CARTESIAN_POINT ( 'NONE',  ( 1.878215178125000495, 14.62812499938548427, 26.74683588394047007 ) ) ;
#44247=CARTESIAN_POINT ( 'NONE',  ( -1.071796769724496334, 15.27634618820330026, 26.00000000000000355 ) ) ;
#44275=CARTESIAN_POINT ( 'NONE',  ( -3.756430356250000102, 15.56562499938548427, 30.00000000000000000 ) ) ;
#44277=CARTESIAN_POINT ( 'NONE',  ( -1.999999999999999112, 16.69999999999999929, 26.53589838486224650 ) ) ;
#44305=( BOUNDED_CURVE ( )  B_SPLINE_CURVE ( 2, ( #46009, #46734, #58514, #59614, #24906, #24547, #47817, #59246, #8654 ),
 .UNSPECIFIED., .F., .F. ) 
 B_SPLINE_CURVE_WITH_KNOTS ( ( 3, 2, 2, 2, 3 ),
 ( 0.1250000000000000000, 0.1296296296296296224, 0.1388888888888888951, 0.1481481481481481399, 0.1527777777777777901 ),
 .UNSPECIFIED. ) 
 CURVE ( )  GEOMETRIC_REPRESENTATION_ITEM ( )  RATIONAL_B_SPLINE_CURVE ( ( 0.9330127018922192983, 0.9330127018922194093, 1.000000000000000000, 0.8660254037844387076, 1.000000000000000000, 0.8660254037844387076, 1.000000000000000000, 0.9330127018922191873, 0.9330127018922194093 ) ) 
 REPRESENTATION_ITEM ( '' )  );
#44311=ORIENTED_EDGE ( 'NONE', *, *, #47391, .F. ) ;
#44323=CARTESIAN_POINT ( 'NONE',  ( -4.000000000000000888, 20.35624999877096641, 32.30940107675850470 ) ) ;
#44360=CARTESIAN_POINT ( 'NONE',  ( 4.000000000000000000, 17.88124999877096855, 27.69059892324149885 ) ) ;
#44364=CARTESIAN_POINT ( 'NONE',  ( -1.878215178125001827, 15.75312499938548427, 33.25316411605952283 ) ) ;
#44376=FACE_OUTER_BOUND ( 'NONE', #60541, .T. ) ;
#44408=CARTESIAN_POINT ( 'NONE',  ( 3.756430356249998770, 18.56562499938548427, 32.16877607737302469 ) ) ;
#44431=CARTESIAN_POINT ( 'NONE',  ( -4.000000000000000000, 13.56874999877096677, 30.00000000000000000 ) ) ;
#44445=CARTESIAN_POINT ( 'NONE',  ( -1.626862140677534273E-15, 15.93124999877096748, 34.00000000000000000 ) ) ;
#44461=CARTESIAN_POINT ( 'NONE',  ( -3.756430356250000102, 15.11562499938548321, 30.00000000000000000 ) ) ;
#44464=ORIENTED_EDGE ( 'NONE', *, *, #14707, .F. ) ;
#44477=CARTESIAN_POINT ( 'NONE',  ( -3.756430356249999214, 18.22812499938548214, 27.83122392262697531 ) ) ;
#44492=CARTESIAN_POINT ( 'NONE',  ( 2.000000000000000444, 17.91874999877096641, 26.53589838486224650 ) ) ;
#44495=CARTESIAN_POINT ( 'NONE',  ( 1.999999999999997335, 12.87500000000000178, 33.46410161513775705 ) ) ;
#44537=CARTESIAN_POINT ( 'NONE',  ( -4.000000000000000000, 20.37500000000000000, 30.00000000000000000 ) ) ;
#44604=EDGE_CURVE ( 'NONE', #24717, #68198, #58100, .T. ) ;
#44609=CARTESIAN_POINT ( 'NONE',  ( -1.878215178124999163, 13.69062499938548427, 26.74683588394047007 ) ) ;
#44617=CARTESIAN_POINT ( 'NONE',  ( 3.756430356249998770, 14.96562499938548108, 32.16877607737301759 ) ) ;
#44618=CARTESIAN_POINT ( 'NONE',  ( -4.000000000000000888, 14.05624999877096748, 32.30940107675850470 ) ) ;
#44641=EDGE_LOOP ( 'NONE', ( #21447, #52564, #2251, #50364, #43535, #70915, #55600, #72011, #59225, #21246, #3914, #49947, #17031, #5808, #47621, #67190, #16029, #6535, #13939, #53046, #14149, #16077, #41443, #50698, #34231, #70050, #55161, #25390, #22818, #59573, #43653, #27451, #64858, #842, #4881, #68653, #19681, #57182, #47507, #28043 ) ) ;
#44644=CARTESIAN_POINT ( 'NONE',  ( 1.878215178125000495, 15.86562499938548321, 26.74683588394047007 ) ) ;
#44647=CARTESIAN_POINT ( 'NONE',  ( 3.999999999999998668, 17.86250000000000071, 32.30940107675850470 ) ) ;
#44724=CARTESIAN_POINT ( 'NONE',  ( 1.878215178125000495, 16.87812499938548072, 26.74683588394047007 ) ) ;
#44735=CARTESIAN_POINT ( 'NONE',  ( 2.393811435568372112E-14, 18.23750000000000071, 34.00000000000000000 ) ) ;
#44739=ORIENTED_EDGE ( 'NONE', *, *, #49591, .T. ) ;
#44768=CARTESIAN_POINT ( 'NONE',  ( -3.756430356250001434, 17.51562499938548356, 32.16877607737301048 ) ) ;
#44794=CARTESIAN_POINT ( 'NONE',  ( 1.999999999999997335, 13.26874999877096606, 33.46410161513775705 ) ) ;
#44821=CARTESIAN_POINT ( 'NONE',  ( 1.878215178124997609, 15.71562499938548108, 33.25316411605952993 ) ) ;
#44824=VERTEX_POINT ( 'NONE', #63147 ) ;
#44836=CARTESIAN_POINT ( 'NONE',  ( -1.878215178125001827, 18.79062499938548214, 33.25316411605952283 ) ) ;
#44844=CARTESIAN_POINT ( 'NONE',  ( -1.071796769724480347, 17.26115380933863008, 34.00000000000000711 ) ) ;
#44850=CARTESIAN_POINT ( 'NONE',  ( 2.828200636599751609E-16, 17.95624999877096784, 25.38119784648299415 ) ) ;
#44853=CARTESIAN_POINT ( 'NONE',  ( -4.000000000000000888, 17.65624999877096712, 32.30940107675850470 ) ) ;
#44898=ORIENTED_EDGE ( 'NONE', *, *, #71305, .F. ) ;
#44960=LINE ( 'NONE', #21682, #25247 ) ;
#44965=CARTESIAN_POINT ( 'NONE',  ( -7.967954043666661671E-16, 15.34062499938548108, 34.33755215474603517 ) ) ;
#44966=DIRECTION ( 'NONE',  ( -0.000000000000000000, -1.000000000000000000, -0.000000000000000000 ) ) ;
#44997=CARTESIAN_POINT ( 'NONE',  ( -4.000000000000000888, 17.26249999999999929, 32.30940107675850470 ) ) ;
#45011=VERTEX_POINT ( 'NONE', #25818 ) ;
#45034=FACE_OUTER_BOUND ( 'NONE', #69594, .T. ) ;
#45077=CARTESIAN_POINT ( 'NONE',  ( -3.756430356250001434, 16.61562499938548143, 32.16877607737301048 ) ) ;
#45087=CARTESIAN_POINT ( 'NONE',  ( 0.6945855708053418898, 20.89427347822356751, 33.93923227099254092 ) ) ;
#45120=CARTESIAN_POINT ( 'NONE',  ( -7.967954043666661671E-16, 16.69062499938548427, 34.33755215474603517 ) ) ;
#45150=( BOUNDED_CURVE ( )  B_SPLINE_CURVE ( 2, ( #23131, #50502, #6153, #28682, #625, #50861, #45687, #68578, #41580 ),
 .UNSPECIFIED., .F., .F. ) 
 B_SPLINE_CURVE_WITH_KNOTS ( ( 3, 2, 2, 2, 3 ),
 ( 0.1527777777777777901, 0.1574074074074074125, 0.1666666666666666574, 0.1759259259259259300, 0.1805555555555555525 ),
 .UNSPECIFIED. ) 
 CURVE ( )  GEOMETRIC_REPRESENTATION_ITEM ( )  RATIONAL_B_SPLINE_CURVE ( ( 0.9330127018922194093, 0.9330127018922195203, 1.000000000000000000, 0.8660254037844387076, 1.000000000000000000, 0.8660254037844387076, 1.000000000000000000, 0.9330127018922194093, 0.9330127018922194093 ) ) 
 REPRESENTATION_ITEM ( '' )  );
#45158=ORIENTED_EDGE ( 'NONE', *, *, #14707, .T. ) ;
#45160=CARTESIAN_POINT ( 'NONE',  ( -1.243387493232115393E-14, 15.70624999877096784, 26.00000000000000000 ) ) ;
#45176=CARTESIAN_POINT ( 'NONE',  ( 1.878215178124997609, 13.91562499938548392, 33.25316411605952993 ) ) ;
#45178=FACE_OUTER_BOUND ( 'NONE', #49424, .T. ) ;
#45191=CARTESIAN_POINT ( 'NONE',  ( -3.756430356250001434, 17.85312499938548214, 32.16877607737301048 ) ) ;
#45206=CARTESIAN_POINT ( 'NONE',  ( -4.000000000000000000, 18.06874999877096855, 30.00000000000000000 ) ) ;
#45218=( BOUNDED_CURVE ( )  B_SPLINE_CURVE ( 2, ( #43357, #53331, #70685, #13804, #20802, #19328, #25990, #37799, #60319 ),
 .UNSPECIFIED., .F., .F. ) 
 B_SPLINE_CURVE_WITH_KNOTS ( ( 3, 2, 2, 2, 3 ),
 ( 0.1805555555555555525, 0.1851851851851851749, 0.1944444444444444475, 0.2037037037037036924, 0.2083333333333333426 ),
 .UNSPECIFIED. ) 
 CURVE ( )  GEOMETRIC_REPRESENTATION_ITEM ( )  RATIONAL_B_SPLINE_CURVE ( ( 0.9330127018922194093, 0.9330127018922194093, 1.000000000000000000, 0.8660254037844387076, 1.000000000000000000, 0.8660254037844387076, 1.000000000000000000, 0.9330127018922191873, 0.9330127018922194093 ) ) 
 REPRESENTATION_ITEM ( '' )  );
#45288=CYLINDRICAL_SURFACE ( 'NONE', #49013, 4.000000000000000000 ) ;
#45298=ORIENTED_EDGE ( 'NONE', *, *, #44604, .F. ) ;
#45325=CARTESIAN_POINT ( 'NONE',  ( 3.756430356250000546, 15.04062499938548392, 27.83122392262697886 ) ) ;
#45357=CARTESIAN_POINT ( 'NONE',  ( -4.000000000000000000, 18.57500000000000284, 30.00000000000000000 ) ) ;
#45376=CARTESIAN_POINT ( 'NONE',  ( 5.810221930991193690E-16, 20.20624999877096428, 26.00000000000000000 ) ) ;
#45440=CARTESIAN_POINT ( 'NONE',  ( 1.878215178124997609, 14.92812499938548321, 33.25316411605952993 ) ) ;
#45483=CARTESIAN_POINT ( 'NONE',  ( -3.756430356249999214, 17.89062499938548356, 27.83122392262697531 ) ) ;
#45524=ORIENTED_EDGE ( 'NONE', *, *, #17942, .T. ) ;
#45543=CARTESIAN_POINT ( 'NONE',  ( -7.967954043666661671E-16, 17.02812499938548285, 34.33755215474603517 ) ) ;
#45574=CARTESIAN_POINT ( 'NONE',  ( -4.000000000000000000, 18.51874999877096784, 30.00000000000000000 ) ) ;
#45583=CARTESIAN_POINT ( 'NONE',  ( 1.999999999999997335, 16.02500000000000213, 33.46410161513775705 ) ) ;
#45601=CARTESIAN_POINT ( 'NONE',  ( 5.810221930991193690E-16, 18.40624999877096357, 26.00000000000000000 ) ) ;
#45687=CARTESIAN_POINT ( 'NONE',  ( 2.000000000000000444, 13.92500000000000071, 26.53589838486224650 ) ) ;
#45693=CARTESIAN_POINT ( 'NONE',  ( 1.878215178125000495, 15.07812499938548179, 26.74683588394047007 ) ) ;
#45699=DIRECTION ( 'NONE',  ( 0.000000000000000000, -0.000000000000000000, 1.000000000000000000 ) ) ;
#45723=CARTESIAN_POINT ( 'NONE',  ( 4.000000000000000000, 20.18750000000000000, 27.69059892324149530 ) ) ;
#45802=CARTESIAN_POINT ( 'NONE',  ( 1.878215178125000495, 18.67812499938548143, 26.74683588394047007 ) ) ;
#45804=CARTESIAN_POINT ( 'NONE',  ( -1.999999999999999112, 13.10000000000000142, 26.53589838486224650 ) ) ;
#45811=CARTESIAN_POINT ( 'NONE',  ( -1.626862140677534273E-15, 16.43750000000000000, 34.00000000000000000 ) ) ;
#45840=CARTESIAN_POINT ( 'NONE',  ( 3.756430356250000102, 16.35312499938548569, 30.00000000000000000 ) ) ;
#45857=( BOUNDED_CURVE ( )  B_SPLINE_CURVE ( 2, ( #56014, #40118, #62989, #17201, #12384 ),
 .UNSPECIFIED., .F., .F. ) 
 B_SPLINE_CURVE_WITH_KNOTS ( ( 3, 2, 3 ),
 ( 0.000000000000000000, 0.009259259259259258745, 0.01388888888888888985 ),
 .UNSPECIFIED. ) 
 CURVE ( )  GEOMETRIC_REPRESENTATION_ITEM ( )  RATIONAL_B_SPLINE_CURVE ( ( 1.000000000000000000, 0.8660254037844387076, 1.000000000000000000, 0.9330127018922192983, 0.9330127018922194093 ) ) 
 REPRESENTATION_ITEM ( '' )  );
#45894=EDGE_CURVE ( 'NONE', #38096, #7083, #20849, .T. ) ;
#45898=CARTESIAN_POINT ( 'NONE',  ( 3.756430356250000102, 16.24062499938548143, 30.00000000000000000 ) ) ;
#45927=CARTESIAN_POINT ( 'NONE',  ( -4.000000000000000000, 19.41874999877096641, 30.00000000000000000 ) ) ;
#45983=CARTESIAN_POINT ( 'NONE',  ( -1.071796769724480347, 19.06115380933863435, 34.00000000000000711 ) ) ;
#45987=CARTESIAN_POINT ( 'NONE',  ( -7.967954043666661671E-16, 14.32812499938548179, 34.33755215474603517 ) ) ;
#46009=CARTESIAN_POINT ( 'NONE',  ( -2.672702088255949472E-15, 13.51250000000000107, 26.00000000000000000 ) ) ;
#46012=DIRECTION ( 'NONE',  ( 1.000000000000000000, 0.000000000000000000, 0.000000000000000000 ) ) ;
#46020=VERTEX_POINT ( 'NONE', #36466 ) ;
#46050=CARTESIAN_POINT ( 'NONE',  ( -3.756430356250000990, 17.96562499938548285, 32.16877607737301048 ) ) ;
#46064=ORIENTED_EDGE ( 'NONE', *, *, #26971, .T. ) ;
#46076=VERTEX_POINT ( 'NONE', #24645 ) ;
#46082=CARTESIAN_POINT ( 'NONE',  ( 3.999999999999998668, 20.11249999999999716, 32.30940107675850470 ) ) ;
#46118=CARTESIAN_POINT ( 'NONE',  ( 1.071796769724485232, 15.68615380933863257, 25.99999999999999645 ) ) ;
#46161=CARTESIAN_POINT ( 'NONE',  ( 3.756430356250000546, 17.29062499938548214, 27.83122392262697886 ) ) ;
#46163=CARTESIAN_POINT ( 'NONE',  ( -3.756430356249999214, 20.47812499938548214, 27.83122392262697531 ) ) ;
#46199=CARTESIAN_POINT ( 'NONE',  ( -7.967954043666661671E-16, 18.94062499938548783, 34.33755215474603517 ) ) ;
#46204=STYLED_ITEM ( 'NONE', ( #12380 ), #30285 ) ;
#46217=SHAPE_REPRESENTATION ( 'pressure gauge', ( #23765 ), #24934 ) ;
#46226=CARTESIAN_POINT ( 'NONE',  ( 2.000000000000000444, 15.21874999877096535, 26.53589838486224650 ) ) ;
#46243=DIRECTION ( 'NONE',  ( -0.000000000000000000, -1.000000000000000000, -0.000000000000000000 ) ) ;
#46257=CARTESIAN_POINT ( 'NONE',  ( -7.967954043666661671E-16, 17.47812499938548214, 34.33755215474603517 ) ) ;
#46274=EDGE_LOOP ( 'NONE', ( #68599, #28998, #24532, #51521 ) ) ;
#46284=CARTESIAN_POINT ( 'NONE',  ( -8.484601909799255319E-16, 19.98124999877096641, 34.61880215351700940 ) ) ;
#46298=ORIENTED_EDGE ( 'NONE', *, *, #25301, .T. ) ;
#46313=FACE_OUTER_BOUND ( 'NONE', #66611, .T. ) ;
#46315=CARTESIAN_POINT ( 'NONE',  ( -1.626862140677534273E-15, 14.63749999999999929, 34.00000000000000000 ) ) ;
#46350=CARTESIAN_POINT ( 'NONE',  ( -3.756430356250001434, 17.40312499938548285, 32.16877607737301048 ) ) ;
#46380=ORIENTED_EDGE ( 'NONE', *, *, #42309, .F. ) ;
#46409=CARTESIAN_POINT ( 'NONE',  ( -1.878215178124999163, 18.30312499938548143, 26.74683588394047007 ) ) ;
#46413=ORIENTED_EDGE ( 'NONE', *, *, #22559, .T. ) ;
#46443=CARTESIAN_POINT ( 'NONE',  ( -4.000000000000000888, 20.41250000000000142, 32.30940107675850470 ) ) ;
#46488=DIRECTION ( 'NONE',  ( -0.000000000000000000, -1.000000000000000000, -0.000000000000000000 ) ) ;
#46523=CARTESIAN_POINT ( 'NONE',  ( 1.878215178124997609, 18.07812499938548356, 33.25316411605952993 ) ) ;
#46525=CARTESIAN_POINT ( 'NONE',  ( 2.000000000000000444, 13.02500000000000036, 26.53589838486224650 ) ) ;
#46530=CARTESIAN_POINT ( 'NONE',  ( -2.000000000000001776, 18.19999999999999929, 33.46410161513775705 ) ) ;
#46562=CARTESIAN_POINT ( 'NONE',  ( 2.655984681222220721E-16, 20.51562499938548356, 25.66244784525396483 ) ) ;
#46592=CARTESIAN_POINT ( 'NONE',  ( 1.999999999999997335, 20.46874999877096712, 33.46410161513775705 ) ) ;
#46618=CARTESIAN_POINT ( 'NONE',  ( -7.967954043666661671E-16, 17.92812499938548498, 34.33755215474603517 ) ) ;
#46650=CARTESIAN_POINT ( 'NONE',  ( -3.756430356250000102, 13.87812499938548250, 30.00000000000000000 ) ) ;
#46715=CARTESIAN_POINT ( 'NONE',  ( -3.756430356250000102, 18.26562499938548356, 30.00000000000000000 ) ) ;
#46734=CARTESIAN_POINT ( 'NONE',  ( -1.071796769724491671, 13.53259618943233633, 26.00000000000000355 ) ) ;
#46741=CARTESIAN_POINT ( 'NONE',  ( -4.000000000000000888, 13.60624999877096641, 32.30940107675850470 ) ) ;
#46773=CARTESIAN_POINT ( 'NONE',  ( -3.756430356250000990, 16.61562499938548143, 32.16877607737301048 ) ) ;
#46778=ORIENTED_EDGE ( 'NONE', *, *, #1971, .F. ) ;
#46807=CARTESIAN_POINT ( 'NONE',  ( -1.999999999999999112, 19.40000000000000213, 26.53589838486224650 ) ) ;
#46833=CARTESIAN_POINT ( 'NONE',  ( 0.6522905807966048464, 20.75364847883808395, 33.69936292076899065 ) ) ;
#46842=ORIENTED_EDGE ( 'NONE', *, *, #22509, .F. ) ;
#46888=CARTESIAN_POINT ( 'NONE',  ( 1.878215178124997609, 19.42812499938548143, 33.25316411605952993 ) ) ;
#46890=CARTESIAN_POINT ( 'NONE',  ( 3.999999999999998668, 13.81249999999999822, 32.30940107675850470 ) ) ;
#46927=CARTESIAN_POINT ( 'NONE',  ( -3.756430356249999214, 20.14062499938548356, 27.83122392262697531 ) ) ;
#46968=CARTESIAN_POINT ( 'NONE',  ( -2.443018120338280585, 25.33977806483805040, 26.82191794298074328 ) ) ;
#46984=CARTESIAN_POINT ( 'NONE',  ( -1.878215178125001827, 18.34062499938548285, 33.25316411605952283 ) ) ;
#47014=CARTESIAN_POINT ( 'NONE',  ( 2.655984681222220721E-16, 13.31562499938548783, 25.66244784525396483 ) ) ;
#47036=CARTESIAN_POINT ( 'NONE',  ( 4.648177544792955741E-15, 14.58124999877096606, 33.99999999999999289 ) ) ;
#47065=ORIENTED_EDGE ( 'NONE', *, *, #28761, .F. ) ;
#47074=CARTESIAN_POINT ( 'NONE',  ( -3.756430356250000102, 16.46562499938548285, 30.00000000000000000 ) ) ;
#47099=CARTESIAN_POINT ( 'NONE',  ( -1.999999999999999112, 14.84374999877096712, 26.53589838486224650 ) ) ;
#47132=CARTESIAN_POINT ( 'NONE',  ( 1.878215178125000495, 16.42812499938548143, 26.74683588394047007 ) ) ;
#47167=CARTESIAN_POINT ( 'NONE',  ( -4.000000000000000888, 19.06249999999999645, 32.30940107675850470 ) ) ;
#47184=CARTESIAN_POINT ( 'NONE',  ( 1.999999999999997335, 19.56874999877096499, 33.46410161513775705 ) ) ;
#47200=ORIENTED_EDGE ( 'NONE', *, *, #14213, .T. ) ;
#47203=CARTESIAN_POINT ( 'NONE',  ( 3.999999999999998668, 15.55624999877096748, 32.30940107675850470 ) ) ;
#47246=CARTESIAN_POINT ( 'NONE',  ( -3.756430356250000102, 19.27812499938548640, 30.00000000000000000 ) ) ;
#47248=CARTESIAN_POINT ( 'NONE',  ( -3.999999999999999556, 12.68750000000000000, 27.69059892324149175 ) ) ;
#47286=CARTESIAN_POINT ( 'NONE',  ( 2.655984681222220721E-16, 19.16562499938548214, 25.66244784525396483 ) ) ;
#47310=VERTEX_POINT ( 'NONE', #29388 ) ;
#47324=CARTESIAN_POINT ( 'NONE',  ( -3.011742865011199921, 25.23389687710447760, 32.64526797158287508 ) ) ;
#47340=CARTESIAN_POINT ( 'NONE',  ( 3.756430356250000102, 18.49062499938548143, 30.00000000000000000 ) ) ;
#47373=CARTESIAN_POINT ( 'NONE',  ( 1.878215178124997609, 13.12812499938548427, 33.25316411605952993 ) ) ;
#47385=ORIENTED_EDGE ( 'NONE', *, *, #1622, .F. ) ;
#47391=EDGE_CURVE ( 'NONE', #13783, #43576, #5764, .T. ) ;
#47418=CARTESIAN_POINT ( 'NONE',  ( 4.898587196589412829E-16, 27.50000000000000000, 34.00000000000000000 ) ) ;
#47433=CARTESIAN_POINT ( 'NONE',  ( 2.655984681222220721E-16, 18.60312499938548214, 25.66244784525396483 ) ) ;
#47435=ORIENTED_EDGE ( 'NONE', *, *, #1622, .T. ) ;
#47443=CARTESIAN_POINT ( 'NONE',  ( 3.756430356249998770, 17.10312499938548214, 32.16877607737302469 ) ) ;
#47456=CARTESIAN_POINT ( 'NONE',  ( -1.999999999999999112, 13.94374999877096677, 26.53589838486224650 ) ) ;
#47460=ORIENTED_EDGE ( 'NONE', *, *, #5433, .F. ) ;
#47491=CARTESIAN_POINT ( 'NONE',  ( -7.967954043666661671E-16, 17.59062499938548285, 34.33755215474603517 ) ) ;
#47507=ORIENTED_EDGE ( 'NONE', *, *, #6118, .T. ) ;
#47607=CARTESIAN_POINT ( 'NONE',  ( -7.967954043666661671E-16, 20.29062499938548214, 34.33755215474603517 ) ) ;
#47609=CARTESIAN_POINT ( 'NONE',  ( 2.000000000000000444, 13.92500000000000071, 26.53589838486224650 ) ) ;
#47621=ORIENTED_EDGE ( 'NONE', *, *, #13863, .T. ) ;
#47647=CARTESIAN_POINT ( 'NONE',  ( -3.756430356250001434, 18.86562499938548498, 32.16877607737301048 ) ) ;
#47686=CARTESIAN_POINT ( 'NONE',  ( 1.878215178125000495, 14.17812499938548321, 26.74683588394047007 ) ) ;
#47699=CARTESIAN_POINT ( 'NONE',  ( 3.756430356249998770, 19.80312499938548143, 32.16877607737301759 ) ) ;
#47731=CARTESIAN_POINT ( 'NONE',  ( -4.000000000000000888, 20.35624999877096641, 32.30940107675850470 ) ) ;
#47787=( BOUNDED_CURVE ( )  B_SPLINE_CURVE ( 2, ( #71931, #48666, #54570, #43123, #9867, #4700, #54939, #4344, #38301 ),
 .UNSPECIFIED., .F., .F. ) 
 B_SPLINE_CURVE_WITH_KNOTS ( ( 3, 2, 2, 2, 3 ),
 ( 0.4861111111111111049, 0.4907407407407407551, 0.5000000000000000000, 0.5092592592592593004, 0.5138888888888889506 ),
 .UNSPECIFIED. ) 
 CURVE ( )  GEOMETRIC_REPRESENTATION_ITEM ( )  RATIONAL_B_SPLINE_CURVE ( ( 0.9330127018922194093, 0.9330127018922194093, 1.000000000000000000, 0.8660254037844387076, 1.000000000000000000, 0.8660254037844387076, 1.000000000000000000, 0.9330127018922185211, 0.9330127018922192983 ) ) 
 REPRESENTATION_ITEM ( '' )  );
#47793=CARTESIAN_POINT ( 'NONE',  ( -1.878215178125001827, 12.94062499938548427, 33.25316411605952283 ) ) ;
#47801=CARTESIAN_POINT ( 'NONE',  ( -3.756430356250000102, 17.81562499938548427, 30.00000000000000000 ) ) ;
#47810=CARTESIAN_POINT ( 'NONE',  ( -3.756430356249999214, 15.07812499938548356, 27.83122392262697531 ) ) ;
#47817=CARTESIAN_POINT ( 'NONE',  ( -2.000000000000001776, 13.70000000000000107, 33.46410161513775705 ) ) ;
#47826=CARTESIAN_POINT ( 'NONE',  ( 1.999999999999997335, 13.26874999877096606, 33.46410161513775705 ) ) ;
#47861=CARTESIAN_POINT ( 'NONE',  ( -1.878215178124999163, 19.65312499938548285, 26.74683588394047007 ) ) ;
#47938=CARTESIAN_POINT ( 'NONE',  ( -1.626862140677534273E-15, 19.53124999877096357, 34.00000000000000000 ) ) ;
#47946=AXIS2_PLACEMENT_3D ( 'NONE', #50954, #719, #38789 ) ;
#47957=DIRECTION ( 'NONE',  ( 0.000000000000000000, 0.000000000000000000, -1.000000000000000000 ) ) ;
#47963=CARTESIAN_POINT ( 'NONE',  ( 1.071796769724489673, 13.49240381056766758, 26.00000000000000000 ) ) ;
#47982=CARTESIAN_POINT ( 'NONE',  ( 3.756430356250000102, 13.54062499938548392, 30.00000000000000000 ) ) ;
#47984=CARTESIAN_POINT ( 'NONE',  ( -2.000000000000001776, 15.94999999999999929, 33.46410161513775705 ) ) ;
#47989=CARTESIAN_POINT ( 'NONE',  ( 5.810221930991193690E-16, 18.01249999999999218, 26.00000000000000000 ) ) ;
#48031=ADVANCED_FACE ( 'NONE', ( #56646 ), #21940, .T. ) ;
#48034=ORIENTED_EDGE ( 'NONE', *, *, #54762, .T. ) ;
#48053=LINE ( 'NONE', #41058, #10878 ) ;
#48062=CARTESIAN_POINT ( 'NONE',  ( -3.471230998791755784, 25.13294848862673803, 27.99513312867361492 ) ) ;
#48075=CARTESIAN_POINT ( 'NONE',  ( 3.756430356250000546, 19.87812499938548427, 27.83122392262697886 ) ) ;
#48108=CARTESIAN_POINT ( 'NONE',  ( -3.756430356250000102, 16.12812499938548427, 30.00000000000000000 ) ) ;
#48132=CARTESIAN_POINT ( 'NONE',  ( 2.000000000000000444, 16.11874999877096570, 26.53589838486224650 ) ) ;
#48151=EDGE_LOOP ( 'NONE', ( #58386, #11280, #25743, #46298 ) ) ;
#48160=CARTESIAN_POINT ( 'NONE',  ( -1.878215178124999163, 13.24062499938548321, 26.74683588394047007 ) ) ;
#48167=CARTESIAN_POINT ( 'NONE',  ( 1.878215178124997609, 20.21562499938548285, 33.25316411605952993 ) ) ;
#48177=CARTESIAN_POINT ( 'NONE',  ( -7.967954043666661671E-16, 16.12812499938548427, 34.33755215474603517 ) ) ;
#48185=CARTESIAN_POINT ( 'NONE',  ( -1.999999999999999112, 14.90000000000000036, 26.53589838486224650 ) ) ;
#48193=CARTESIAN_POINT ( 'NONE',  ( -4.000000000000000888, 14.95624999877096606, 32.30940107675850470 ) ) ;
#48200=EDGE_CURVE ( 'NONE', #9005, #58713, #58581, .T. ) ;
#48227=CARTESIAN_POINT ( 'NONE',  ( -1.878215178125001827, 20.70312499938548001, 33.25316411605952283 ) ) ;
#48232=EDGE_LOOP ( 'NONE', ( #27292, #6551, #35022, #66552, #68975, #46842, #60912, #10780, #66987, #26083, #41958, #44311, #24294, #64352, #35676, #31092, #34966, #68431, #15453, #20423, #72093, #68054, #16345, #70605, #37739, #20056, #4501, #55252, #4299, #46778, #32926, #1506, #57805, #24295, #18271, #202, #15434, #11748, #29463, #43118 ) ) ;
#48242=EDGE_CURVE ( 'NONE', #27263, #65514, #12859, .T. ) ;
#48261=CARTESIAN_POINT ( 'NONE',  ( -1.071796769724490339, 14.82634618820330097, 26.00000000000000000 ) ) ;
#48264=CARTESIAN_POINT ( 'NONE',  ( -1.626862140677534273E-15, 19.58750000000000213, 34.00000000000000000 ) ) ;
#48302=CARTESIAN_POINT ( 'NONE',  ( 4.648177544792955741E-15, 13.73749999999999716, 33.99999999999999289 ) ) ;
#48341=DIRECTION ( 'NONE',  ( 0.000000000000000000, 0.000000000000000000, 1.000000000000000000 ) ) ;
#48349=CARTESIAN_POINT ( 'NONE',  ( -3.756430356250000102, 12.86562499938548321, 30.00000000000000000 ) ) ;
#48351=CARTESIAN_POINT ( 'NONE',  ( -3.999999999999999556, 15.83750000000000036, 27.69059892324149175 ) ) ;
#48385=CARTESIAN_POINT ( 'NONE',  ( -1.999999999999999112, 17.60000000000000142, 26.53589838486224650 ) ) ;
#48434=CARTESIAN_POINT ( 'NONE',  ( -3.756430356249999214, 14.29062499938548214, 27.83122392262697531 ) ) ;
#48446=CARTESIAN_POINT ( 'NONE',  ( -3.756430356250000102, 19.61562499938548143, 30.00000000000000000 ) ) ;
#48476=CARTESIAN_POINT ( 'NONE',  ( 3.756430356250000102, 15.00312499938548427, 30.00000000000000000 ) ) ;
#48501=CYLINDRICAL_SURFACE ( 'NONE', #6504, 4.000000000000000000 ) ;
#48536=CARTESIAN_POINT ( 'NONE',  ( -7.967954043666661671E-16, 18.82812499938548356, 34.33755215474603517 ) ) ;
#48545=CARTESIAN_POINT ( 'NONE',  ( -1.878215178125001827, 15.64062499938548356, 33.25316411605952283 ) ) ;
#48560=CARTESIAN_POINT ( 'NONE',  ( 4.000000000000000000, 16.49374999877096570, 30.00000000000000000 ) ) ;
#48594=CARTESIAN_POINT ( 'NONE',  ( 1.878215178125000495, 20.47812499938548569, 26.74683588394047007 ) ) ;
#48629=CARTESIAN_POINT ( 'NONE',  ( -4.000000000000000888, 18.10624999877096641, 32.30940107675850470 ) ) ;
#48666=CARTESIAN_POINT ( 'NONE',  ( 1.071796769724488785, 16.85134618820330132, 34.00000000000000000 ) ) ;
#48676=CARTESIAN_POINT ( 'NONE',  ( -1.878215178124999163, 12.79062499938548392, 26.74683588394047007 ) ) ;
#48686=CARTESIAN_POINT ( 'NONE',  ( -3.756430356249999214, 13.39062499938548179, 27.83122392262697176 ) ) ;
#48714=CARTESIAN_POINT ( 'NONE',  ( 3.756430356250000102, 13.09062499938548463, 30.00000000000000000 ) ) ;
#48716=CARTESIAN_POINT ( 'NONE',  ( 2.000000000000000444, 14.82500000000000107, 26.53589838486224650 ) ) ;
#48797=CARTESIAN_POINT ( 'NONE',  ( -3.756430356250000102, 12.97812499938548214, 30.00000000000000000 ) ) ;
#48808=CARTESIAN_POINT ( 'NONE',  ( -1.878215178125001827, 20.14062499938548356, 33.25316411605952283 ) ) ;
#48827=ORIENTED_EDGE ( 'NONE', *, *, #25975, .T. ) ;
#48839=CARTESIAN_POINT ( 'NONE',  ( -3.756430356250000102, 15.22812499938548392, 30.00000000000000000 ) ) ;
#48865=CARTESIAN_POINT ( 'NONE',  ( -2.672702088255949472E-15, 13.45624999877096784, 26.00000000000000000 ) ) ;
#48902=CARTESIAN_POINT ( 'NONE',  ( 3.756430356250000546, 19.42812499938548143, 27.83122392262697886 ) ) ;
#48907=CLOSED_SHELL ( 'NONE', ( #37347, #37175, #55855, #9012, #29568, #40485, #43137, #42580, #19024, #30040, #10333, #4102, #48031, #26087, #56863, #64386, #69287, #69757, #11148, #35563, #12542, #21291, #24565, #55678, #67441, #17317, #62389, #17706, #27243, #60747, #53579, #52407, #11636, #20661, #61932, #9517, #55412, #21155, #62663, #24600, #64171, #34272, #32148, #30551, #7221, #41033, #43795, #9054 ) ) ;
#48912=CARTESIAN_POINT ( 'NONE',  ( 1.878215178125000495, 16.31562499938548427, 26.74683588394047007 ) ) ;
#48930=CARTESIAN_POINT ( 'NONE',  ( -1.999999999999999112, 16.64374999877096784, 26.53589838486224650 ) ) ;
#48962=CARTESIAN_POINT ( 'NONE',  ( -1.878215178124999163, 20.55312499938548143, 26.74683588394047007 ) ) ;
#48963=CARTESIAN_POINT ( 'NONE',  ( 5.810221930991193690E-16, 14.41249999999999787, 26.00000000000000000 ) ) ;
#49013=AXIS2_PLACEMENT_3D ( 'NONE', #7203, #33829, #6844 ) ;
#49047=CARTESIAN_POINT ( 'NONE',  ( -7.967954043666661671E-16, 12.97812499938548392, 34.33755215474603517 ) ) ;
#49056=CARTESIAN_POINT ( 'NONE',  ( 3.756430356250000102, 12.75312499938548427, 30.00000000000000000 ) ) ;
#49067=ORIENTED_EDGE ( 'NONE', *, *, #59834, .F. ) ;
#49085=CARTESIAN_POINT ( 'NONE',  ( 2.655984681222220721E-16, 13.65312499938548463, 25.66244784525396483 ) ) ;
#49087=CARTESIAN_POINT ( 'NONE',  ( -2.000000000000001776, 14.15000000000000036, 33.46410161513775705 ) ) ;
#49161=CARTESIAN_POINT ( 'NONE',  ( -3.999999999999999112, 15.83750000000000036, 27.69059892324149530 ) ) ;
#49170=CARTESIAN_POINT ( 'NONE',  ( -1.878215178125001827, 13.50312499938548427, 33.25316411605952283 ) ) ;
#49210=CARTESIAN_POINT ( 'NONE',  ( -3.756430356250001434, 15.71562499938548108, 32.16877607737301048 ) ) ;
#49222=VERTEX_POINT ( 'NONE', #57180 ) ;
#49254=CARTESIAN_POINT ( 'NONE',  ( -1.999999999999999112, 19.79374999877096286, 26.53589838486224650 ) ) ;
#49261=ORIENTED_EDGE ( 'NONE', *, *, #19955, .T. ) ;
#49265=CARTESIAN_POINT ( 'NONE',  ( 3.756430356249998770, 14.85312499938548214, 32.16877607737301759 ) ) ;
#49271=CARTESIAN_POINT ( 'NONE',  ( 3.756430356250000546, 18.97812499938548214, 27.83122392262697886 ) ) ;
#49280=CARTESIAN_POINT ( 'NONE',  ( 3.756430356250000102, 17.59062499938548285, 30.00000000000000000 ) ) ;
#49288=CARTESIAN_POINT ( 'NONE',  ( 1.999999999999997335, 15.12500000000000000, 33.46410161513775705 ) ) ;
#49295=CARTESIAN_POINT ( 'NONE',  ( 3.999999999999998668, 16.45624999877096784, 32.30940107675850470 ) ) ;
#49299=VERTEX_POINT ( 'NONE', #69401 ) ;
#49328=CARTESIAN_POINT ( 'NONE',  ( -3.756430356250000102, 19.27812499938548640, 30.00000000000000000 ) ) ;
#49337=CARTESIAN_POINT ( 'NONE',  ( 0.000000000000000000, 27.50000000000000000, 30.00000000000000000 ) ) ;
#49361=CARTESIAN_POINT ( 'NONE',  ( -1.626862140677534273E-15, 15.03124999877096535, 34.00000000000000000 ) ) ;
#49408=CARTESIAN_POINT ( 'NONE',  ( -1.878215178125001827, 13.84062499938548285, 33.25316411605952283 ) ) ;
#49418=CARTESIAN_POINT ( 'NONE',  ( -4.000000000000000888, 16.81250000000000000, 32.30940107675850470 ) ) ;
#49424=EDGE_LOOP ( 'NONE', ( #3665, #56779, #38577, #30554 ) ) ;
#49443=CARTESIAN_POINT ( 'NONE',  ( 3.756430356250000546, 14.47812499938548747, 27.83122392262697886 ) ) ;
#49445=CARTESIAN_POINT ( 'NONE',  ( -2.000000000000001776, 17.75000000000000355, 33.46410161513775705 ) ) ;
#49494=EDGE_CURVE ( 'NONE', #16672, #27542, #8057, .T. ) ;
#49531=CARTESIAN_POINT ( 'NONE',  ( -7.967954043666661671E-16, 15.34062499938548463, 34.33755215474603517 ) ) ;
#49537=EDGE_CURVE ( 'NONE', #72457, #67390, #54585, .T. ) ;
#49574=CARTESIAN_POINT ( 'NONE',  ( -3.756430356249999214, 16.09062499938548285, 27.83122392262697531 ) ) ;
#49591=EDGE_CURVE ( 'NONE', #21163, #70620, #2944, .T. ) ;
#49616=CARTESIAN_POINT ( 'NONE',  ( -1.071796769724492115, 19.96115380933863293, 34.00000000000000000 ) ) ;
#49628=CARTESIAN_POINT ( 'NONE',  ( 3.756430356250000546, 15.82812499938548356, 27.83122392262697886 ) ) ;
#49631=VERTEX_POINT ( 'NONE', #20954 ) ;
#49634=CARTESIAN_POINT ( 'NONE',  ( 1.878215178125000495, 19.91562499938548569, 26.74683588394047007 ) ) ;
#49644=CARTESIAN_POINT ( 'NONE',  ( -3.756430356250000102, 17.81562499938548427, 30.00000000000000000 ) ) ;
#49660=CARTESIAN_POINT ( 'NONE',  ( -3.999999999999999556, 16.68124999877096570, 27.69059892324149175 ) ) ;
#49663=CARTESIAN_POINT ( 'NONE',  ( 1.071796769724490561, 12.85759618943233917, 34.00000000000000000 ) ) ;
#49690=AXIS2_PLACEMENT_3D ( 'NONE', #70501, #8436, #19507 ) ;
#49694=CARTESIAN_POINT ( 'NONE',  ( -1.071796769724502107, 20.67634618820330417, 26.00000000000000711 ) ) ;
#49708=ORIENTED_EDGE ( 'NONE', *, *, #52890, .T. ) ;
#49712=CARTESIAN_POINT ( 'NONE',  ( 1.999999999999997335, 19.17500000000000071, 33.46410161513775705 ) ) ;
#49722=MECHANICAL_DESIGN_GEOMETRIC_PRESENTATION_REPRESENTATION('',(#37895),#62674);
#49776=CARTESIAN_POINT ( 'NONE',  ( -3.756430356249999214, 13.27812499938548463, 27.83122392262697531 ) ) ;
#49781=CARTESIAN_POINT ( 'NONE',  ( -2.000000000000001776, 18.59374999877096357, 33.46410161513775705 ) ) ;
#49784=CARTESIAN_POINT ( 'NONE',  ( -7.967954043666661671E-16, 13.99062499938548498, 34.33755215474603517 ) ) ;
#49786=CARTESIAN_POINT ( 'NONE',  ( -2.000000000000001776, 16.85000000000000142, 33.46410161513775705 ) ) ;
#49811=CARTESIAN_POINT ( 'NONE',  ( 3.756430356249998770, 13.95312499938548179, 32.16877607737302469 ) ) ;
#49813=CARTESIAN_POINT ( 'NONE',  ( 1.999999999999997335, 16.47500000000000142, 33.46410161513775705 ) ) ;
#49855=VERTEX_POINT ( 'NONE', #26885 ) ;
#49873=FACE_OUTER_BOUND ( 'NONE', #54833, .T. ) ;
#49892=CARTESIAN_POINT ( 'NONE',  ( 3.756430356250000546, 16.84062499938548285, 27.83122392262697886 ) ) ;
#49935=CARTESIAN_POINT ( 'NONE',  ( -3.756430356250001434, 18.41562499938548214, 32.16877607737301048 ) ) ;
#49947=ORIENTED_EDGE ( 'NONE', *, *, #21313, .T. ) ;
#49986=EDGE_CURVE ( 'NONE', #49299, #70620, #9153, .T. ) ;
#49992=CARTESIAN_POINT ( 'NONE',  ( -1.878215178125001827, 13.84062499938548285, 33.25316411605952283 ) ) ;
#50008=CARTESIAN_POINT ( 'NONE',  ( -1.878215178124999163, 18.64062499938548356, 26.74683588394047007 ) ) ;
#50024=CARTESIAN_POINT ( 'NONE',  ( 3.999999999999998668, 18.70624999877096784, 32.30940107675850470 ) ) ;
#50109=CARTESIAN_POINT ( 'NONE',  ( -4.000000000000000000, 19.02499999999999858, 30.00000000000000000 ) ) ;
#50135=VECTOR ( 'NONE', #64503, 1000.000000000000000 ) ;
#50138=CARTESIAN_POINT ( 'NONE',  ( 3.756430356250000102, 14.89062499938548356, 30.00000000000000000 ) ) ;
#50148=CARTESIAN_POINT ( 'NONE',  ( -1.878215178125001827, 13.95312499938548356, 33.25316411605952283 ) ) ;
#50175=CARTESIAN_POINT ( 'NONE',  ( 2.655984681222220721E-16, 15.90312499938548108, 25.66244784525396483 ) ) ;
#50178=CARTESIAN_POINT ( 'NONE',  ( -4.000000000000000000, 17.22500000000000142, 30.00000000000000000 ) ) ;
#50223=ORIENTED_EDGE ( 'NONE', *, *, #5878, .F. ) ;
#50224=B_SPLINE_CURVE_WITH_KNOTS ( 'NONE', 3,
 ( #29513, #19868, #12876, #2527, #30961, #7701, #63842, #58661, #52770, #8425, #13233, #36142, #57934, #70120, #52048, #29870, #52408, #63488, #7341, #35409, #13966, #36504, #2172, #24683, #64578, #1452, #13596, #35771, #53497, #1816, #8069, #23958 ),
 .UNSPECIFIED., .F., .F.,
 ( 4, 2, 2, 2, 2, 2, 2, 2, 2, 2, 2, 2, 2, 2, 2, 4 ),
 ( 0.000000000000000000, 0.0007851728441139026876, 0.001570345688227805375, 0.002355518532341708063, 0.003140691376455610750, 0.003925864220569513438, 0.004711037064683416126, 0.005496209908797318813, 0.006281382752911221501, 0.007066555597025125056, 0.007851728441139026876, 0.009422074129366811435, 0.01020724697348069851, 0.01099241981759458385, 0.01177759266170846919, 0.01256276550582235453 ),
 .UNSPECIFIED. ) ;
#50260=FACE_OUTER_BOUND ( 'NONE', #51607, .T. ) ;
#50263=CARTESIAN_POINT ( 'NONE',  ( 3.756430356250000102, 16.35312499938548569, 30.00000000000000000 ) ) ;
#50292=APPLICATION_CONTEXT ( 'automotive_design' ) ;
#50309=CARTESIAN_POINT ( 'NONE',  ( 3.756430356250000546, 16.39062499938548356, 27.83122392262697886 ) ) ;
#50333=CARTESIAN_POINT ( 'NONE',  ( 1.999999999999997335, 15.06874999877096677, 33.46410161513775705 ) ) ;
#50361=CARTESIAN_POINT ( 'NONE',  ( 2.655984681222220721E-16, 14.55312499938548321, 25.66244784525396483 ) ) ;
#50364=ORIENTED_EDGE ( 'NONE', *, *, #48242, .T. ) ;
#50377=CARTESIAN_POINT ( 'NONE',  ( 1.878215178125000495, 19.46562499938548640, 26.74683588394047007 ) ) ;
#50391=CARTESIAN_POINT ( 'NONE',  ( -4.000000000000000000, 18.96874999877096357, 30.00000000000000000 ) ) ;
#50417=CARTESIAN_POINT ( 'NONE',  ( 3.756430356250000102, 12.64062499938548356, 30.00000000000000000 ) ) ;
#50473=( LENGTH_UNIT ( ) NAMED_UNIT ( * ) SI_UNIT ( .MILLI., .METRE. ) );
#50502=CARTESIAN_POINT ( 'NONE',  ( 1.071796769724491893, 13.75759618943233420, 34.00000000000000000 ) ) ;
#50509=CARTESIAN_POINT ( 'NONE',  ( 3.756430356250000102, 15.00312499938548427, 30.00000000000000000 ) ) ;
#50510=CARTESIAN_POINT ( 'NONE',  ( -1.071796769724486120, 15.46115380933863293, 34.00000000000000000 ) ) ;
#50521=VERTEX_POINT ( 'NONE', #8976 ) ;
#50528=CARTESIAN_POINT ( 'NONE',  ( 1.071796769724488785, 19.60759618943233562, 34.00000000000000000 ) ) ;
#50539=CARTESIAN_POINT ( 'NONE',  ( -8.484601909799255319E-16, 18.23750000000000071, 34.61880215351700940 ) ) ;
#50572=EDGE_LOOP ( 'NONE', ( #71713, #66317, #64277, #20882 ) ) ;
#50573=VERTEX_POINT ( 'NONE', #31133 ) ;
#50598=CARTESIAN_POINT ( 'NONE',  ( 4.000000000000000000, 12.50000000000000000, 30.00000000000000000 ) ) ;
#50619=CARTESIAN_POINT ( 'NONE',  ( -3.756430356249999214, 16.54062499938548569, 27.83122392262697531 ) ) ;
#50649=ORIENTED_EDGE ( 'NONE', *, *, #22559, .F. ) ;
#50662=CARTESIAN_POINT ( 'NONE',  ( -3.756430356249999214, 16.54062499938548569, 27.83122392262697531 ) ) ;
#50685=CARTESIAN_POINT ( 'NONE',  ( -1.999999999999999112, 19.84999999999999787, 26.53589838486224650 ) ) ;
#50698=ORIENTED_EDGE ( 'NONE', *, *, #64830, .T. ) ;
#50714=LINE ( 'NONE', #68070, #35958 ) ;
#50717=CARTESIAN_POINT ( 'NONE',  ( -3.756430356249999214, 13.72812499938548392, 27.83122392262697176 ) ) ;
#50733=CARTESIAN_POINT ( 'NONE',  ( 3.756430356249998770, 18.90312499938548640, 32.16877607737302469 ) ) ;
#50737=EDGE_LOOP ( 'NONE', ( #34265, #413, #47200, #70421 ) ) ;
#50747=CARTESIAN_POINT ( 'NONE',  ( 4.000000000000000000, 17.84374999877096712, 30.00000000000000000 ) ) ;
#50750=CARTESIAN_POINT ( 'NONE',  ( 4.000000000000000000, 12.95000000000000107, 30.00000000000000000 ) ) ;
#50808=ORIENTED_EDGE ( 'NONE', *, *, #6209, .T. ) ;
#50856=CIRCLE ( 'NONE', #28424, 4.000000000000003553 ) ;
#50861=CARTESIAN_POINT ( 'NONE',  ( 4.000000000000000000, 13.88750000000000107, 27.69059892324149885 ) ) ;
#50866=CARTESIAN_POINT ( 'NONE',  ( -3.756430356249999214, 14.74062499938548676, 27.83122392262697176 ) ) ;
#50872=DIRECTION ( 'NONE',  ( -0.000000000000000000, -1.000000000000000000, -0.000000000000000000 ) ) ;
#50896=CARTESIAN_POINT ( 'NONE',  ( -2.000000000000001776, 17.30000000000000071, 33.46410161513775705 ) ) ;
#50916=EDGE_CURVE ( 'NONE', #27263, #55447, #66586, .T. ) ;
#50954=CARTESIAN_POINT ( 'NONE',  ( 0.000000000000000000, 27.50000000000000000, 30.00000000000000000 ) ) ;
#50977=CARTESIAN_POINT ( 'NONE',  ( -1.878215178125001827, 16.65312499938548285, 33.25316411605952283 ) ) ;
#50986=CARTESIAN_POINT ( 'NONE',  ( 0.6522905807966048464, 20.75364847883808395, 33.69936292076899065 ) ) ;
#51020=CARTESIAN_POINT ( 'NONE',  ( 3.756430356249998770, 16.31562499938548427, 32.16877607737302469 ) ) ;
#51024=( BOUNDED_CURVE ( )  B_SPLINE_CURVE ( 2, ( #4664, #67454, #39009 ),
 .UNSPECIFIED., .F., .F. ) 
 B_SPLINE_CURVE_WITH_KNOTS ( ( 3, 3 ),
 ( 0.9861111111111111605, 0.9876227203420996359 ),
 .UNSPECIFIED. ) 
 CURVE ( )  GEOMETRIC_REPRESENTATION_ITEM ( )  RATIONAL_B_SPLINE_CURVE ( ( 0.9330127018922194093, 0.9330127018922197424, 0.9401540307732418889 ) ) 
 REPRESENTATION_ITEM ( '' )  );
#51029=CARTESIAN_POINT ( 'NONE',  ( 2.393811435568372112E-14, 17.28124999877096712, 34.00000000000000000 ) ) ;
#51052=AXIS2_PLACEMENT_3D ( 'NONE', #43972, #72398, #15874 ) ;
#51076=CARTESIAN_POINT ( 'NONE',  ( 3.756430356250000546, 17.62812499938548427, 27.83122392262697886 ) ) ;
#51109=CARTESIAN_POINT ( 'NONE',  ( 1.999999999999997335, 17.76874999877096428, 33.46410161513775705 ) ) ;
#51112=CARTESIAN_POINT ( 'NONE',  ( 1.626862140677534470E-15, 12.83750000000000213, 34.00000000000000000 ) ) ;
#51119=FACE_OUTER_BOUND ( 'NONE', #20389, .T. ) ;
#51135=CARTESIAN_POINT ( 'NONE',  ( 0.000000000000000000, 27.50000000000000000, 30.00000000000000000 ) ) ;
#51140=DIRECTION ( 'NONE',  ( -0.000000000000000000, -1.000000000000000000, -0.000000000000000000 ) ) ;
#51192=( NAMED_UNIT ( * ) SI_UNIT ( $, .STERADIAN. ) SOLID_ANGLE_UNIT ( ) );
#51227=CARTESIAN_POINT ( 'NONE',  ( 2.655984681222220721E-16, 15.11562499938548321, 25.66244784525396483 ) ) ;
#51228=CARTESIAN_POINT ( 'NONE',  ( -1.071796769724489229, 14.11115380933862973, 34.00000000000000000 ) ) ;
#51259=CARTESIAN_POINT ( 'NONE',  ( -4.000000000000000000, 19.47499999999999787, 30.00000000000000000 ) ) ;
#51293=VERTEX_POINT ( 'NONE', #51029 ) ;
#51296=CARTESIAN_POINT ( 'NONE',  ( 2.000000000000000444, 18.36874999877096570, 26.53589838486224650 ) ) ;
#51305=CARTESIAN_POINT ( 'NONE',  ( -1.626862140677534273E-15, 17.78749999999999787, 34.00000000000000000 ) ) ;
#51316=AXIS2_PLACEMENT_3D ( 'NONE', #31732, #19900, #41713 ) ;
#51324=( LENGTH_UNIT ( ) NAMED_UNIT ( * ) SI_UNIT ( .MILLI., .METRE. ) );
#51341=CARTESIAN_POINT ( 'NONE',  ( -1.878215178125001827, 18.00312499938548427, 33.25316411605952283 ) ) ;
#51381=CARTESIAN_POINT ( 'NONE',  ( -7.967954043666661671E-16, 17.14062499938548356, 34.33755215474603517 ) ) ;
#51425=DIRECTION ( 'NONE',  ( -0.000000000000000000, -1.000000000000000000, -0.000000000000000000 ) ) ;
#51438=CARTESIAN_POINT ( 'NONE',  ( -1.878215178124999163, 16.39062499938548356, 26.74683588394047007 ) ) ;
#51469=CARTESIAN_POINT ( 'NONE',  ( 1.999999999999997335, 19.11874999877096570, 33.46410161513775705 ) ) ;
#51499=FACE_OUTER_BOUND ( 'NONE', #65132, .T. ) ;
#51512=AXIS2_PLACEMENT_3D ( 'NONE', #6598, #29128, #51661 ) ;
#51521=ORIENTED_EDGE ( 'NONE', *, *, #20103, .F. ) ;
#51533=CARTESIAN_POINT ( 'NONE',  ( -3.756430356249999214, 15.97812499938548392, 27.83122392262697531 ) ) ;
#51535=ORIENTED_EDGE ( 'NONE', *, *, #33859, .T. ) ;
#51581=AXIS2_PLACEMENT_3D ( 'NONE', #20488, #25689, #64840 ) ;
#51595=CARTESIAN_POINT ( 'NONE',  ( -1.878215178124999163, 17.40312499938548285, 26.74683588394047007 ) ) ;
#51601=DIRECTION ( 'NONE',  ( 0.000000000000000000, 1.000000000000000000, 0.000000000000000000 ) ) ;
#51607=EDGE_LOOP ( 'NONE', ( #62445, #63188, #67086, #63218 ) ) ;
#51626=CARTESIAN_POINT ( 'NONE',  ( 1.999999999999997335, 20.07499999999999929, 33.46410161513775705 ) ) ;
#51649=CARTESIAN_POINT ( 'NONE',  ( 4.648177544792955741E-15, 14.18750000000000000, 33.99999999999999289 ) ) ;
#51661=DIRECTION ( 'NONE',  ( 0.000000000000000000, 0.000000000000000000, -1.000000000000000000 ) ) ;
#51668=DIRECTION ( 'NONE',  ( 0.000000000000000000, 0.000000000000000000, -1.000000000000000000 ) ) ;
#51705=CARTESIAN_POINT ( 'NONE',  ( -3.756430356250000102, 17.92812499938548498, 30.00000000000000000 ) ) ;
#51707=CARTESIAN_POINT ( 'NONE',  ( -3.999999999999999556, 13.13750000000000107, 27.69059892324149175 ) ) ;
#51742=ORIENTED_EDGE ( 'NONE', *, *, #55968, .F. ) ;
#51798=CARTESIAN_POINT ( 'NONE',  ( 1.878215178124997609, 17.06562499938548072, 33.25316411605952993 ) ) ;
#51815=VERTEX_POINT ( 'NONE', #18094 ) ;
#51820=CARTESIAN_POINT ( 'NONE',  ( -1.071796769724502107, 17.07634618820330275, 26.00000000000000711 ) ) ;
#51827=CARTESIAN_POINT ( 'NONE',  ( -7.967954043666661671E-16, 13.54062499938548214, 34.33755215474603517 ) ) ;
#51852=CARTESIAN_POINT ( 'NONE',  ( -4.000000000000000888, 13.21250000000000036, 32.30940107675850470 ) ) ;
#51872=( BOUNDED_CURVE ( )  B_SPLINE_CURVE ( 2, ( #59191, #14869, #59560, #31130, #36312, #59931, #48132, #31870, #70656 ),
 .UNSPECIFIED., .F., .F. ) 
 B_SPLINE_CURVE_WITH_KNOTS ( ( 3, 2, 2, 2, 3 ),
 ( 0.3750000000000000000, 0.3796296296296296502, 0.3888888888888888951, 0.3981481481481481399, 0.4027777777777777901 ),
 .UNSPECIFIED. ) 
 CURVE ( )  GEOMETRIC_REPRESENTATION_ITEM ( )  RATIONAL_B_SPLINE_CURVE ( ( 0.9330127018922194093, 0.9330127018922194093, 1.000000000000000000, 0.8660254037844387076, 1.000000000000000000, 0.8660254037844387076, 1.000000000000000000, 0.9330127018922189652, 0.9330127018922194093 ) ) 
 REPRESENTATION_ITEM ( '' )  );
#51886=CARTESIAN_POINT ( 'NONE',  ( 0.3499505129295816808, 20.49406157211743462, 34.00000000000000000 ) ) ;
#51891=CARTESIAN_POINT ( 'NONE',  ( 1.878215178124997609, 16.16562499938548569, 33.25316411605952993 ) ) ;
#51952=CARTESIAN_POINT ( 'NONE',  ( -1.878215178125001827, 18.00312499938548427, 33.25316411605952283 ) ) ;
#51961=EDGE_CURVE ( 'NONE', #70824, #53784, #36082, .T. ) ;
#51986=CARTESIAN_POINT ( 'NONE',  ( 2.828200636599751609E-16, 20.26249999999999929, 25.38119784648299415 ) ) ;
#52032=CARTESIAN_POINT ( 'NONE',  ( 2.000000000000000444, 17.97500000000000142, 26.53589838486224650 ) ) ;
#52048=CARTESIAN_POINT ( 'NONE',  ( 3.871071818048498869, 25.03394779433038408, 28.95871227317249463 ) ) ;
#52065=CARTESIAN_POINT ( 'NONE',  ( 3.756430356250000102, 17.25312499938548072, 30.00000000000000000 ) ) ;
#52067=CARTESIAN_POINT ( 'NONE',  ( -0.6941640578732103384, 20.61426548399373004, 33.93677634907117380 ) ) ;
#52104=CARTESIAN_POINT ( 'NONE',  ( 1.878215178125000495, 19.57812499938548356, 26.74683588394047007 ) ) ;
#52118=UNCERTAINTY_MEASURE_WITH_UNIT (LENGTH_MEASURE( 1.000000000000000082E-05 ), #22740, 'distance_accuracy_value', 'NONE');
#52160=CARTESIAN_POINT ( 'NONE',  ( 1.878215178125000495, 17.66562499938548214, 26.74683588394047007 ) ) ;
#52190=CARTESIAN_POINT ( 'NONE',  ( -3.756430356250001434, 13.01562499938548534, 32.16877607737301048 ) ) ;
#52243=ORIENTED_EDGE ( 'NONE', *, *, #35065, .T. ) ;
#52251=CARTESIAN_POINT ( 'NONE',  ( 2.655984681222220721E-16, 17.25312499938548072, 25.66244784525396483 ) ) ;
#52276=CARTESIAN_POINT ( 'NONE',  ( -8.484601909799255319E-16, 14.58124999877096606, 34.61880215351700940 ) ) ;
#52294=FACE_OUTER_BOUND ( 'NONE', #66412, .T. ) ;
#52309=CARTESIAN_POINT ( 'NONE',  ( -3.756430356249999214, 16.09062499938548285, 27.83122392262697176 ) ) ;
#52343=CARTESIAN_POINT ( 'NONE',  ( 3.999999999999998668, 19.21250000000000213, 32.30940107675850470 ) ) ;
#52407=ADVANCED_FACE ( 'NONE', ( #39959 ), #27422, .T. ) ;
#52408=CARTESIAN_POINT ( 'NONE',  ( 3.999890280212508475, 25.00002925860763625, 29.73607354501108446 ) ) ;
#52426=CARTESIAN_POINT ( 'NONE',  ( 1.878215178124997609, 18.97812499938548214, 33.25316411605952993 ) ) ;
#52428=CARTESIAN_POINT ( 'NONE',  ( -1.999999999999999112, 13.55000000000000071, 26.53589838486224650 ) ) ;
#52466=CARTESIAN_POINT ( 'NONE',  ( -3.756430356250000102, 19.27812499938548640, 30.00000000000000000 ) ) ;
#52504=CARTESIAN_POINT ( 'NONE',  ( -3.973417775690189835, 25.00714840155672292, 30.52930962823944938 ) ) ;
#52521=CARTESIAN_POINT ( 'NONE',  ( -3.756430356250000102, 18.26562499938548356, 30.00000000000000000 ) ) ;
#52544=CARTESIAN_POINT ( 'NONE',  ( 4.000000000000000000, 18.78124999877096357, 27.69059892324149885 ) ) ;
#52553=CARTESIAN_POINT ( 'NONE',  ( 2.828200636599751609E-16, 20.20624999877096784, 25.38119784648299415 ) ) ;
#52564=ORIENTED_EDGE ( 'NONE', *, *, #8903, .T. ) ;
#52575=CARTESIAN_POINT ( 'NONE',  ( -1.071796769724490783, 13.26740381056766616, 34.00000000000000711 ) ) ;
#52580=CIRCLE ( 'NONE', #20734, 4.000000000000003553 ) ;
#52594=DIRECTION ( 'NONE',  ( 0.000000000000000000, 0.000000000000000000, 1.000000000000000000 ) ) ;
#52613=CARTESIAN_POINT ( 'NONE',  ( 3.756430356250000546, 16.27812499938548285, 27.83122392262697886 ) ) ;
#52636=CARTESIAN_POINT ( 'NONE',  ( 4.000000000000000000, 14.24374999877096748, 30.00000000000000000 ) ) ;
#52668=CARTESIAN_POINT ( 'NONE',  ( 1.878215178124997609, 17.17812499938548498, 33.25316411605952993 ) ) ;
#52720=CARTESIAN_POINT ( 'NONE',  ( 1.071796769724488785, 19.55134618820330417, 34.00000000000000000 ) ) ;
#52752=CARTESIAN_POINT ( 'NONE',  ( 1.878215178125000495, 12.71562499938548463, 26.74683588394047007 ) ) ;
#52764=DIRECTION ( 'NONE',  ( -0.000000000000000000, -1.000000000000000000, -0.000000000000000000 ) ) ;
#52770=CARTESIAN_POINT ( 'NONE',  ( 2.645498907222010754, 25.30421092789820392, 26.98856407078577391 ) ) ;
#52787=CARTESIAN_POINT ( 'NONE',  ( 1.878215178125000495, 19.57812499938548356, 26.74683588394047007 ) ) ;
#52789=CARTESIAN_POINT ( 'NONE',  ( 3.756430356250000102, 19.84062499938548640, 30.00000000000000000 ) ) ;
#52827=CARTESIAN_POINT ( 'NONE',  ( -3.756430356250001434, 20.21562499938548285, 32.16877607737301048 ) ) ;
#52882=CARTESIAN_POINT ( 'NONE',  ( 3.756430356250000546, 20.32812499938548711, 27.83122392262697886 ) ) ;
#52890=EDGE_CURVE ( 'NONE', #29218, #50573, #58723, .T. ) ;
#52913=CARTESIAN_POINT ( 'NONE',  ( 3.999999999999998668, 20.50624999877096499, 32.30940107675850470 ) ) ;
#52935=LINE ( 'NONE', #35220, #20605 ) ;
#52974=CARTESIAN_POINT ( 'NONE',  ( -3.756430356250000102, 17.36562499938548498, 30.00000000000000000 ) ) ;
#52984=CARTESIAN_POINT ( 'NONE',  ( -3.756430356250001434, 16.95312499938548356, 32.16877607737301048 ) ) ;
#52998=CARTESIAN_POINT ( 'NONE',  ( -2.000000000000001776, 13.19374999877096677, 33.46410161513775705 ) ) ;
#53030=CARTESIAN_POINT ( 'NONE',  ( 3.756430356249998770, 17.21562499938548285, 32.16877607737301759 ) ) ;
#53046=ORIENTED_EDGE ( 'NONE', *, *, #19843, .T. ) ;
#53110=CARTESIAN_POINT ( 'NONE',  ( -3.756430356250000102, 12.86562499938548321, 30.00000000000000000 ) ) ;
#53130=EDGE_CURVE ( 'NONE', #71973, #12632, #70932, .T. ) ;
#53146=CARTESIAN_POINT ( 'NONE',  ( -3.756430356250001434, 20.66562499938548569, 32.16877607737301048 ) ) ;
#53148=CARTESIAN_POINT ( 'NONE',  ( 2.828200636599751609E-16, 13.06250000000000355, 25.38119784648299415 ) ) ;
#53183=CARTESIAN_POINT ( 'NONE',  ( 5.810221930991193690E-16, 17.56250000000000000, 26.00000000000000000 ) ) ;
#53187=CARTESIAN_POINT ( 'NONE',  ( 1.878215178124997609, 19.42812499938548143, 33.25316411605952993 ) ) ;
#53224=CARTESIAN_POINT ( 'NONE',  ( -1.297222828952121931, 25.48705884896387985, 26.20721131224835787 ) ) ;
#53227=CARTESIAN_POINT ( 'NONE',  ( 3.756430356249998770, 14.51562499938548356, 32.16877607737302469 ) ) ;
#53241=CARTESIAN_POINT ( 'NONE',  ( 1.878215178124997609, 19.31562499938548427, 33.25316411605952993 ) ) ;
#53243=ORIENTED_EDGE ( 'NONE', *, *, #53130, .T. ) ;
#53273=CARTESIAN_POINT ( 'NONE',  ( 2.000000000000000444, 20.61874999877096570, 26.53589838486224650 ) ) ;
#53331=CARTESIAN_POINT ( 'NONE',  ( -1.071796769724490339, 13.98259618943233740, 26.00000000000000000 ) ) ;
#53337=CARTESIAN_POINT ( 'NONE',  ( -7.967954043666661671E-16, 17.02812499938548285, 34.33755215474603517 ) ) ;
#53346=CARTESIAN_POINT ( 'NONE',  ( -1.878215178124999163, 15.04062499938548392, 26.74683588394047007 ) ) ;
#53353=CARTESIAN_POINT ( 'NONE',  ( -1.071796769724486120, 15.06740381056766687, 34.00000000000000000 ) ) ;
#53361=CARTESIAN_POINT ( 'NONE',  ( 2.828200636599751609E-16, 14.35624999877096641, 25.38119784648299415 ) ) ;
#53365=ORIENTED_EDGE ( 'NONE', *, *, #51961, .F. ) ;
#53397=CARTESIAN_POINT ( 'NONE',  ( 3.756430356250000546, 18.64062499938548356, 27.83122392262697886 ) ) ;
#53425=CARTESIAN_POINT ( 'NONE',  ( 4.000000000000000000, 14.28124999877096890, 27.69059892324149885 ) ) ;
#53453=DIRECTION ( 'NONE',  ( -0.000000000000000000, -1.000000000000000000, -0.000000000000000000 ) ) ;
#53497=CARTESIAN_POINT ( 'NONE',  ( 1.042938436496270160, 25.50788288962337447, 33.87058137810289793 ) ) ;
#53514=CARTESIAN_POINT ( 'NONE',  ( -1.878215178125001827, 13.39062499938548356, 33.25316411605952283 ) ) ;
#53516=CARTESIAN_POINT ( 'NONE',  ( 4.000000000000000000, 15.23750000000000071, 27.69059892324149530 ) ) ;
#53579=ADVANCED_FACE ( 'NONE', ( #56492 ), #23226, .T. ) ;
#53584=CARTESIAN_POINT ( 'NONE',  ( 3.999999999999998668, 20.50624999877096499, 32.30940107675850470 ) ) ;
#53598=CARTESIAN_POINT ( 'NONE',  ( 1.878215178125000495, 13.72812499938548392, 26.74683588394047007 ) ) ;
#53613=CARTESIAN_POINT ( 'NONE',  ( -1.878215178124999163, 19.99062499938548143, 26.74683588394047007 ) ) ;
#53615=VERTEX_POINT ( 'NONE', #56134 ) ;
#53644=CARTESIAN_POINT ( 'NONE',  ( -3.756430356249999214, 14.74062499938548498, 27.83122392262697531 ) ) ;
#53652=CARTESIAN_POINT ( 'NONE',  ( 4.000000000000000000, 18.80000000000000071, 30.00000000000000000 ) ) ;
#53656=VECTOR ( 'NONE', #58569, 1000.000000000000000 ) ;
#53686=LINE ( 'NONE', #14518, #7770 ) ;
#53708=CARTESIAN_POINT ( 'NONE',  ( 3.756430356249998770, 18.45312499938548001, 32.16877607737302469 ) ) ;
#53718=CARTESIAN_POINT ( 'NONE',  ( -3.756430356250001434, 15.60312499938548392, 32.16877607737301048 ) ) ;
#53726=CARTESIAN_POINT ( 'NONE',  ( -2.000000000000001776, 15.05000000000000071, 33.46410161513775705 ) ) ;
#53735=CARTESIAN_POINT ( 'NONE',  ( -4.000000000000000000, 13.11874999877096570, 30.00000000000000000 ) ) ;
#53768=CARTESIAN_POINT ( 'NONE',  ( -3.756430356250000102, 20.62812499938548072, 30.00000000000000000 ) ) ;
#53784=VERTEX_POINT ( 'NONE', #17322 ) ;
#53804=CARTESIAN_POINT ( 'NONE',  ( -1.071796769724490339, 19.38259618943233775, 26.00000000000000000 ) ) ;
#53892=CARTESIAN_POINT ( 'NONE',  ( 3.756430356250000546, 13.57812499938548711, 27.83122392262697886 ) ) ;
#53894=CARTESIAN_POINT ( 'NONE',  ( -1.999999999999999112, 14.00000000000000000, 26.53589838486224650 ) ) ;
#53975=CARTESIAN_POINT ( 'NONE',  ( 3.756430356250000102, 14.55312499938548321, 30.00000000000000000 ) ) ;
#53987=CARTESIAN_POINT ( 'NONE',  ( 3.756430356250000546, 19.42812499938548143, 27.83122392262697886 ) ) ;
#54020=CARTESIAN_POINT ( 'NONE',  ( 1.878215178125000495, 14.17812499938548321, 26.74683588394047007 ) ) ;
#54071=CARTESIAN_POINT ( 'NONE',  ( -1.071796769724492115, 16.81115380933863435, 34.00000000000000000 ) ) ;
#54074=CARTESIAN_POINT ( 'NONE',  ( -3.756430356250000990, 13.35312499938548392, 32.16877607737301048 ) ) ;
#54081=CARTESIAN_POINT ( 'NONE',  ( 3.756430356250000102, 20.29062499938548569, 30.00000000000000000 ) ) ;
#54090=CARTESIAN_POINT ( 'NONE',  ( 1.878215178124997609, 16.61562499938548143, 33.25316411605952993 ) ) ;
#54104=CARTESIAN_POINT ( 'NONE',  ( -4.000000000000000000, 17.16874999877096641, 30.00000000000000000 ) ) ;
#54137=CARTESIAN_POINT ( 'NONE',  ( -1.878215178124999163, 19.20312499938548356, 26.74683588394047007 ) ) ;
#54167=DIRECTION ( 'NONE',  ( -0.000000000000000000, -1.000000000000000000, -0.000000000000000000 ) ) ;
#54204=VERTEX_POINT ( 'NONE', #15780 ) ;
#54226=CARTESIAN_POINT ( 'NONE',  ( 2.655984681222220721E-16, 13.31562499938548783, 25.66244784525396483 ) ) ;
#54254=CARTESIAN_POINT ( 'NONE',  ( 1.878215178124997609, 20.32812499938548356, 33.25316411605952993 ) ) ;
#54256=CARTESIAN_POINT ( 'NONE',  ( -3.999999999999999556, 14.48750000000000071, 27.69059892324149175 ) ) ;
#54294=CARTESIAN_POINT ( 'NONE',  ( -1.626862140677534273E-15, 17.78749999999999787, 34.00000000000000000 ) ) ;
#54307=ORIENTED_EDGE ( 'NONE', *, *, #29408, .F. ) ;
#54313=AXIS2_PLACEMENT_3D ( 'NONE', #3991, #42414, #47957 ) ;
#54341=CARTESIAN_POINT ( 'NONE',  ( -1.878215178124999163, 14.25312499938548250, 26.74683588394047007 ) ) ;
#54353=CARTESIAN_POINT ( 'NONE',  ( 3.756430356250000102, 19.39062499938548356, 30.00000000000000000 ) ) ;
#54382=CARTESIAN_POINT ( 'NONE',  ( -3.756430356249999214, 15.19062499938548250, 27.83122392262697531 ) ) ;
#54406=DIRECTION ( 'NONE',  ( 1.000000000000000000, 0.000000000000000000, 0.000000000000000000 ) ) ;
#54407=CARTESIAN_POINT ( 'NONE',  ( 0.000000000000000000, 27.50000000000000000, 30.00000000000000000 ) ) ;
#54443=CARTESIAN_POINT ( 'NONE',  ( 1.878215178124997609, 18.86562499938548143, 33.25316411605952993 ) ) ;
#54452=CARTESIAN_POINT ( 'NONE',  ( -7.967954043666661671E-16, 15.67812499938548321, 34.33755215474603517 ) ) ;
#54461=DIRECTION ( 'NONE',  ( -0.000000000000000000, -1.000000000000000000, -0.000000000000000000 ) ) ;
#54467=CARTESIAN_POINT ( 'NONE',  ( 2.000000000000000444, 16.56874999877096499, 26.53589838486224650 ) ) ;
#54489=EDGE_CURVE ( 'NONE', #67390, #46076, #65854, .T. ) ;
#54492=CARTESIAN_POINT ( 'NONE',  ( -2.000000000000001776, 18.64999999999999858, 33.46410161513775705 ) ) ;
#54499=CARTESIAN_POINT ( 'NONE',  ( -1.878215178125001827, 18.90312499938548285, 33.25316411605952283 ) ) ;
#54500=CARTESIAN_POINT ( 'NONE',  ( 0.000000000000000000, 27.50000000000000000, 30.00000000000000000 ) ) ;
#54507=DIRECTION ( 'NONE',  ( -0.000000000000000000, -1.000000000000000000, -0.000000000000000000 ) ) ;
#54533=CARTESIAN_POINT ( 'NONE',  ( -1.999999999999999112, 19.40000000000000213, 26.53589838486224650 ) ) ;
#54558=DIRECTION ( 'NONE',  ( 0.1736433700863484753, 0.000000000000000000, 0.9848086007062769598 ) ) ;
#54570=CARTESIAN_POINT ( 'NONE',  ( 1.999999999999997335, 16.86874999877096570, 33.46410161513775705 ) ) ;
#54578=CARTESIAN_POINT ( 'NONE',  ( 1.878215178125000495, 14.51562499938548356, 26.74683588394047007 ) ) ;
#54585=LINE ( 'NONE', #37953, #40835 ) ;
#54591=CARTESIAN_POINT ( 'NONE',  ( -1.071796769724502107, 16.68259618943233491, 26.00000000000000711 ) ) ;
#54613=CARTESIAN_POINT ( 'NONE',  ( 3.756430356250000546, 19.99062499938548143, 27.83122392262697886 ) ) ;
#54615=CARTESIAN_POINT ( 'NONE',  ( 2.828200636599751609E-16, 13.96250000000000213, 25.38119784648299415 ) ) ;
#54634=CARTESIAN_POINT ( 'NONE',  ( -4.000000000000000888, 15.46250000000000036, 32.30940107675850470 ) ) ;
#54641=CARTESIAN_POINT ( 'NONE',  ( 2.000000000000000444, 18.81874999877096499, 26.53589838486224650 ) ) ;
#54651=ORIENTED_EDGE ( 'NONE', *, *, #13863, .F. ) ;
#54669=CARTESIAN_POINT ( 'NONE',  ( 1.071796769724490783, 12.98615380933863328, 26.00000000000000000 ) ) ;
#54692=DIRECTION ( 'NONE',  ( 0.000000000000000000, 0.000000000000000000, -1.000000000000000000 ) ) ;
#54701=CARTESIAN_POINT ( 'NONE',  ( 1.071796769724485232, 15.74240381056766402, 25.99999999999999645 ) ) ;
#54713=CYLINDRICAL_SURFACE ( 'NONE', #9983, 4.000000000000000000 ) ;
#54732=EDGE_CURVE ( 'NONE', #36300, #29715, #276, .T. ) ;
#54744=CARTESIAN_POINT ( 'NONE',  ( 3.756430356250000546, 14.14062499938548356, 27.83122392262697886 ) ) ;
#54762=EDGE_CURVE ( 'NONE', #69714, #32715, #16150, .T. ) ;
#54791=EDGE_LOOP ( 'NONE', ( #66234, #46413, #3023, #65217 ) ) ;
#54795=CARTESIAN_POINT ( 'NONE',  ( 3.756430356250000102, 15.34062499938548285, 30.00000000000000000 ) ) ;
#54797=DIRECTION ( 'NONE',  ( -0.000000000000000000, -1.000000000000000000, -0.000000000000000000 ) ) ;
#54813=CARTESIAN_POINT ( 'NONE',  ( -3.756430356250000102, 18.71562499938548285, 30.00000000000000000 ) ) ;
#54824=SHAPE_DEFINITION_REPRESENTATION ( #15488, #46217 ) ;
#54829=CARTESIAN_POINT ( 'NONE',  ( 4.000000000000000000, 16.08124999877096784, 27.69059892324149530 ) ) ;
#54833=EDGE_LOOP ( 'NONE', ( #43890, #40845, #25100, #17735 ) ) ;
#54862=CARTESIAN_POINT ( 'NONE',  ( 3.756430356250000546, 19.09062499938548285, 27.83122392262697886 ) ) ;
#54881=CARTESIAN_POINT ( 'NONE',  ( 1.071796769724488785, 19.15759618943233278, 34.00000000000000000 ) ) ;
#54913=DIRECTION ( 'NONE',  ( 1.000000000000000000, 0.000000000000000000, 0.000000000000000000 ) ) ;
#54939=CARTESIAN_POINT ( 'NONE',  ( 2.000000000000000444, 17.01874999877096428, 26.53589838486224650 ) ) ;
#54947=CARTESIAN_POINT ( 'NONE',  ( 3.756430356249998770, 13.95312499938548179, 32.16877607737302469 ) ) ;
#54956=CARTESIAN_POINT ( 'NONE',  ( 4.000000000000000000, 17.03750000000000142, 27.69059892324149885 ) ) ;
#54983=CARTESIAN_POINT ( 'NONE',  ( -3.756430356249999214, 15.07812499938548356, 27.83122392262697531 ) ) ;
#54985=CARTESIAN_POINT ( 'NONE',  ( 1.999999999999997335, 14.67500000000000071, 33.46410161513775705 ) ) ;
#55020=ORIENTED_EDGE ( 'NONE', *, *, #40081, .T. ) ;
#55046=VECTOR ( 'NONE', #4027, 1000.000000000000000 ) ;
#55070=CARTESIAN_POINT ( 'NONE',  ( 3.756430356250000546, 16.39062499938548356, 27.83122392262697886 ) ) ;
#55080=CARTESIAN_POINT ( 'NONE',  ( 3.999999999999998668, 16.45624999877096784, 32.30940107675850470 ) ) ;
#55115=CARTESIAN_POINT ( 'NONE',  ( 3.756430356250000102, 15.90312499938548108, 30.00000000000000000 ) ) ;
#55121=VECTOR ( 'NONE', #46243, 1000.000000000000000 ) ;
#55134=( BOUNDED_CURVE ( )  B_SPLINE_CURVE ( 2, ( #929, #28992, #29708, #23437, #12351, #68879, #57414, #45983, #68519 ),
 .UNSPECIFIED., .F., .F. ) 
 B_SPLINE_CURVE_WITH_KNOTS ( ( 3, 2, 2, 2, 3 ),
 ( 0.7361111111111111605, 0.7407407407407406996, 0.7500000000000000000, 0.7592592592592593004, 0.7638888888888889506 ),
 .UNSPECIFIED. ) 
 CURVE ( )  GEOMETRIC_REPRESENTATION_ITEM ( )  RATIONAL_B_SPLINE_CURVE ( ( 0.9330127018922192983, 0.9330127018922200755, 1.000000000000000000, 0.8660254037844387076, 1.000000000000000000, 0.8660254037844387076, 1.000000000000000000, 0.9330127018922185211, 0.9330127018922192983 ) ) 
 REPRESENTATION_ITEM ( '' )  );
#55161=ORIENTED_EDGE ( 'NONE', *, *, #44604, .T. ) ;
#55170=CARTESIAN_POINT ( 'NONE',  ( -7.967954043666661671E-16, 14.77812499938548463, 34.33755215474603517 ) ) ;
#55176=CARTESIAN_POINT ( 'NONE',  ( -1.878215178124999163, 19.09062499938548285, 26.74683588394047007 ) ) ;
#55186=CARTESIAN_POINT ( 'NONE',  ( 3.756430356249998770, 17.55312499938548143, 32.16877607737302469 ) ) ;
#55203=CARTESIAN_POINT ( 'NONE',  ( 2.828200636599751609E-16, 16.15624999877096712, 25.38119784648299415 ) ) ;
#55245=LINE ( 'NONE', #26804, #18292 ) ;
#55252=ORIENTED_EDGE ( 'NONE', *, *, #10225, .F. ) ;
#55306=LINE ( 'NONE', #9505, #24393 ) ;
#55314=CARTESIAN_POINT ( 'NONE',  ( 1.878215178125000495, 13.16562499938548392, 26.74683588394047007 ) ) ;
#55322=CARTESIAN_POINT ( 'NONE',  ( 2.655984681222220721E-16, 15.56562499938548250, 25.66244784525396483 ) ) ;
#55350=CARTESIAN_POINT ( 'NONE',  ( 3.756430356250000102, 15.79062499938548392, 30.00000000000000000 ) ) ;
#55352=CARTESIAN_POINT ( 'NONE',  ( -1.999999999999999112, 16.25000000000000000, 26.53589838486224650 ) ) ;
#55387=DIRECTION ( 'NONE',  ( 0.000000000000000000, 0.000000000000000000, -1.000000000000000000 ) ) ;
#55412=ADVANCED_FACE ( 'NONE', ( #42318 ), #64844, .T. ) ;
#55426=CARTESIAN_POINT ( 'NONE',  ( 1.138803498474273873E-14, 15.98750000000000249, 34.00000000000000000 ) ) ;
#55435=CARTESIAN_POINT ( 'NONE',  ( 2.655984681222220721E-16, 16.46562499938548285, 25.66244784525396483 ) ) ;
#55447=VERTEX_POINT ( 'NONE', #8695 ) ;
#55477=CARTESIAN_POINT ( 'NONE',  ( -3.756430356250001434, 17.06562499938548427, 32.16877607737301048 ) ) ;
#55484=LINE ( 'NONE', #38864, #41566 ) ;
#55498=CARTESIAN_POINT ( 'NONE',  ( -2.000000000000001776, 20.00000000000000000, 33.46410161513775705 ) ) ;
#55506=EDGE_CURVE ( 'NONE', #67424, #29801, #33287, .T. ) ;
#55532=CARTESIAN_POINT ( 'NONE',  ( -1.878215178125001827, 15.19062499938548427, 33.25316411605952283 ) ) ;
#55546=CARTESIAN_POINT ( 'NONE',  ( 2.655984681222220721E-16, 18.60312499938548214, 25.66244784525396483 ) ) ;
#55561=CARTESIAN_POINT ( 'NONE',  ( 2.000000000000000444, 15.66874999877096464, 26.53589838486224650 ) ) ;
#55594=CARTESIAN_POINT ( 'NONE',  ( -1.999999999999999112, 20.69374999877096499, 26.53589838486224650 ) ) ;
#55600=ORIENTED_EDGE ( 'NONE', *, *, #64818, .T. ) ;
#55628=CARTESIAN_POINT ( 'NONE',  ( 5.810221930991193690E-16, 17.50624999877096499, 26.00000000000000000 ) ) ;
#55673=CARTESIAN_POINT ( 'NONE',  ( 3.756430356249998770, 14.85312499938548392, 32.16877607737302469 ) ) ;
#55678=ADVANCED_FACE ( 'NONE', ( #72950 ), #22332, .T. ) ;
#55682=CARTESIAN_POINT ( 'NONE',  ( 3.756430356249998770, 13.61562499938548321, 32.16877607737301759 ) ) ;
#55711=CARTESIAN_POINT ( 'NONE',  ( 3.756430356250000102, 14.89062499938548356, 30.00000000000000000 ) ) ;
#55713=CARTESIAN_POINT ( 'NONE',  ( -3.999999999999999556, 17.18750000000000000, 27.69059892324149175 ) ) ;
#55781=( BOUNDED_SURFACE ( )  B_SPLINE_SURFACE ( 1, 2, ( 
 ( #58888, #24913, #69275, #30101, #63359, #40841, #53735, #8298, #52998, #12743, #47826, #1678, #30828, #35639, #69631, #42283, #70356, #68910, #18268, #46741, #58161, #35279, #36732, #8662, #57801, #64807, #7565, #36002, #47456, #69989, #59254, #41555, #31193, #13454, #58521, #64441, #52636, #3128, #7931, #53361, #7210, #19359, #2042, #2758, #13101, #52276, #18637, #14197, #41201, #63709, #24553, #41916, #47099, #13833, #4957, #48193, #3502, #37470, #70716, #16025, #61097, #37096, #4596, #59990, #15292, #9760, #26763, #38573, #71459, #10495, #65912, #37831, #43751, #9400, #55561, #60351, #32662, #33023, #32294, #14930, #60720, #65543, #20091, #66276, #15654, #54829, #38193, #55203, #4236, #42648, #10130, #14563, #26021, #31930, #59621, #49295, #48560, #27126, #54467, #71828, #48930, #49660, #3865, #43388, #26388, #21199, #65172, #72188, #21567, #44121, #66648, #20835, #9035, #31565, #54104, #71086, #20460, #43014, #40031, #72916, #39671, #22656, #22298, #6038, #34104, #21936, #67739, #56643, #11223, #28572, #51109, #68105, #50747, #506, #44492, #44850, #40382, #61818, #45206, #5682, #72549, #10852, #11587, #16748, #23016, #17471, #39305, #150, #67386, #27860, #45574, #33747, #62544, #6401, #28933, #50024, #11941, #17112, #67025, #62191, #61458, #68459, #50391, #27490, #34466, #56994, #51469, #56292, #28218, #16385, #38940, #12296, #872, #23379, #45927, #34831, #17821, #33386, #62901, #55922, #57357, #5318, #29652, #7848, #2671, #69549, #25188, #1959, #69190, #46284, #36288, #13370, #35912, #69904, #13015, #52553, #63625, #36646, #30741, #47731, #70270, #18908, #58437, #52913, #18182, #19642, #53273, #23736, #41824, #18550, #24466, #42198, #58072, #41469, #19270 ),
 ( #63988, #1592, #8212, #1230, #68825, #64722, #64356, #52190, #7482, #13747, #47373, #6763, #2311, #14106, #58802, #47014, #30010, #29297, #35553, #30384, #24826, #51827, #40751, #63266, #12658, #35193, #57718, #7123, #24102, #41115, #46650, #65823, #21114, #15205, #60631, #37011, #25936, #54744, #54020, #3036, #37743, #66555, #26302, #20745, #20006, #9312, #10043, #60263, #15567, #9677, #31846, #3777, #8576, #53644, #42927, #44033, #59168, #43667, #14477, #4146, #48476, #43303, #31104, #65451, #38110, #54382, #48839, #59534, #15935, #8946, #25567, #71744, #26678, #65086, #71370, #71000, #31478, #32210, #72096, #49210, #66189, #59907, #32577, #3416, #55115, #20376, #4514, #21480, #27043, #49574, #48108, #70631, #14843, #42559, #37384, #51020, #45840, #50309, #61731, #416, #10769, #50662, #33659, #33302, #17021, #45120, #32939, #5597, #67655, #22214, #39580, #62103, #5950, #11132, #11497, #55477, #55840, #51381, #72831, #56204, #16661, #10407, #21845, #22572, #27769, #34019, #28483, #44768, #28134, #5227, #38857, #56556, #67303, #22925, #17387, #39945, #61008, #45483, #66, #4869, #68015, #72460, #6313, #61372, #38484, #62458, #11856, #34375, #39219, #56908, #27405, #49935, #23292, #28842, #783, #44408, #68377, #66934, #16303, #57632, #18466, #64267, #19186, #47647, #17738, #46199, #7038, #40297, #58716, #30655, #6681, #47286, #29567, #57988, #52466, #69465, #8128, #41029, #53187, #35466, #7398, #13288, #52104, #25103, #29926, #2229, #2584, #1873, #1509, #30295, #35108, #62819, #35825, #58348, #24379, #7759, #24742, #46927, #12211, #52827, #57269, #68740, #24013, #29209, #18823, #18098, #69820, #46562, #41386, #41739, #23655, #63545, #69104, #40659, #63898 ) ),
 .UNSPECIFIED., .F., .F., .T. ) 
 B_SPLINE_SURFACE_WITH_KNOTS ( ( 2, 2 ),
 ( 3, 2, 2, 2, 2, 2, 2, 2, 2, 2, 2, 2, 2, 2, 2, 2, 2, 2, 2, 2, 2, 2, 2, 2, 2, 2, 2, 2, 2, 2, 2, 2, 2, 2, 2, 2, 2, 2, 2, 2, 2, 2, 2, 2, 2, 2, 2, 2, 2, 2, 2, 2, 2, 2, 2, 2, 2, 2, 2, 2, 2, 2, 2, 2, 2, 2, 2, 2, 2, 2, 2, 2, 2, 2, 2, 2, 2, 2, 2, 2, 2, 2, 2, 2, 2, 2, 2, 2, 2, 2, 2, 2, 2, 2, 2, 2, 2, 2, 2, 2, 2, 2, 2, 2, 2, 2, 2, 3 ),
 ( 0.000000000000000000, 1.000000000000000000 ),
 ( 0.000000000000000000, 0.009259259259259258745, 0.01851851851851851749, 0.02777777777777777624, 0.03703703703703703498, 0.04629629629629629373, 0.05555555555555555247, 0.06481481481481481122, 0.07407407407407406996, 0.08333333333333332871, 0.09259259259259258745, 0.1018518518518518462, 0.1111111111111111049, 0.1203703703703703637, 0.1296296296296296224, 0.1388888888888888951, 0.1481481481481481399, 0.1574074074074074125, 0.1666666666666666574, 0.1759259259259259300, 0.1851851851851851749, 0.1944444444444444475, 0.2037037037037036924, 0.2129629629629629650, 0.2222222222222222099, 0.2314814814814814825, 0.2407407407407407274, 0.2500000000000000000, 0.2592592592592592449, 0.2685185185185185452, 0.2777777777777777901, 0.2870370370370370350, 0.2962962962962962798, 0.3055555555555555802, 0.3148148148148148251, 0.3240740740740740700, 0.3333333333333333148, 0.3425925925925926152, 0.3518518518518518601, 0.3611111111111111049, 0.3703703703703703498, 0.3796296296296296502, 0.3888888888888888951, 0.3981481481481481399, 0.4074074074074073848, 0.4166666666666666852, 0.4259259259259259300, 0.4351851851851851749, 0.4444444444444444198, 0.4537037037037037202, 0.4629629629629629650, 0.4722222222222222099, 0.4814814814814814548, 0.4907407407407407551, 0.5000000000000000000, 0.5092592592592593004, 0.5185185185185184897, 0.5277777777777777901, 0.5370370370370370905, 0.5462962962962962798, 0.5555555555555555802, 0.5648148148148147696, 0.5740740740740740700, 0.5833333333333333703, 0.5925925925925925597, 0.6018518518518518601, 0.6111111111111111605, 0.6203703703703703498, 0.6296296296296296502, 0.6388888888888888395, 0.6481481481481481399, 0.6574074074074074403, 0.6666666666666666297, 0.6759259259259259300, 0.6851851851851852304, 0.6944444444444444198, 0.7037037037037037202, 0.7129629629629629095, 0.7222222222222222099, 0.7314814814814815103, 0.7407407407407406996, 0.7500000000000000000, 0.7592592592592593004, 0.7685185185185184897, 0.7777777777777777901, 0.7870370370370370905, 0.7962962962962962798, 0.8055555555555555802, 0.8148148148148147696, 0.8240740740740740700, 0.8333333333333333703, 0.8425925925925925597, 0.8518518518518518601, 0.8611111111111111605, 0.8703703703703703498, 0.8796296296296296502, 0.8888888888888888395, 0.8981481481481481399, 0.9074074074074074403, 0.9166666666666666297, 0.9259259259259259300, 0.9351851851851852304, 0.9444444444444444198, 0.9537037037037037202, 0.9629629629629629095, 0.9722222222222222099, 0.9814814814814815103, 0.9876227255986288478 ),
 .UNSPECIFIED. ) 
 GEOMETRIC_REPRESENTATION_ITEM ( )  RATIONAL_B_SPLINE_SURFACE ( (
 ( 1.000000000000000000, 0.8660254037844387076, 1.000000000000000000, 0.8660254037844387076, 1.000000000000000000, 0.8660254037844387076, 1.000000000000000000, 0.8660254037844387076, 1.000000000000000000, 0.8660254037844387076, 1.000000000000000000, 0.8660254037844387076, 1.000000000000000000, 0.8660254037844387076, 1.000000000000000000, 0.8660254037844387076, 1.000000000000000000, 0.8660254037844387076, 1.000000000000000000, 0.8660254037844387076, 1.000000000000000000, 0.8660254037844387076, 1.000000000000000000, 0.8660254037844387076, 1.000000000000000000, 0.8660254037844387076, 1.000000000000000000, 0.8660254037844387076, 1.000000000000000000, 0.8660254037844387076, 1.000000000000000000, 0.8660254037844387076, 1.000000000000000000, 0.8660254037844387076, 1.000000000000000000, 0.8660254037844387076, 1.000000000000000000, 0.8660254037844387076, 1.000000000000000000, 0.8660254037844387076, 1.000000000000000000, 0.8660254037844387076, 1.000000000000000000, 0.8660254037844387076, 1.000000000000000000, 0.8660254037844387076, 1.000000000000000000, 0.8660254037844387076, 1.000000000000000000, 0.8660254037844387076, 1.000000000000000000, 0.8660254037844387076, 1.000000000000000000, 0.8660254037844387076, 1.000000000000000000, 0.8660254037844387076, 1.000000000000000000, 0.8660254037844387076, 1.000000000000000000, 0.8660254037844387076, 1.000000000000000000, 0.8660254037844387076, 1.000000000000000000, 0.8660254037844387076, 1.000000000000000000, 0.8660254037844387076, 1.000000000000000000, 0.8660254037844387076, 1.000000000000000000, 0.8660254037844387076, 1.000000000000000000, 0.8660254037844387076, 1.000000000000000000, 0.8660254037844387076, 1.000000000000000000, 0.8660254037844387076, 1.000000000000000000, 0.8660254037844387076, 1.000000000000000000, 0.8660254037844387076, 1.000000000000000000, 0.8660254037844387076, 1.000000000000000000, 0.8660254037844387076, 1.000000000000000000, 0.8660254037844387076, 1.000000000000000000, 0.8660254037844387076, 1.000000000000000000, 0.8660254037844387076, 1.000000000000000000, 0.8660254037844387076, 1.000000000000000000, 0.8660254037844387076, 1.000000000000000000, 0.8660254037844387076, 1.000000000000000000, 0.8660254037844387076, 1.000000000000000000, 0.8660254037844387076, 1.000000000000000000, 0.8660254037844387076, 1.000000000000000000, 0.8660254037844387076, 1.000000000000000000, 0.8660254037844387076, 1.000000000000000000, 0.8660254037844387076, 1.000000000000000000, 0.8660254037844387076, 1.000000000000000000, 0.8660254037844387076, 1.000000000000000000, 0.8660254037844387076, 1.000000000000000000, 0.8660254037844387076, 1.000000000000000000, 0.8660254037844387076, 1.000000000000000000, 0.8660254037844387076, 1.000000000000000000, 0.8660254037844387076, 1.000000000000000000, 0.8660254037844387076, 1.000000000000000000, 0.8660254037844387076, 1.000000000000000000, 0.8660254037844387076, 1.000000000000000000, 0.8660254037844387076, 1.000000000000000000, 0.8660254037844387076, 1.000000000000000000, 0.8660254037844387076, 1.000000000000000000, 0.8660254037844387076, 1.000000000000000000, 0.8660254037844387076, 1.000000000000000000, 0.8660254037844387076, 1.000000000000000000, 0.8660254037844387076, 1.000000000000000000, 0.8660254037844387076, 1.000000000000000000, 0.8660254037844387076, 1.000000000000000000, 0.8660254037844387076, 1.000000000000000000, 0.8660254037844387076, 1.000000000000000000, 0.8660254037844387076, 1.000000000000000000, 0.8660254037844387076, 1.000000000000000000, 0.8660254037844387076, 1.000000000000000000, 0.8660254037844387076, 1.000000000000000000, 0.8660254037844387076, 1.000000000000000000, 0.8660254037844387076, 1.000000000000000000, 0.8660254037844387076, 1.000000000000000000, 0.8660254037844387076, 1.000000000000000000, 0.8660254037844387076, 1.000000000000000000, 0.8660254037844387076, 1.000000000000000000, 0.8660254037844387076, 1.000000000000000000, 0.8660254037844387076, 1.000000000000000000, 0.8660254037844387076, 1.000000000000000000, 0.8660254037844387076, 1.000000000000000000, 0.8660254037844387076, 1.000000000000000000, 0.8660254037844387076, 1.000000000000000000, 0.8660254037844387076, 1.000000000000000000, 0.8660254037844387076, 1.000000000000000000, 0.8660254037844387076, 1.000000000000000000, 0.8660254037844387076, 1.000000000000000000, 0.8660254037844387076, 1.000000000000000000, 0.8660254037844387076, 1.000000000000000000, 0.8660254037844387076, 1.000000000000000000, 0.8660254037844387076, 1.000000000000000000, 0.8660254037844387076, 1.000000000000000000, 0.8660254037844387076, 1.000000000000000000, 0.8660254037844387076, 1.000000000000000000, 0.8660254037844387076, 1.000000000000000000, 0.8660254037844387076, 1.000000000000000000, 0.8660254037844387076, 1.000000000000000000, 0.8660254037844387076, 1.000000000000000000, 0.9111407643075507545, 0.9401540804404022733),
 ( 1.000000000000000000, 0.8660254037844387076, 1.000000000000000000, 0.8660254037844387076, 1.000000000000000000, 0.8660254037844387076, 1.000000000000000000, 0.8660254037844387076, 1.000000000000000000, 0.8660254037844387076, 1.000000000000000000, 0.8660254037844387076, 1.000000000000000000, 0.8660254037844387076, 1.000000000000000000, 0.8660254037844387076, 1.000000000000000000, 0.8660254037844387076, 1.000000000000000000, 0.8660254037844387076, 1.000000000000000000, 0.8660254037844387076, 1.000000000000000000, 0.8660254037844387076, 1.000000000000000000, 0.8660254037844387076, 1.000000000000000000, 0.8660254037844387076, 1.000000000000000000, 0.8660254037844387076, 1.000000000000000000, 0.8660254037844387076, 1.000000000000000000, 0.8660254037844387076, 1.000000000000000000, 0.8660254037844387076, 1.000000000000000000, 0.8660254037844387076, 1.000000000000000000, 0.8660254037844387076, 1.000000000000000000, 0.8660254037844387076, 1.000000000000000000, 0.8660254037844387076, 1.000000000000000000, 0.8660254037844387076, 1.000000000000000000, 0.8660254037844387076, 1.000000000000000000, 0.8660254037844387076, 1.000000000000000000, 0.8660254037844387076, 1.000000000000000000, 0.8660254037844387076, 1.000000000000000000, 0.8660254037844387076, 1.000000000000000000, 0.8660254037844387076, 1.000000000000000000, 0.8660254037844387076, 1.000000000000000000, 0.8660254037844387076, 1.000000000000000000, 0.8660254037844387076, 1.000000000000000000, 0.8660254037844387076, 1.000000000000000000, 0.8660254037844387076, 1.000000000000000000, 0.8660254037844387076, 1.000000000000000000, 0.8660254037844387076, 1.000000000000000000, 0.8660254037844387076, 1.000000000000000000, 0.8660254037844387076, 1.000000000000000000, 0.8660254037844387076, 1.000000000000000000, 0.8660254037844387076, 1.000000000000000000, 0.8660254037844387076, 1.000000000000000000, 0.8660254037844387076, 1.000000000000000000, 0.8660254037844387076, 1.000000000000000000, 0.8660254037844387076, 1.000000000000000000, 0.8660254037844387076, 1.000000000000000000, 0.8660254037844387076, 1.000000000000000000, 0.8660254037844387076, 1.000000000000000000, 0.8660254037844387076, 1.000000000000000000, 0.8660254037844387076, 1.000000000000000000, 0.8660254037844387076, 1.000000000000000000, 0.8660254037844387076, 1.000000000000000000, 0.8660254037844387076, 1.000000000000000000, 0.8660254037844387076, 1.000000000000000000, 0.8660254037844387076, 1.000000000000000000, 0.8660254037844387076, 1.000000000000000000, 0.8660254037844387076, 1.000000000000000000, 0.8660254037844387076, 1.000000000000000000, 0.8660254037844387076, 1.000000000000000000, 0.8660254037844387076, 1.000000000000000000, 0.8660254037844387076, 1.000000000000000000, 0.8660254037844387076, 1.000000000000000000, 0.8660254037844387076, 1.000000000000000000, 0.8660254037844387076, 1.000000000000000000, 0.8660254037844387076, 1.000000000000000000, 0.8660254037844387076, 1.000000000000000000, 0.8660254037844387076, 1.000000000000000000, 0.8660254037844387076, 1.000000000000000000, 0.8660254037844387076, 1.000000000000000000, 0.8660254037844387076, 1.000000000000000000, 0.8660254037844387076, 1.000000000000000000, 0.8660254037844387076, 1.000000000000000000, 0.8660254037844387076, 1.000000000000000000, 0.8660254037844387076, 1.000000000000000000, 0.8660254037844387076, 1.000000000000000000, 0.8660254037844387076, 1.000000000000000000, 0.8660254037844387076, 1.000000000000000000, 0.8660254037844387076, 1.000000000000000000, 0.8660254037844387076, 1.000000000000000000, 0.8660254037844387076, 1.000000000000000000, 0.8660254037844387076, 1.000000000000000000, 0.8660254037844387076, 1.000000000000000000, 0.8660254037844387076, 1.000000000000000000, 0.8660254037844387076, 1.000000000000000000, 0.8660254037844387076, 1.000000000000000000, 0.8660254037844387076, 1.000000000000000000, 0.8660254037844387076, 1.000000000000000000, 0.8660254037844387076, 1.000000000000000000, 0.8660254037844387076, 1.000000000000000000, 0.8660254037844387076, 1.000000000000000000, 0.8660254037844387076, 1.000000000000000000, 0.8660254037844387076, 1.000000000000000000, 0.8660254037844387076, 1.000000000000000000, 0.8660254037844387076, 1.000000000000000000, 0.8660254037844387076, 1.000000000000000000, 0.8660254037844387076, 1.000000000000000000, 0.8660254037844387076, 1.000000000000000000, 0.8660254037844387076, 1.000000000000000000, 0.8660254037844387076, 1.000000000000000000, 0.8660254037844387076, 1.000000000000000000, 0.8660254037844387076, 1.000000000000000000, 0.8660254037844387076, 1.000000000000000000, 0.8660254037844387076, 1.000000000000000000, 0.8660254037844387076, 1.000000000000000000, 0.8660254037844387076, 1.000000000000000000, 0.8660254037844387076, 1.000000000000000000, 0.8660254037844387076, 1.000000000000000000, 0.9111407643075507545, 0.9401540804404022733) ) ) 
 REPRESENTATION_ITEM ( '' )  SURFACE ( )  );
#55797=CARTESIAN_POINT ( 'NONE',  ( -7.967954043666661671E-16, 15.79062499938548392, 34.33755215474603517 ) ) ;
#55837=ORIENTED_EDGE ( 'NONE', *, *, #58697, .T. ) ;
#55840=CARTESIAN_POINT ( 'NONE',  ( -1.878215178125001827, 17.10312499938548214, 33.25316411605952283 ) ) ;
#55855=ADVANCED_FACE ( 'NONE', ( #27522 ), #43785, .T. ) ;
#55894=CARTESIAN_POINT ( 'NONE',  ( 2.655984681222220721E-16, 14.10312499938548392, 25.66244784525396483 ) ) ;
#55908=CARTESIAN_POINT ( 'NONE',  ( 3.756430356250000546, 19.42812499938548143, 27.83122392262697886 ) ) ;
#55922=CARTESIAN_POINT ( 'NONE',  ( 3.999999999999998668, 19.60624999877096997, 32.30940107675850470 ) ) ;
#55968=EDGE_CURVE ( 'NONE', #62113, #36300, #60192, .T. ) ;
#55993=CARTESIAN_POINT ( 'NONE',  ( -1.243387493232115393E-14, 16.60624999877096641, 26.00000000000000000 ) ) ;
#56014=CARTESIAN_POINT ( 'NONE',  ( 4.000000000000000000, 12.50000000000000000, 30.00000000000000000 ) ) ;
#56047=CARTESIAN_POINT ( 'NONE',  ( 1.878215178124997609, 14.92812499938548321, 33.25316411605952993 ) ) ;
#56077=CARTESIAN_POINT ( 'NONE',  ( 3.756430356249998770, 14.85312499938548392, 32.16877607737302469 ) ) ;
#56080=CARTESIAN_POINT ( 'NONE',  ( 1.999999999999997335, 17.82499999999999929, 33.46410161513775705 ) ) ;
#56100=CARTESIAN_POINT ( 'NONE',  ( 1.071796769724491227, 20.18615380933863079, 26.00000000000000000 ) ) ;
#56134=CARTESIAN_POINT ( 'NONE',  ( -1.626862140677534273E-15, 19.13749999999999929, 34.00000000000000000 ) ) ;
#56159=CARTESIAN_POINT ( 'NONE',  ( -1.878215178124999163, 16.50312499938548427, 26.74683588394047007 ) ) ;
#56169=CARTESIAN_POINT ( 'NONE',  ( 4.000000000000000000, 18.38750000000000284, 27.69059892324149885 ) ) ;
#56174=ORIENTED_EDGE ( 'NONE', *, *, #1971, .T. ) ;
#56204=CARTESIAN_POINT ( 'NONE',  ( 3.756430356249998770, 17.21562499938548285, 32.16877607737302469 ) ) ;
#56222=( BOUNDED_CURVE ( )  B_SPLINE_CURVE ( 2, ( #40215, #18740, #24657, #64180, #36112, #58633, #51296, #697, #62737 ),
 .UNSPECIFIED., .F., .F. ) 
 B_SPLINE_CURVE_WITH_KNOTS ( ( 3, 2, 2, 2, 3 ),
 ( 0.6527777777777777901, 0.6574074074074074403, 0.6666666666666666297, 0.6759259259259259300, 0.6805555555555555802 ),
 .UNSPECIFIED. ) 
 CURVE ( )  GEOMETRIC_REPRESENTATION_ITEM ( )  RATIONAL_B_SPLINE_CURVE ( ( 0.9330127018922194093, 0.9330127018922194093, 1.000000000000000000, 0.8660254037844387076, 1.000000000000000000, 0.8660254037844387076, 1.000000000000000000, 0.9330127018922194093, 0.9330127018922194093 ) ) 
 REPRESENTATION_ITEM ( '' )  );
#56262=CARTESIAN_POINT ( 'NONE',  ( 3.756430356250000102, 14.89062499938548356, 30.00000000000000000 ) ) ;
#56279=CARTESIAN_POINT ( 'NONE',  ( 1.878215178124997609, 18.41562499938548214, 33.25316411605952993 ) ) ;
#56283=ORIENTED_EDGE ( 'NONE', *, *, #66773, .F. ) ;
#56292=CARTESIAN_POINT ( 'NONE',  ( 3.999999999999998668, 19.15624999877096357, 32.30940107675850470 ) ) ;
#56323=CARTESIAN_POINT ( 'NONE',  ( -4.000000000000000888, 20.80624999877097281, 32.30940107675850470 ) ) ;
#56324=DIRECTION ( 'NONE',  ( 0.000000000000000000, 0.000000000000000000, -1.000000000000000000 ) ) ;
#56372=FACE_OUTER_BOUND ( 'NONE', #46274, .T. ) ;
#56407=CARTESIAN_POINT ( 'NONE',  ( -3.756430356250000990, 15.71562499938548108, 32.16877607737301048 ) ) ;
#56438=CARTESIAN_POINT ( 'NONE',  ( -3.999999999999999556, 18.53749999999999787, 27.69059892324149175 ) ) ;
#56450=CARTESIAN_POINT ( 'NONE',  ( 4.000000000000000000, 13.83124999877096606, 27.69059892324149885 ) ) ;
#56492=FACE_OUTER_BOUND ( 'NONE', #12342, .T. ) ;
#56498=CARTESIAN_POINT ( 'NONE',  ( 0.000000000000000000, 27.50000000000000000, 30.00000000000000000 ) ) ;
#56515=CARTESIAN_POINT ( 'NONE',  ( 2.655984681222220721E-16, 15.11562499938548321, 25.66244784525396483 ) ) ;
#56556=CARTESIAN_POINT ( 'NONE',  ( 3.756430356249998770, 17.66562499938548214, 32.16877607737302469 ) ) ;
#56571=( BOUNDED_CURVE ( )  B_SPLINE_CURVE ( 2, ( #28566, #51820, #39664, #1223, #498, #23729, #10846, #44844, #62183 ),
 .UNSPECIFIED., .F., .F. ) 
 B_SPLINE_CURVE_WITH_KNOTS ( ( 3, 2, 2, 2, 3 ),
 ( 0.5138888888888889506, 0.5185185185185184897, 0.5277777777777777901, 0.5370370370370370905, 0.5416666666666667407 ),
 .UNSPECIFIED. ) 
 CURVE ( )  GEOMETRIC_REPRESENTATION_ITEM ( )  RATIONAL_B_SPLINE_CURVE ( ( 0.9330127018922192983, 0.9330127018922200755, 1.000000000000000000, 0.8660254037844387076, 1.000000000000000000, 0.8660254037844387076, 1.000000000000000000, 0.9330127018922185211, 0.9330127018922192983 ) ) 
 REPRESENTATION_ITEM ( '' )  );
#56581=CARTESIAN_POINT ( 'NONE',  ( 3.999999999999998668, 13.30624999877096570, 32.30940107675850470 ) ) ;
#56611=CARTESIAN_POINT ( 'NONE',  ( -3.756430356249999214, 16.42812499938548143, 27.83122392262697176 ) ) ;
#56613=CARTESIAN_POINT ( 'NONE',  ( 0.000000000000000000, 27.50000000000000000, 30.00000000000000000 ) ) ;
#56628=LINE ( 'NONE', #1576, #21859 ) ;
#56643=CARTESIAN_POINT ( 'NONE',  ( -4.000000000000000888, 17.65624999877096712, 32.30940107675850470 ) ) ;
#56646=FACE_OUTER_BOUND ( 'NONE', #59816, .T. ) ;
#56653=CARTESIAN_POINT ( 'NONE',  ( 1.071796769724495002, 16.00759618943233775, 34.00000000000000000 ) ) ;
#56754=CARTESIAN_POINT ( 'NONE',  ( -3.756430356249999214, 14.29062499938548214, 27.83122392262697176 ) ) ;
#56762=EDGE_CURVE ( 'NONE', #53784, #24717, #37887, .T. ) ;
#56779=ORIENTED_EDGE ( 'NONE', *, *, #55506, .F. ) ;
#56784=CARTESIAN_POINT ( 'NONE',  ( -1.999999999999999112, 19.84999999999999787, 26.53589838486224650 ) ) ;
#56863=ADVANCED_FACE ( 'NONE', ( #18751 ), #343, .T. ) ;
#56868=CARTESIAN_POINT ( 'NONE',  ( -3.756430356249999214, 17.44062499938548427, 27.83122392262697531 ) ) ;
#56908=CARTESIAN_POINT ( 'NONE',  ( -3.756430356249999214, 18.34062499938548640, 27.83122392262697531 ) ) ;
#56933=CARTESIAN_POINT ( 'NONE',  ( 4.000000000000000000, 15.18124999877096570, 27.69059892324149885 ) ) ;
#56963=CARTESIAN_POINT ( 'NONE',  ( 3.756430356250000546, 16.27812499938548285, 27.83122392262697886 ) ) ;
#56982=ORIENTED_EDGE ( 'NONE', *, *, #50916, .T. ) ;
#56994=CARTESIAN_POINT ( 'NONE',  ( -8.484601909799255319E-16, 19.08124999877096784, 34.61880215351700940 ) ) ;
#57004=CARTESIAN_POINT ( 'NONE',  ( 2.000000000000000444, 16.17500000000000071, 26.53589838486224650 ) ) ;
#57005=( BOUNDED_CURVE ( )  B_SPLINE_CURVE ( 2, ( #1760, #17632, #57531, #17275, #57159, #56450, #68270, #69360, #34630 ),
 .UNSPECIFIED., .F., .F. ) 
 B_SPLINE_CURVE_WITH_KNOTS ( ( 3, 2, 2, 2, 3 ),
 ( 0.09722222222222222376, 0.1018518518518518462, 0.1111111111111111049, 0.1203703703703703637, 0.1250000000000000000 ),
 .UNSPECIFIED. ) 
 CURVE ( )  GEOMETRIC_REPRESENTATION_ITEM ( )  RATIONAL_B_SPLINE_CURVE ( ( 0.9330127018922192983, 0.9330127018922194093, 1.000000000000000000, 0.8660254037844387076, 1.000000000000000000, 0.8660254037844387076, 1.000000000000000000, 0.9330127018922191873, 0.9330127018922192983 ) ) 
 REPRESENTATION_ITEM ( '' )  );
#57009=ORIENTED_EDGE ( 'NONE', *, *, #25685, .F. ) ;
#57048=ORIENTED_EDGE ( 'NONE', *, *, #4064, .T. ) ;
#57114=CARTESIAN_POINT ( 'NONE',  ( -1.878215178124999163, 16.50312499938548427, 26.74683588394047007 ) ) ;
#57117=CARTESIAN_POINT ( 'NONE',  ( -1.626862140677534273E-15, 19.98124999877096641, 34.00000000000000000 ) ) ;
#57146=CARTESIAN_POINT ( 'NONE',  ( -2.000000000000001776, 20.44999999999999929, 33.46410161513775705 ) ) ;
#57159=CARTESIAN_POINT ( 'NONE',  ( 4.000000000000000000, 13.79374999877096641, 30.00000000000000000 ) ) ;
#57180=CARTESIAN_POINT ( 'NONE',  ( 5.810221930991193690E-16, 19.75624999877096499, 26.00000000000000000 ) ) ;
#57182=ORIENTED_EDGE ( 'NONE', *, *, #25554, .T. ) ;
#57185=CYLINDRICAL_SURFACE ( 'NONE', #51512, 4.000000000000000000 ) ;
#57213=FACE_OUTER_BOUND ( 'NONE', #14120, .T. ) ;
#57229=CARTESIAN_POINT ( 'NONE',  ( 3.756430356250000546, 18.19062499938548427, 27.83122392262697886 ) ) ;
#57231=CARTESIAN_POINT ( 'NONE',  ( 3.999999999999998668, 13.36250000000000071, 32.30940107675850470 ) ) ;
#57269=CARTESIAN_POINT ( 'NONE',  ( -1.878215178125001827, 20.25312499938548072, 33.25316411605952283 ) ) ;
#57300=CARTESIAN_POINT ( 'NONE',  ( -1.626862140677534273E-15, 15.03124999877096535, 34.00000000000000000 ) ) ;
#57317=CARTESIAN_POINT ( 'NONE',  ( 1.071796769724488785, 15.55759618943233491, 34.00000000000000000 ) ) ;
#57330=CARTESIAN_POINT ( 'NONE',  ( -1.878215178124999163, 17.29062499938548214, 26.74683588394047007 ) ) ;
#57346=VERTEX_POINT ( 'NONE', #31093 ) ;
#57357=CARTESIAN_POINT ( 'NONE',  ( 4.000000000000000000, 19.64374999877096428, 30.00000000000000000 ) ) ;
#57406=ORIENTED_EDGE ( 'NONE', *, *, #17867, .F. ) ;
#57414=CARTESIAN_POINT ( 'NONE',  ( -2.000000000000001776, 19.04374999877096641, 33.46410161513775705 ) ) ;
#57420=CARTESIAN_POINT ( 'NONE',  ( 2.655984681222220721E-16, 15.45312499938548179, 25.66244784525396483 ) ) ;
#57482=CARTESIAN_POINT ( 'NONE',  ( 3.756430356249998770, 16.76562499938548356, 32.16877607737301759 ) ) ;
#57517=CARTESIAN_POINT ( 'NONE',  ( -2.000000000000001776, 20.00000000000000000, 33.46410161513775705 ) ) ;
#57531=CARTESIAN_POINT ( 'NONE',  ( 1.999999999999997335, 13.71874999877096535, 33.46410161513775705 ) ) ;
#57596=CARTESIAN_POINT ( 'NONE',  ( 3.756430356250000546, 17.74062499938548143, 27.83122392262697886 ) ) ;
#57598=CARTESIAN_POINT ( 'NONE',  ( -4.000000000000000888, 13.66250000000000142, 32.30940107675850470 ) ) ;
#57605=DIRECTION ( 'NONE',  ( -0.000000000000000000, -1.000000000000000000, -0.000000000000000000 ) ) ;
#57632=CARTESIAN_POINT ( 'NONE',  ( 2.655984681222220721E-16, 18.71562499938548285, 25.66244784525396483 ) ) ;
#57641=ORIENTED_EDGE ( 'NONE', *, *, #70842, .T. ) ;
#57657=CYLINDRICAL_SURFACE ( 'NONE', #65466, 4.000000000000000000 ) ;
#57659=CARTESIAN_POINT ( 'NONE',  ( 2.000000000000000444, 13.41874999877096641, 26.53589838486224650 ) ) ;
#57689=CARTESIAN_POINT ( 'NONE',  ( 3.756430356250000102, 17.59062499938548285, 30.00000000000000000 ) ) ;
#57718=CARTESIAN_POINT ( 'NONE',  ( 1.878215178125000495, 13.72812499938548392, 26.74683588394047007 ) ) ;
#57741=DIRECTION ( 'NONE',  ( -0.000000000000000000, -1.000000000000000000, -0.000000000000000000 ) ) ;
#57754=EDGE_LOOP ( 'NONE', ( #46380, #29612, #22461, #15717 ) ) ;
#57768=VERTEX_POINT ( 'NONE', #1043 ) ;
#57775=CARTESIAN_POINT ( 'NONE',  ( -1.878215178124999163, 16.84062499938548285, 26.74683588394047007 ) ) ;
#57801=CARTESIAN_POINT ( 'NONE',  ( 4.000000000000000000, 13.79374999877096641, 30.00000000000000000 ) ) ;
#57805=ORIENTED_EDGE ( 'NONE', *, *, #60483, .F. ) ;
#57835=CARTESIAN_POINT ( 'NONE',  ( 2.655984681222220721E-16, 16.01562499938548356, 25.66244784525396483 ) ) ;
#57906=CARTESIAN_POINT ( 'NONE',  ( 4.648177544792955741E-15, 14.18750000000000000, 33.99999999999999289 ) ) ;
#57916=CYLINDRICAL_SURFACE ( 'NONE', #70202, 4.000000000000000000 ) ;
#57934=CARTESIAN_POINT ( 'NONE',  ( 3.593717626727911174, 25.10350949617167160, 28.22432905880962650 ) ) ;
#57950=CARTESIAN_POINT ( 'NONE',  ( -3.756430356250001434, 17.51562499938548356, 32.16877607737301048 ) ) ;
#57952=CARTESIAN_POINT ( 'NONE',  ( -3.756430356250000102, 20.06562499938548072, 30.00000000000000000 ) ) ;
#57988=CARTESIAN_POINT ( 'NONE',  ( -3.756430356249999214, 19.24062499938548143, 27.83122392262697531 ) ) ;
#57999=EDGE_CURVE ( 'NONE', #25000, #29715, #38188, .T. ) ;
#58045=CARTESIAN_POINT ( 'NONE',  ( 3.756430356249998770, 17.10312499938548214, 32.16877607737301759 ) ) ;
#58072=CARTESIAN_POINT ( 'NONE',  ( -2.000000000000001776, 20.84374999877096357, 33.46410161513775705 ) ) ;
#58100=( BOUNDED_CURVE ( )  B_SPLINE_CURVE ( 2, ( #47989, #19153, #7727, #41707, #8093, #24710, #46530, #58316, #70517 ),
 .UNSPECIFIED., .F., .F. ) 
 B_SPLINE_CURVE_WITH_KNOTS ( ( 3, 2, 2, 2, 3 ),
 ( 0.6805555555555555802, 0.6851851851851852304, 0.6944444444444444198, 0.7037037037037037202, 0.7083333333333333703 ),
 .UNSPECIFIED. ) 
 CURVE ( )  GEOMETRIC_REPRESENTATION_ITEM ( )  RATIONAL_B_SPLINE_CURVE ( ( 0.9330127018922194093, 0.9330127018922194093, 1.000000000000000000, 0.8660254037844387076, 1.000000000000000000, 0.8660254037844387076, 1.000000000000000000, 0.9330127018922185211, 0.9330127018922192983 ) ) 
 REPRESENTATION_ITEM ( '' )  );
#58135=CARTESIAN_POINT ( 'NONE',  ( 2.655984681222220721E-16, 18.15312499938548285, 25.66244784525396483 ) ) ;
#58154=CARTESIAN_POINT ( 'NONE',  ( 1.071796769724491227, 17.54240381056766651, 26.00000000000000000 ) ) ;
#58161=CARTESIAN_POINT ( 'NONE',  ( -2.000000000000001776, 13.64374999877096784, 33.46410161513775705 ) ) ;
#58170=CARTESIAN_POINT ( 'NONE',  ( 3.756430356250000102, 12.64062499938548356, 30.00000000000000000 ) ) ;
#58195=CARTESIAN_POINT ( 'NONE',  ( -1.878215178125001827, 16.20312499938548356, 33.25316411605952283 ) ) ;
#58229=CARTESIAN_POINT ( 'NONE',  ( 1.999999999999997335, 19.17500000000000071, 33.46410161513775705 ) ) ;
#58266=CARTESIAN_POINT ( 'NONE',  ( -1.243387493232115393E-14, 15.70624999877096784, 26.00000000000000000 ) ) ;
#58277=CARTESIAN_POINT ( 'NONE',  ( 1.071796769724491227, 17.99240381056766935, 26.00000000000000000 ) ) ;
#58309=CARTESIAN_POINT ( 'NONE',  ( 3.756430356249998770, 19.01562499938548356, 32.16877607737302469 ) ) ;
#58311=CARTESIAN_POINT ( 'NONE',  ( 1.878215178125000495, 19.91562499938548569, 26.74683588394047007 ) ) ;
#58316=CARTESIAN_POINT ( 'NONE',  ( -1.071796769724480347, 18.21740381056766722, 34.00000000000000711 ) ) ;
#58348=CARTESIAN_POINT ( 'NONE',  ( 3.756430356250000546, 19.99062499938548143, 27.83122392262697886 ) ) ;
#58357=VERTEX_POINT ( 'NONE', #65658 ) ;
#58386=ORIENTED_EDGE ( 'NONE', *, *, #70897, .F. ) ;
#58388=CARTESIAN_POINT ( 'NONE',  ( -3.871985432722222509, 25.03371007018978744, 28.96247042170731589 ) ) ;
#58391=CARTESIAN_POINT ( 'NONE',  ( -2.498395430326213790E-14, 19.30624999877096926, 26.00000000000000000 ) ) ;
#58405=CARTESIAN_POINT ( 'NONE',  ( -1.878215178124999163, 18.64062499938548356, 26.74683588394047007 ) ) ;
#58437=CARTESIAN_POINT ( 'NONE',  ( 1.999999999999997335, 20.46874999877096712, 33.46410161513775705 ) ) ;
#58471=AXIS2_PLACEMENT_3D ( 'NONE', #38809, #32163, #15888 ) ;
#58498=CARTESIAN_POINT ( 'NONE',  ( 1.878215178125000495, 17.66562499938548214, 26.74683588394047007 ) ) ;
#58514=CARTESIAN_POINT ( 'NONE',  ( -1.999999999999999112, 13.55000000000000071, 26.53589838486224650 ) ) ;
#58521=CARTESIAN_POINT ( 'NONE',  ( 1.999999999999997335, 14.16874999877096641, 33.46410161513775705 ) ) ;
#58524=CARTESIAN_POINT ( 'NONE',  ( 4.000000000000000000, 19.23124999877096641, 27.69059892324149885 ) ) ;
#58558=CARTESIAN_POINT ( 'NONE',  ( 3.756430356250000546, 16.84062499938548285, 27.83122392262697886 ) ) ;
#58569=DIRECTION ( 'NONE',  ( -0.000000000000000000, -1.000000000000000000, -0.000000000000000000 ) ) ;
#58581=( BOUNDED_CURVE ( )  B_SPLINE_CURVE ( 2, ( #11590, #61100, #10498, #153, #67742, #44853, #72919, #23019, #27129 ),
 .UNSPECIFIED., .F., .F. ) 
 B_SPLINE_CURVE_WITH_KNOTS ( ( 3, 2, 2, 2, 3 ),
 ( 0.5694444444444444198, 0.5740740740740740700, 0.5833333333333333703, 0.5925925925925925597, 0.5972222222222222099 ),
 .UNSPECIFIED. ) 
 CURVE ( )  GEOMETRIC_REPRESENTATION_ITEM ( )  RATIONAL_B_SPLINE_CURVE ( ( 0.9330127018922194093, 0.9330127018922194093, 1.000000000000000000, 0.8660254037844387076, 1.000000000000000000, 0.8660254037844387076, 1.000000000000000000, 0.9330127018922194093, 0.9330127018922194093 ) ) 
 REPRESENTATION_ITEM ( '' )  );
#58599=CARTESIAN_POINT ( 'NONE',  ( -2.498395430326213790E-14, 19.30624999877096926, 26.00000000000000000 ) ) ;
#58633=CARTESIAN_POINT ( 'NONE',  ( 4.000000000000000000, 18.33124999877096784, 27.69059892324149885 ) ) ;
#58655=CARTESIAN_POINT ( 'NONE',  ( 0.000000000000000000, 27.50000000000000000, 30.00000000000000000 ) ) ;
#58661=CARTESIAN_POINT ( 'NONE',  ( 2.441062857229242322, 25.34009520733920340, 26.82048057073465230 ) ) ;
#58676=CARTESIAN_POINT ( 'NONE',  ( -3.756430356250000102, 13.31562499938548427, 30.00000000000000000 ) ) ;
#58678=CARTESIAN_POINT ( 'NONE',  ( -4.000000000000000888, 12.76250000000000284, 32.30940107675850470 ) ) ;
#58697=EDGE_CURVE ( 'NONE', #29564, #28631, #44960, .T. ) ;
#58713=VERTEX_POINT ( 'NONE', #38695 ) ;
#58716=CARTESIAN_POINT ( 'NONE',  ( 3.756430356250000102, 19.05312499938548143, 30.00000000000000000 ) ) ;
#58723=( BOUNDED_CURVE ( )  B_SPLINE_CURVE ( 2, ( #42494, #42857, #9966, #54669, #4073 ),
 .UNSPECIFIED., .F., .F. ) 
 B_SPLINE_CURVE_WITH_KNOTS ( ( 3, 2, 3 ),
 ( 0.000000000000000000, 0.009259259259259258745, 0.01388888888888888985 ),
 .UNSPECIFIED. ) 
 CURVE ( )  GEOMETRIC_REPRESENTATION_ITEM ( )  RATIONAL_B_SPLINE_CURVE ( ( 1.000000000000000000, 0.8660254037844387076, 1.000000000000000000, 0.9330127018922192983, 0.9330127018922194093 ) ) 
 REPRESENTATION_ITEM ( '' )  );
#58743=CARTESIAN_POINT ( 'NONE',  ( 5.000000000000000000, 39.99999999999999289, 15.00000000000000178 ) ) ;
#58754=CARTESIAN_POINT ( 'NONE',  ( -1.042719862598425307, 25.50793469220265663, 33.87077893255365524 ) ) ;
#58771=CARTESIAN_POINT ( 'NONE',  ( -3.756430356249999214, 20.47812499938548569, 27.83122392262697176 ) ) ;
#58802=CARTESIAN_POINT ( 'NONE',  ( 1.878215178125000495, 13.27812499938548285, 26.74683588394047007 ) ) ;
#58864=CARTESIAN_POINT ( 'NONE',  ( 3.756430356250000102, 17.59062499938548285, 30.00000000000000000 ) ) ;
#58873=CARTESIAN_POINT ( 'NONE',  ( -3.756430356250001434, 16.50312499938548783, 32.16877607737301048 ) ) ;
#58888=CARTESIAN_POINT ( 'NONE',  ( 4.000000000000000000, 12.89374999877096606, 30.00000000000000000 ) ) ;
#58917=( BOUNDED_CURVE ( )  B_SPLINE_CURVE ( 2, ( #8584, #70279, #30749, #70639, #53652, #7856, #19650, #13378, #2319 ),
 .UNSPECIFIED., .F., .F. ) 
 B_SPLINE_CURVE_WITH_KNOTS ( ( 3, 2, 2, 2, 3 ),
 ( 0.7638888888888889506, 0.7685185185185184897, 0.7777777777777777901, 0.7870370370370370905, 0.7916666666666667407 ),
 .UNSPECIFIED. ) 
 CURVE ( )  GEOMETRIC_REPRESENTATION_ITEM ( )  RATIONAL_B_SPLINE_CURVE ( ( 0.9330127018922192983, 0.9330127018922200755, 1.000000000000000000, 0.8660254037844387076, 1.000000000000000000, 0.8660254037844387076, 1.000000000000000000, 0.9330127018922185211, 0.9330127018922192983 ) ) 
 REPRESENTATION_ITEM ( '' )  );
#58921=CARTESIAN_POINT ( 'NONE',  ( 3.756430356250000102, 18.60312499938548214, 30.00000000000000000 ) ) ;
#58983=( BOUNDED_CURVE ( )  B_SPLINE_CURVE ( 2, ( #48865, #20771, #43327, #15590, #44431, #16325, #66959, #21869, #11158 ),
 .UNSPECIFIED., .F., .F. ) 
 B_SPLINE_CURVE_WITH_KNOTS ( ( 3, 2, 2, 2, 3 ),
 ( 0.06944444444444444753, 0.07407407407407406996, 0.08333333333333332871, 0.09259259259259258745, 0.09722222222222222376 ),
 .UNSPECIFIED. ) 
 CURVE ( )  GEOMETRIC_REPRESENTATION_ITEM ( )  RATIONAL_B_SPLINE_CURVE ( ( 0.9330127018922192983, 0.9330127018922194093, 1.000000000000000000, 0.8660254037844387076, 1.000000000000000000, 0.8660254037844387076, 1.000000000000000000, 0.9330127018922191873, 0.9330127018922192983 ) ) 
 REPRESENTATION_ITEM ( '' )  );
#58997=FACE_OUTER_BOUND ( 'NONE', #72844, .T. ) ;
#59024=CARTESIAN_POINT ( 'NONE',  ( 2.000000000000000444, 13.47500000000000142, 26.53589838486224650 ) ) ;
#59041=CARTESIAN_POINT ( 'NONE',  ( -3.756430356249999214, 19.69062499938548427, 27.83122392262697531 ) ) ;
#59043=CARTESIAN_POINT ( 'NONE',  ( 4.000000000000000000, 13.88750000000000107, 27.69059892324149530 ) ) ;
#59124=CARTESIAN_POINT ( 'NONE',  ( -3.756430356249999214, 12.94062499938548250, 27.83122392262697531 ) ) ;
#59137=CARTESIAN_POINT ( 'NONE',  ( -3.756430356250000990, 20.55312499938548143, 32.16877607737301048 ) ) ;
#59168=CARTESIAN_POINT ( 'NONE',  ( -1.878215178125001827, 14.85312499938548214, 33.25316411605952283 ) ) ;
#59191=CARTESIAN_POINT ( 'NONE',  ( -1.626862140677534273E-15, 15.93124999877096748, 34.00000000000000000 ) ) ;
#59196=EDGE_CURVE ( 'NONE', #13067, #72457, #45150, .T. ) ;
#59197=( BOUNDED_CURVE ( )  B_SPLINE_CURVE ( 2, ( #49056, #4361, #9884, #71948, #21324, #43877, #65294, #38322, #15779, #31691, #60847, #37225, #15054, #10254, #37592, #54226, #2882, #48686, #71209, #20586, #43141, #60113, #61574, #55682, #34221, #27612, #28688, #67861, #62668, #4716, #21690, #16149, #50148, #49784, #5079, #72676, #27979, #67503, #39060, #22418, #22059, #56754, #68227, #10977, #61221, #264, #28328, #61943, #10615, #39792, #44246, #33145, #22774, #50866, #67147, #33498, #11347, #66777, #56047, #44617, #50509, #45325, #45693, #51227, #16507, #27250, #23138, #17590, #5439, #44965, #38701, #40149, #73035, #17232, #12063, #55322, #72308, #33864, #16867, #56407, #39422, #5798, #62309, #11705, #6159, #631, #13490, #57835, #34586, #52309, #18304, #63023, #58195, #40875, #34954, #36038, #6886, #7966, #47132, #41953, #57114, #13133, #63392, #46773, #1711, #7244, #19029, #57482, #995, #58558, #7598, #30502, #12777, #64105, #18670, #35313, #24947, #30137, #52668, #53030, #2424, #29773, #41232, #23502, #51595, #6526, #70021, #12422, #2075, #47491, #24224, #35672, #41587, #29058, #64473, #69309, #24584, #29419, #69663, #46050, #51952, #68585, #19392, #63744, #17946, #40508, #1352, #23861, #46409, #68946, #8329, #43047, #20126, #37865, #31226, #14963, #58921, #53397, #30859, #37128, #43784, #31961, #43422, #65944, #54499, #4270, #9792, #3163, #36408, #54862, #26794, #36768, #54137, #70390, #49328, #2790, #9433, #71860, #21232, #25315, #20491, #3900, #70751, #60021, #47861, #3532, #13867, #26054, #42681, #15324, #59657, #19766, #31600, #65204, #42317, #37501, #14593, #14230, #60384, #59285, #32325, #26421, #64843, #8694, #65573, #9066, #48594, #71119, #48962, #71492, #53768, #25692, #48227, #20869, #38974 ),
 .UNSPECIFIED., .F., .F. ) 
 B_SPLINE_CURVE_WITH_KNOTS ( ( 3, 2, 2, 2, 2, 2, 2, 2, 2, 2, 2, 2, 2, 2, 2, 2, 2, 2, 2, 2, 2, 2, 2, 2, 2, 2, 2, 2, 2, 2, 2, 2, 2, 2, 2, 2, 2, 2, 2, 2, 2, 2, 2, 2, 2, 2, 2, 2, 2, 2, 2, 2, 2, 2, 2, 2, 2, 2, 2, 2, 2, 2, 2, 2, 2, 2, 2, 2, 2, 2, 2, 2, 2, 2, 2, 2, 2, 2, 2, 2, 2, 2, 2, 2, 2, 2, 2, 2, 2, 2, 2, 2, 2, 2, 2, 2, 2, 2, 2, 2, 2, 2, 2, 2, 2, 2, 2, 3 ),
 ( 0.000000000000000000, 0.009375299918951271114, 0.01875059983790254223, 0.02812589975685381508, 0.03750119967580508445, 0.04687649959475635730, 0.05625179951370763015, 0.06562709943265890300, 0.07500239935161016891, 0.08437769927056144870, 0.09375299918951271461, 0.1031282991084639805, 0.1125035990274152603, 0.1218788989463665262, 0.1312541988653178060, 0.1406294987842690858, 0.1500047987032203378, 0.1593800986221716176, 0.1687553985411228974, 0.1781306984600741772, 0.1875059983790254292, 0.1968812982979767090, 0.2062565982169279610, 0.2156318981358792686, 0.2250071980548305206, 0.2343824979737818004, 0.2437577978927330524, 0.2531330978116843600, 0.2625083977306356120, 0.2718836976495869195, 0.2812589975685381716, 0.2906342974874894236, 0.3000095974064406756, 0.3093848973253919832, 0.3187601972443432352, 0.3281354971632944872, 0.3375107970822457948, 0.3468860970011971023, 0.3562613969201483544, 0.3656366968390996064, 0.3750119967580508584, 0.3843872966770021660, 0.3937625965959534180, 0.4031378965149046700, 0.4125131964338559221, 0.4218884963528072296, 0.4312637962717585371, 0.4406390961907097892, 0.4500143961096610412, 0.4593896960286123488, 0.4687649959475636008, 0.4781402958665148528, 0.4875155957854661049, 0.4968908957044174124, 0.5062661956233687199, 0.5156414955423199720, 0.5250167954612712240, 0.5343920953802224760, 0.5437673952991738391, 0.5531426952181249801, 0.5625179951370763431, 0.5718932950560274842, 0.5812685949749788472, 0.5906438948939302103, 0.6000191948128813513, 0.6093944947318327143, 0.6187697946507839664, 0.6281450945697352184, 0.6375203944886864704, 0.6468956944076377225, 0.6562709943265889745, 0.6656462942455403375, 0.6750215941644915896, 0.6843968940834428416, 0.6937721940023942047, 0.7031474939213453457, 0.7125227938402967087, 0.7218980937592478497, 0.7312733936781992128, 0.7406486935971504648, 0.7500239935161017168, 0.7593992934350529689, 0.7687745933540043319, 0.7781498932729555840, 0.7875251931919068360, 0.7969004931108581991, 0.8062757930298093401, 0.8156510929487607031, 0.8250263928677118441, 0.8344016927866632072, 0.8437769927056144592, 0.8531522926245657112, 0.8625275925435170743, 0.8719028924624683263, 0.8812781923814195784, 0.8906534923003708304, 0.9000287922193220824, 0.9094040921382733345, 0.9187793920572246975, 0.9281546919761758385, 0.9375299918951272016, 0.9469052918140784536, 0.9562805917330297056, 0.9656558916519810687, 0.9750311915709322097, 0.9844064914898835728, 0.9937817914088348248, 1.000000000000000000 ),
 .UNSPECIFIED. ) 
 CURVE ( )  GEOMETRIC_REPRESENTATION_ITEM ( )  RATIONAL_B_SPLINE_CURVE ( ( 1.000000000000000000, 0.8660254037844387076, 1.000000000000000000, 0.8660254037844387076, 1.000000000000000000, 0.8660254037844387076, 1.000000000000000000, 0.8660254037844387076, 1.000000000000000000, 0.8660254037844387076, 1.000000000000000000, 0.8660254037844387076, 1.000000000000000000, 0.8660254037844387076, 1.000000000000000000, 0.8660254037844387076, 1.000000000000000000, 0.8660254037844387076, 1.000000000000000000, 0.8660254037844387076, 1.000000000000000000, 0.8660254037844387076, 1.000000000000000000, 0.8660254037844387076, 1.000000000000000000, 0.8660254037844387076, 1.000000000000000000, 0.8660254037844387076, 1.000000000000000000, 0.8660254037844387076, 1.000000000000000000, 0.8660254037844387076, 1.000000000000000000, 0.8660254037844387076, 1.000000000000000000, 0.8660254037844387076, 1.000000000000000000, 0.8660254037844387076, 1.000000000000000000, 0.8660254037844387076, 1.000000000000000000, 0.8660254037844387076, 1.000000000000000000, 0.8660254037844387076, 1.000000000000000000, 0.8660254037844387076, 1.000000000000000000, 0.8660254037844387076, 1.000000000000000000, 0.8660254037844387076, 1.000000000000000000, 0.8660254037844387076, 1.000000000000000000, 0.8660254037844387076, 1.000000000000000000, 0.8660254037844387076, 1.000000000000000000, 0.8660254037844387076, 1.000000000000000000, 0.8660254037844387076, 1.000000000000000000, 0.8660254037844387076, 1.000000000000000000, 0.8660254037844387076, 1.000000000000000000, 0.8660254037844387076, 1.000000000000000000, 0.8660254037844387076, 1.000000000000000000, 0.8660254037844387076, 1.000000000000000000, 0.8660254037844387076, 1.000000000000000000, 0.8660254037844387076, 1.000000000000000000, 0.8660254037844387076, 1.000000000000000000, 0.8660254037844387076, 1.000000000000000000, 0.8660254037844387076, 1.000000000000000000, 0.8660254037844387076, 1.000000000000000000, 0.8660254037844387076, 1.000000000000000000, 0.8660254037844387076, 1.000000000000000000, 0.8660254037844387076, 1.000000000000000000, 0.8660254037844387076, 1.000000000000000000, 0.8660254037844387076, 1.000000000000000000, 0.8660254037844387076, 1.000000000000000000, 0.8660254037844387076, 1.000000000000000000, 0.8660254037844387076, 1.000000000000000000, 0.8660254037844387076, 1.000000000000000000, 0.8660254037844387076, 1.000000000000000000, 0.8660254037844387076, 1.000000000000000000, 0.8660254037844387076, 1.000000000000000000, 0.8660254037844387076, 1.000000000000000000, 0.8660254037844387076, 1.000000000000000000, 0.8660254037844387076, 1.000000000000000000, 0.8660254037844387076, 1.000000000000000000, 0.8660254037844387076, 1.000000000000000000, 0.8660254037844387076, 1.000000000000000000, 0.8660254037844387076, 1.000000000000000000, 0.8660254037844387076, 1.000000000000000000, 0.8660254037844387076, 1.000000000000000000, 0.8660254037844387076, 1.000000000000000000, 0.8660254037844387076, 1.000000000000000000, 0.8660254037844387076, 1.000000000000000000, 0.8660254037844387076, 1.000000000000000000, 0.8660254037844387076, 1.000000000000000000, 0.8660254037844387076, 1.000000000000000000, 0.8660254037844387076, 1.000000000000000000, 0.8660254037844387076, 1.000000000000000000, 0.8660254037844387076, 1.000000000000000000, 0.8660254037844387076, 1.000000000000000000, 0.8660254037844387076, 1.000000000000000000, 0.8660254037844387076, 1.000000000000000000, 0.8660254037844387076, 1.000000000000000000, 0.8660254037844387076, 1.000000000000000000, 0.8660254037844387076, 1.000000000000000000, 0.8660254037844387076, 1.000000000000000000, 0.8660254037844387076, 1.000000000000000000, 0.8660254037844387076, 1.000000000000000000, 0.8660254037844387076, 1.000000000000000000, 0.8660254037844387076, 1.000000000000000000, 0.8660254037844387076, 1.000000000000000000, 0.8660254037844387076, 1.000000000000000000, 0.8660254037844387076, 1.000000000000000000, 0.8660254037844387076, 1.000000000000000000, 0.8660254037844387076, 1.000000000000000000, 0.8660254037844387076, 1.000000000000000000, 0.8660254037844387076, 1.000000000000000000, 0.8660254037844387076, 1.000000000000000000, 0.8660254037844387076, 1.000000000000000000, 0.8660254037844387076, 1.000000000000000000, 0.8660254037844387076, 1.000000000000000000, 0.8660254037844387076, 1.000000000000000000, 0.8660254037844387076, 1.000000000000000000, 0.8660254037844387076, 1.000000000000000000, 0.8660254037844387076, 1.000000000000000000, 0.8660254037844387076, 1.000000000000000000, 0.8660254037844387076, 1.000000000000000000, 0.8660254037844387076, 1.000000000000000000, 0.8660254037844387076, 1.000000000000000000, 0.8660254037844387076, 1.000000000000000000, 0.8660254037844387076, 1.000000000000000000, 0.8660254037844387076, 1.000000000000000000, 0.8660254037844387076, 1.000000000000000000, 0.8660254037844387076, 1.000000000000000000, 0.9111407643075507545, 0.9401540804404022733 ) ) 
 REPRESENTATION_ITEM ( '' )  );
#59214=VERTEX_POINT ( 'NONE', #7237 ) ;
#59225=ORIENTED_EDGE ( 'NONE', *, *, #25685, .T. ) ;
#59229=CARTESIAN_POINT ( 'NONE',  ( -7.967954043666661671E-16, 18.37812499938548427, 34.33755215474603517 ) ) ;
#59238=CARTESIAN_POINT ( 'NONE',  ( -3.756430356250001434, 16.05312499938548143, 32.16877607737301048 ) ) ;
#59246=CARTESIAN_POINT ( 'NONE',  ( -1.071796769724489229, 13.71740381056766722, 34.00000000000000000 ) ) ;
#59254=CARTESIAN_POINT ( 'NONE',  ( -4.000000000000000000, 14.01874999877096606, 30.00000000000000000 ) ) ;
#59285=CARTESIAN_POINT ( 'NONE',  ( -3.756430356250000990, 20.21562499938548285, 32.16877607737301048 ) ) ;
#59316=CARTESIAN_POINT ( 'NONE',  ( 4.898587196589412829E-16, 27.50000000000000000, 34.00000000000000000 ) ) ;
#59338=CARTESIAN_POINT ( 'NONE',  ( 3.999999999999998668, 19.60624999877096641, 32.30940107675850470 ) ) ;
#59362=( BOUNDED_CURVE ( )  B_SPLINE_CURVE ( 2, ( #31252, #3925, #37526, #13892, #9090, #53425, #43074, #70417, #42344 ),
 .UNSPECIFIED., .F., .F. ) 
 B_SPLINE_CURVE_WITH_KNOTS ( ( 3, 2, 2, 2, 3 ),
 ( 0.1527777777777777901, 0.1574074074074074125, 0.1666666666666666574, 0.1759259259259259300, 0.1805555555555555525 ),
 .UNSPECIFIED. ) 
 CURVE ( )  GEOMETRIC_REPRESENTATION_ITEM ( )  RATIONAL_B_SPLINE_CURVE ( ( 0.9330127018922194093, 0.9330127018922195203, 1.000000000000000000, 0.8660254037844387076, 1.000000000000000000, 0.8660254037844387076, 1.000000000000000000, 0.9330127018922194093, 0.9330127018922194093 ) ) 
 REPRESENTATION_ITEM ( '' )  );
#59396=FACE_OUTER_BOUND ( 'NONE', #24154, .T. ) ;
#59406=CARTESIAN_POINT ( 'NONE',  ( 3.756430356250000546, 13.12812499938548250, 27.83122392262697886 ) ) ;
#59408=CARTESIAN_POINT ( 'NONE',  ( -3.999999999999999556, 15.38750000000000107, 27.69059892324149175 ) ) ;
#59479=CARTESIAN_POINT ( 'NONE',  ( 1.071796769724488785, 16.45759618943233704, 34.00000000000000000 ) ) ;
#59487=CARTESIAN_POINT ( 'NONE',  ( -3.794299971169996066, 25.05385333968535733, 28.70714863339405554 ) ) ;
#59491=CARTESIAN_POINT ( 'NONE',  ( 3.756430356250000102, 12.75312499938548427, 30.00000000000000000 ) ) ;
#59502=CARTESIAN_POINT ( 'NONE',  ( -7.967954043666661671E-16, 20.17812499938548143, 34.33755215474603517 ) ) ;
#59534=CARTESIAN_POINT ( 'NONE',  ( -3.756430356250001434, 15.26562499938548356, 32.16877607737301048 ) ) ;
#59560=CARTESIAN_POINT ( 'NONE',  ( 1.999999999999997335, 15.96874999877096535, 33.46410161513775705 ) ) ;
#59573=ORIENTED_EDGE ( 'NONE', *, *, #68005, .T. ) ;
#59579=DIRECTION ( 'NONE',  ( -0.000000000000000000, -1.000000000000000000, -0.000000000000000000 ) ) ;
#59587=CARTESIAN_POINT ( 'NONE',  ( -3.999999999999999112, 16.68124999877096570, 27.69059892324149530 ) ) ;
#59592=ORIENTED_EDGE ( 'NONE', *, *, #8903, .F. ) ;
#59597=CARTESIAN_POINT ( 'NONE',  ( 1.878215178125000495, 19.46562499938548640, 26.74683588394047007 ) ) ;
#59606=CARTESIAN_POINT ( 'NONE',  ( 1.878215178125000495, 16.76562499938548356, 26.74683588394047007 ) ) ;
#59614=CARTESIAN_POINT ( 'NONE',  ( -3.999999999999999112, 13.58750000000000213, 27.69059892324149530 ) ) ;
#59621=CARTESIAN_POINT ( 'NONE',  ( 1.999999999999997335, 16.41874999877096641, 33.46410161513775705 ) ) ;
#59654=CARTESIAN_POINT ( 'NONE',  ( -3.486133158594716510E-16, 12.61250000000000426, 26.00000000000000355 ) ) ;
#59657=CARTESIAN_POINT ( 'NONE',  ( 1.878215178124997609, 19.87812499938548072, 33.25316411605952993 ) ) ;
#59694=CARTESIAN_POINT ( 'NONE',  ( -4.000000000000000000, 18.06874999877096855, 30.00000000000000000 ) ) ;
#59746=DIRECTION ( 'NONE',  ( -0.000000000000000000, -1.000000000000000000, -0.000000000000000000 ) ) ;
#59751=CARTESIAN_POINT ( 'NONE',  ( -1.071796769724480347, 16.86740381056766580, 34.00000000000000711 ) ) ;
#59760=ORIENTED_EDGE ( 'NONE', *, *, #6118, .F. ) ;
#59772=AXIS2_PLACEMENT_3D ( 'NONE', #62011, #16934, #55387 ) ;
#59777=CARTESIAN_POINT ( 'NONE',  ( -3.756430356250001434, 20.21562499938548285, 32.16877607737301048 ) ) ;
#59779=CARTESIAN_POINT ( 'NONE',  ( -8.484601909799255319E-16, 15.53749999999999964, 34.61880215351700940 ) ) ;
#59816=EDGE_LOOP ( 'NONE', ( #6299, #26071, #67905, #34749 ) ) ;
#59834=EDGE_CURVE ( 'NONE', #11370, #49299, #32857, .T. ) ;
#59860=CARTESIAN_POINT ( 'NONE',  ( 4.000000000000000000, 17.84374999877096712, 30.00000000000000000 ) ) ;
#59864=CARTESIAN_POINT ( 'NONE',  ( 2.655984681222220721E-16, 14.66562499938548214, 25.66244784525396483 ) ) ;
#59875=CARTESIAN_POINT ( 'NONE',  ( 1.878215178125000495, 19.01562499938548356, 26.74683588394047007 ) ) ;
#59907=CARTESIAN_POINT ( 'NONE',  ( -7.967954043666661671E-16, 15.79062499938548392, 34.33755215474603517 ) ) ;
#59931=CARTESIAN_POINT ( 'NONE',  ( 4.000000000000000000, 16.08124999877096784, 27.69059892324149885 ) ) ;
#59950=CYLINDRICAL_SURFACE ( 'NONE', #677, 4.000000000000000000 ) ;
#59960=CARTESIAN_POINT ( 'NONE',  ( 3.756430356249998770, 13.50312499938548427, 32.16877607737301759 ) ) ;
#59966=CARTESIAN_POINT ( 'NONE',  ( -3.756430356250000102, 20.51562499938548356, 30.00000000000000000 ) ) ;
#59975=CARTESIAN_POINT ( 'NONE',  ( 3.756430356250000546, 17.17812499938548143, 27.83122392262697886 ) ) ;
#59990=CARTESIAN_POINT ( 'NONE',  ( 2.828200636599751609E-16, 15.25624999877096499, 25.38119784648299415 ) ) ;
#60021=CARTESIAN_POINT ( 'NONE',  ( 2.655984681222220721E-16, 19.61562499938548143, 25.66244784525396483 ) ) ;
#60027=ORIENTED_EDGE ( 'NONE', *, *, #15468, .F. ) ;
#60031=CARTESIAN_POINT ( 'NONE',  ( -2.498395430326213790E-14, 20.26249999999999929, 26.00000000000000000 ) ) ;
#60104=CARTESIAN_POINT ( 'NONE',  ( 1.878215178124997609, 14.81562499938548427, 33.25316411605952993 ) ) ;
#60113=CARTESIAN_POINT ( 'NONE',  ( -7.967954043666661671E-16, 13.54062499938548214, 34.33755215474603517 ) ) ;
#60139=CARTESIAN_POINT ( 'NONE',  ( 3.756430356249998770, 19.91562499938548214, 32.16877607737302469 ) ) ;
#60141=CARTESIAN_POINT ( 'NONE',  ( -8.484601909799255319E-16, 15.98750000000000249, 34.61880215351700940 ) ) ;
#60142=CARTESIAN_POINT ( 'NONE',  ( -3.999999999999999112, 17.18750000000000000, 27.69059892324149530 ) ) ;
#60147=CARTESIAN_POINT ( 'NONE',  ( 0.000000000000000000, 27.50000000000000000, 26.00000000000000000 ) ) ;
#60166=CARTESIAN_POINT ( 'NONE',  ( 1.999999999999997335, 18.66874999877096641, 33.46410161513775705 ) ) ;
#60175=CARTESIAN_POINT ( 'NONE',  ( -3.999999999999999112, 17.63749999999999929, 27.69059892324149530 ) ) ;
#60192=LINE ( 'NONE', #4071, #17034 ) ;
#60221=CARTESIAN_POINT ( 'NONE',  ( 3.756430356250000102, 13.65312499938548285, 30.00000000000000000 ) ) ;
#60263=CARTESIAN_POINT ( 'NONE',  ( 3.756430356249998770, 14.51562499938548356, 32.16877607737302469 ) ) ;
#60287=CARTESIAN_POINT ( 'NONE',  ( 1.071796769724479237, 20.24240381056766935, 25.99999999999999645 ) ) ;
#60301=VERTEX_POINT ( 'NONE', #50417 ) ;
#60319=CARTESIAN_POINT ( 'NONE',  ( 4.648177544792955741E-15, 14.18750000000000000, 33.99999999999999289 ) ) ;
#60326=CARTESIAN_POINT ( 'NONE',  ( 3.756430356250000546, 20.32812499938548356, 27.83122392262697886 ) ) ;
#60336=CARTESIAN_POINT ( 'NONE',  ( -1.878215178124999163, 17.74062499938548498, 26.74683588394047007 ) ) ;
#60351=CARTESIAN_POINT ( 'NONE',  ( 2.828200636599751609E-16, 15.70624999877096606, 25.38119784648299415 ) ) ;
#60360=CARTESIAN_POINT ( 'NONE',  ( -4.000000000000000000, 16.26874999877096784, 30.00000000000000000 ) ) ;
#60377=CARTESIAN_POINT ( 'NONE',  ( -1.999999999999999112, 18.50000000000000000, 26.53589838486224650 ) ) ;
#60384=CARTESIAN_POINT ( 'NONE',  ( -3.756430356250000102, 20.17812499938548143, 30.00000000000000000 ) ) ;
#60398=ORIENTED_EDGE ( 'NONE', *, *, #55968, .T. ) ;
#60413=ORIENTED_EDGE ( 'NONE', *, *, #20857, .T. ) ;
#60466=CARTESIAN_POINT ( 'NONE',  ( 3.756430356249998770, 13.50312499938548250, 32.16877607737302469 ) ) ;
#60476=CARTESIAN_POINT ( 'NONE',  ( 4.000000000000000000, 17.00000000000000000, 30.00000000000000000 ) ) ;
#60483=EDGE_CURVE ( 'NONE', #41970, #8994, #2215, .T. ) ;
#60495=LINE ( 'NONE', #14703, #37860 ) ;
#60504=CARTESIAN_POINT ( 'NONE',  ( -3.756430356249999214, 15.52812499938548108, 27.83122392262697531 ) ) ;
#60506=CARTESIAN_POINT ( 'NONE',  ( 4.000000000000000000, 14.30000000000000071, 30.00000000000000000 ) ) ;
#60541=EDGE_LOOP ( 'NONE', ( #35147, #8182, #56174, #51742 ) ) ;
#60559=EDGE_CURVE ( 'NONE', #35360, #57346, #52935, .T. ) ;
#60574=CARTESIAN_POINT ( 'NONE',  ( 0.000000000000000000, 27.50000000000000000, 26.00000000000000000 ) ) ;
#60590=CARTESIAN_POINT ( 'NONE',  ( 2.655984681222220721E-16, 13.76562499938548179, 25.66244784525396483 ) ) ;
#60631=CARTESIAN_POINT ( 'NONE',  ( 1.878215178124997609, 14.02812499938548285, 33.25316411605952993 ) ) ;
#60649=B_SPLINE_CURVE_WITH_KNOTS ( 'NONE', 3,
 ( #7437, #1915, #29963, #58754, #65404, #36240, #41778, #24780, #25142, #47324, #8899, #13326, #69857, #19224, #31057, #52504, #25517, #36600, #35865, #58388, #59487, #2989, #48062, #13697, #8164, #64676, #46968, #30693, #7801, #53224, #70219, #3369, #30338, #14061 ),
 .UNSPECIFIED., .F., .F.,
 ( 4, 2, 2, 2, 2, 2, 2, 2, 2, 2, 2, 2, 2, 2, 2, 2, 4 ),
 ( 0.01256276550582235453, 0.01334772285915210993, 0.01413268021248186360, 0.01491763756581161900, 0.01570259491914137440, 0.01648755227247112806, 0.01727250962580088173, 0.01805746697913063886, 0.01884242433246039253, 0.01962738168579014619, 0.02041233903911990333, 0.02119729639244965352, 0.02198225374577941066, 0.02276721109910916432, 0.02355216845243891799, 0.02433712580576867512, 0.02512208315909842879 ),
 .UNSPECIFIED. ) ;
#60658=DIRECTION ( 'NONE',  ( -0.000000000000000000, -1.000000000000000000, -0.000000000000000000 ) ) ;
#60686=CARTESIAN_POINT ( 'NONE',  ( 1.878215178125000495, 14.96562499938548463, 26.74683588394047007 ) ) ;
#60693=CARTESIAN_POINT ( 'NONE',  ( -3.756430356250001434, 18.75312499938548427, 32.16877607737301048 ) ) ;
#60702=CARTESIAN_POINT ( 'NONE',  ( 3.756430356250000546, 18.97812499938548214, 27.83122392262697886 ) ) ;
#60712=CARTESIAN_POINT ( 'NONE',  ( 1.071796769724485232, 15.29240381056766651, 25.99999999999999645 ) ) ;
#60715=PRODUCT_CONTEXT ( 'NONE', #50292, 'mechanical' ) ;
#60720=CARTESIAN_POINT ( 'NONE',  ( -2.000000000000001776, 15.89374999877096784, 33.46410161513775705 ) ) ;
#60746=CARTESIAN_POINT ( 'NONE',  ( -1.999999999999999112, 14.39374999877096606, 26.53589838486224650 ) ) ;
#60747=ADVANCED_FACE ( 'NONE', ( #46313 ), #63649, .T. ) ;
#60763=ORIENTED_EDGE ( 'NONE', *, *, #3608, .T. ) ;
#60794=LINE ( 'NONE', #71157, #32460 ) ;
#60834=EDGE_CURVE ( 'NONE', #65514, #18562, #20101, .T. ) ;
#60839=CARTESIAN_POINT ( 'NONE',  ( 3.756430356249998770, 14.40312499938548463, 32.16877607737302469 ) ) ;
#60847=CARTESIAN_POINT ( 'NONE',  ( 1.878215178124997609, 13.12812499938548427, 33.25316411605952993 ) ) ;
#60877=CARTESIAN_POINT ( 'NONE',  ( -3.756430356249999214, 14.17812499938548498, 27.83122392262697531 ) ) ;
#60879=CARTESIAN_POINT ( 'NONE',  ( -1.999999999999999112, 17.14999999999999858, 26.53589838486224650 ) ) ;
#60880=CARTESIAN_POINT ( 'NONE',  ( -4.000000000000000000, 17.22500000000000142, 30.00000000000000000 ) ) ;
#60912=ORIENTED_EDGE ( 'NONE', *, *, #69480, .F. ) ;
#60913=VERTEX_POINT ( 'NONE', #17496 ) ;
#60965=CARTESIAN_POINT ( 'NONE',  ( 3.756430356249998770, 16.31562499938548427, 32.16877607737302469 ) ) ;
#60979=ORIENTED_EDGE ( 'NONE', *, *, #5722, .F. ) ;
#61008=CARTESIAN_POINT ( 'NONE',  ( -1.878215178124999163, 17.85312499938548214, 26.74683588394047007 ) ) ;
#61021=EDGE_CURVE ( 'NONE', #54204, #49855, #17306, .T. ) ;
#61034=DIRECTION ( 'NONE',  ( 0.000000000000000000, 0.000000000000000000, -1.000000000000000000 ) ) ;
#61065=CARTESIAN_POINT ( 'NONE',  ( -3.756430356250000102, 15.56562499938548427, 30.00000000000000000 ) ) ;
#61071=CARTESIAN_POINT ( 'NONE',  ( -7.967954043666661671E-16, 20.17812499938548143, 34.33755215474603517 ) ) ;
#61080=CARTESIAN_POINT ( 'NONE',  ( 3.756430356250000102, 18.49062499938548143, 30.00000000000000000 ) ) ;
#61097=CARTESIAN_POINT ( 'NONE',  ( 4.000000000000000000, 15.14374999877096606, 30.00000000000000000 ) ) ;
#61100=CARTESIAN_POINT ( 'NONE',  ( -1.071796769724490339, 17.52634618820329848, 26.00000000000000000 ) ) ;
#61153=CARTESIAN_POINT ( 'NONE',  ( -1.626862140677534273E-15, 15.53749999999999964, 34.00000000000000000 ) ) ;
#61166=CARTESIAN_POINT ( 'NONE',  ( 4.000000000000000000, 17.39374999877096428, 30.00000000000000000 ) ) ;
#61212=CARTESIAN_POINT ( 'NONE',  ( -7.967954043666661671E-16, 13.87812499938548250, 34.33755215474603517 ) ) ;
#61221=CARTESIAN_POINT ( 'NONE',  ( -1.878215178125001827, 14.40312499938548463, 33.25316411605952283 ) ) ;
#61249=CARTESIAN_POINT ( 'NONE',  ( 3.756430356250000546, 15.82812499938548179, 27.83122392262697886 ) ) ;
#61251=CARTESIAN_POINT ( 'NONE',  ( 4.000000000000000000, 16.58750000000000213, 27.69059892324149530 ) ) ;
#61307=AXIS2_PLACEMENT_3D ( 'NONE', #41500, #32152, #32518 ) ;
#61329=CARTESIAN_POINT ( 'NONE',  ( 1.878215178125000495, 15.52812499938548285, 26.74683588394047007 ) ) ;
#61372=CARTESIAN_POINT ( 'NONE',  ( 3.756430356249998770, 18.11562499938547788, 32.16877607737302469 ) ) ;
#61397=CARTESIAN_POINT ( 'NONE',  ( -1.071796769724492115, 20.01740381056766438, 34.00000000000000000 ) ) ;
#61428=CARTESIAN_POINT ( 'NONE',  ( -1.878215178124999163, 15.04062499938548392, 26.74683588394047007 ) ) ;
#61430=CYLINDRICAL_SURFACE ( 'NONE', #796, 4.000000000000000000 ) ;
#61443=CARTESIAN_POINT ( 'NONE',  ( -3.756430356250001434, 19.20312499938548356, 32.16877607737301048 ) ) ;
#61458=CARTESIAN_POINT ( 'NONE',  ( -1.999999999999999112, 18.89374999877096784, 26.53589838486224650 ) ) ;
#61461=DIRECTION ( 'NONE',  ( 0.000000000000000000, 0.000000000000000000, -1.000000000000000000 ) ) ;
#61491=DIRECTION ( 'NONE',  ( -0.000000000000000000, -1.000000000000000000, -0.000000000000000000 ) ) ;
#61523=CARTESIAN_POINT ( 'NONE',  ( 1.071796769724500997, 17.30134618820330417, 33.99999999999999289 ) ) ;
#61574=CARTESIAN_POINT ( 'NONE',  ( 1.878215178124997609, 13.57812499938548356, 33.25316411605952993 ) ) ;
#61605=CARTESIAN_POINT ( 'NONE',  ( 3.756430356249998770, 14.40312499938548463, 32.16877607737302469 ) ) ;
#61608=CARTESIAN_POINT ( 'NONE',  ( 3.999999999999998668, 17.41250000000000142, 32.30940107675850470 ) ) ;
#61649=AXIS2_PLACEMENT_3D ( 'NONE', #17155, #39347, #28257 ) ;
#61650=CARTESIAN_POINT ( 'NONE',  ( -1.071796769724492115, 20.41115380933863221, 34.00000000000000000 ) ) ;
#61688=CARTESIAN_POINT ( 'NONE',  ( -1.878215178125001827, 16.20312499938548356, 33.25316411605952283 ) ) ;
#61698=CARTESIAN_POINT ( 'NONE',  ( 3.999999999999998668, 18.31250000000000000, 32.30940107675850470 ) ) ;
#61731=CARTESIAN_POINT ( 'NONE',  ( 1.878215178125000495, 16.42812499938548143, 26.74683588394047007 ) ) ;
#61748=( BOUNDED_CURVE ( )  B_SPLINE_CURVE ( 2, ( #19724, #42275, #48185, #30462, #64798, #2388, #53726, #53353, #2751 ),
 .UNSPECIFIED., .F., .F. ) 
 B_SPLINE_CURVE_WITH_KNOTS ( ( 3, 2, 2, 2, 3 ),
 ( 0.2916666666666666852, 0.2962962962962962798, 0.3055555555555555802, 0.3148148148148148251, 0.3194444444444444753 ),
 .UNSPECIFIED. ) 
 CURVE ( )  GEOMETRIC_REPRESENTATION_ITEM ( )  RATIONAL_B_SPLINE_CURVE ( ( 0.9330127018922194093, 0.9330127018922197424, 1.000000000000000000, 0.8660254037844387076, 1.000000000000000000, 0.8660254037844387076, 1.000000000000000000, 0.9330127018922189652, 0.9330127018922194093 ) ) 
 REPRESENTATION_ITEM ( '' )  );
#61775=CARTESIAN_POINT ( 'NONE',  ( 0.000000000000000000, 27.50000000000000000, 30.00000000000000000 ) ) ;
#61786=CARTESIAN_POINT ( 'NONE',  ( 3.756430356250000546, 14.47812499938548747, 27.83122392262697886 ) ) ;
#61803=CARTESIAN_POINT ( 'NONE',  ( 3.756430356250000546, 17.62812499938548427, 27.83122392262697886 ) ) ;
#61818=CARTESIAN_POINT ( 'NONE',  ( -3.999999999999999556, 18.03124999877096712, 27.69059892324149175 ) ) ;
#61862=VECTOR ( 'NONE', #32146, 1000.000000000000000 ) ;
#61889=CARTESIAN_POINT ( 'NONE',  ( 0.6945846161026939525, 20.50052346155192140, 33.93923243933046763 ) ) ;
#61906=SURFACE_STYLE_USAGE ( .BOTH. , #10941 ) ;
#61932=ADVANCED_FACE ( 'NONE', ( #63291 ), #13041, .T. ) ;
#61943=CARTESIAN_POINT ( 'NONE',  ( 3.756430356249998770, 14.51562499938548356, 32.16877607737301759 ) ) ;
#61973=CARTESIAN_POINT ( 'NONE',  ( 4.000000000000000000, 18.38749999999999929, 27.69059892324149530 ) ) ;
#62011=CARTESIAN_POINT ( 'NONE',  ( 0.000000000000000000, 27.50000000000000000, 30.00000000000000000 ) ) ;
#62061=CARTESIAN_POINT ( 'NONE',  ( 1.878215178124997609, 15.82812499938548356, 33.25316411605952993 ) ) ;
#62075=ORIENTED_EDGE ( 'NONE', *, *, #7791, .F. ) ;
#62103=CARTESIAN_POINT ( 'NONE',  ( 2.655984681222220721E-16, 16.91562499938548214, 25.66244784525396483 ) ) ;
#62113=VERTEX_POINT ( 'NONE', #70297 ) ;
#62158=CARTESIAN_POINT ( 'NONE',  ( 1.878215178125000495, 17.21562499938548285, 26.74683588394047007 ) ) ;
#62183=CARTESIAN_POINT ( 'NONE',  ( 2.393811435568372112E-14, 17.28124999877096712, 34.00000000000000000 ) ) ;
#62191=CARTESIAN_POINT ( 'NONE',  ( 2.828200636599751609E-16, 18.85624999877096641, 25.38119784648299415 ) ) ;
#62228=ORIENTED_EDGE ( 'NONE', *, *, #44171, .T. ) ;
#62279=CARTESIAN_POINT ( 'NONE',  ( 5.810221930991193690E-16, 17.50624999877096499, 26.00000000000000000 ) ) ;
#62309=CARTESIAN_POINT ( 'NONE',  ( 1.878215178124997609, 15.82812499938548356, 33.25316411605952993 ) ) ;
#62315=LINE ( 'NONE', #28334, #69047 ) ;
#62339=CARTESIAN_POINT ( 'NONE',  ( 4.000000000000000000, 17.03750000000000142, 27.69059892324149530 ) ) ;
#62382=CARTESIAN_POINT ( 'NONE',  ( 0.000000000000000000, 27.50000000000000000, 30.00000000000000000 ) ) ;
#62389=ADVANCED_FACE ( 'NONE', ( #21139 ), #48501, .T. ) ;
#62418=CARTESIAN_POINT ( 'NONE',  ( 3.756430356249998770, 15.41562499938548392, 32.16877607737302469 ) ) ;
#62445=ORIENTED_EDGE ( 'NONE', *, *, #2787, .F. ) ;
#62458=CARTESIAN_POINT ( 'NONE',  ( 3.756430356250000546, 18.19062499938548427, 27.83122392262697886 ) ) ;
#62468=( BOUNDED_CURVE ( )  B_SPLINE_CURVE ( 2, ( #59654, #42314, #15321, #70748, #65570, #36765, #9063, #26051, #3897 ),
 .UNSPECIFIED., .F., .F. ) 
 B_SPLINE_CURVE_WITH_KNOTS ( ( 3, 2, 2, 2, 3 ),
 ( 0.01388888888888888985, 0.01851851851851851749, 0.02777777777777777624, 0.03703703703703703498, 0.04166666666666667129 ),
 .UNSPECIFIED. ) 
 CURVE ( )  GEOMETRIC_REPRESENTATION_ITEM ( )  RATIONAL_B_SPLINE_CURVE ( ( 0.9330127018922194093, 0.9330127018922194093, 1.000000000000000000, 0.8660254037844387076, 1.000000000000000000, 0.8660254037844387076, 1.000000000000000000, 0.9330127018922191873, 0.9330127018922192983 ) ) 
 REPRESENTATION_ITEM ( '' )  );
#62496=CARTESIAN_POINT ( 'NONE',  ( -1.626862140677534273E-15, 15.93124999877096748, 34.00000000000000000 ) ) ;
#62510=CYLINDRICAL_SURFACE ( 'NONE', #22993, 4.000000000000000000 ) ;
#62512=CARTESIAN_POINT ( 'NONE',  ( -7.967954043666661671E-16, 16.57812499938548356, 34.33755215474603517 ) ) ;
#62544=CARTESIAN_POINT ( 'NONE',  ( -2.000000000000001776, 18.59374999877096357, 33.46410161513775705 ) ) ;
#62573=CARTESIAN_POINT ( 'NONE',  ( 1.071796769724488785, 14.65759618943233455, 34.00000000000000000 ) ) ;
#62578=CARTESIAN_POINT ( 'NONE',  ( 3.999999999999998668, 16.51249999999999929, 32.30940107675850470 ) ) ;
#62630=( NAMED_UNIT ( * ) SI_UNIT ( $, .STERADIAN. ) SOLID_ANGLE_UNIT ( ) );
#62654=AXIS2_PLACEMENT_3D ( 'NONE', #13605, #69420, #35062 ) ;
#62663=ADVANCED_FACE ( 'NONE', ( #20262, #20629 ), #30628, .T. ) ;
#62668=CARTESIAN_POINT ( 'NONE',  ( -1.878215178124999163, 13.80312499938548321, 26.74683588394047007 ) ) ;
#62674=( GEOMETRIC_REPRESENTATION_CONTEXT ( 3 ) GLOBAL_UNCERTAINTY_ASSIGNED_CONTEXT ( ( #7773 ) ) GLOBAL_UNIT_ASSIGNED_CONTEXT ( ( #51324, #67243, #39518 ) ) REPRESENTATION_CONTEXT ( 'NONE', 'WORKASPACE' ) );
#62700=CARTESIAN_POINT ( 'NONE',  ( -4.000000000000000000, 20.37500000000000000, 30.00000000000000000 ) ) ;
#62737=CARTESIAN_POINT ( 'NONE',  ( 5.810221930991193690E-16, 18.40624999877096357, 26.00000000000000000 ) ) ;
#62780=CARTESIAN_POINT ( 'NONE',  ( -3.756430356250001434, 17.96562499938548285, 32.16877607737301048 ) ) ;
#62782=CARTESIAN_POINT ( 'NONE',  ( -8.484601909799255319E-16, 13.28749999999999964, 34.61880215351700940 ) ) ;
#62789=CARTESIAN_POINT ( 'NONE',  ( -3.999999999999999112, 16.28750000000000142, 27.69059892324149530 ) ) ;
#62819=CARTESIAN_POINT ( 'NONE',  ( 3.756430356249998770, 19.91562499938548214, 32.16877607737302469 ) ) ;
#62835=EDGE_CURVE ( 'NONE', #13067, #47310, #15094, .T. ) ;
#62859=CARTESIAN_POINT ( 'NONE',  ( -1.626862140677534273E-15, 15.53750000000000142, 34.00000000000000000 ) ) ;
#62871=CARTESIAN_POINT ( 'NONE',  ( -1.878215178124999163, 16.84062499938548285, 26.74683588394047007 ) ) ;
#62901=CARTESIAN_POINT ( 'NONE',  ( 1.999999999999997335, 19.56874999877096499, 33.46410161513775705 ) ) ;
#62934=CARTESIAN_POINT ( 'NONE',  ( 1.071796769724479237, 16.64240381056766438, 25.99999999999999645 ) ) ;
#62961=CARTESIAN_POINT ( 'NONE',  ( 1.878215178125000495, 14.96562499938548463, 26.74683588394047007 ) ) ;
#62985=SURFACE_STYLE_FILL_AREA ( #40470 ) ;
#62989=CARTESIAN_POINT ( 'NONE',  ( 2.000000000000000444, 12.57500000000000107, 26.53589838486224650 ) ) ;
#62992=CARTESIAN_POINT ( 'NONE',  ( 1.071796769724479237, 19.28615380933863221, 25.99999999999999645 ) ) ;
#63023=CARTESIAN_POINT ( 'NONE',  ( -3.756430356250000990, 16.16562499938548569, 32.16877607737301048 ) ) ;
#63027=CARTESIAN_POINT ( 'NONE',  ( -5.000000000000000000, 39.99999999999999289, 15.00000000000000178 ) ) ;
#63055=CARTESIAN_POINT ( 'NONE',  ( 4.000000000000000000, 19.73749999999999716, 27.69059892324149530 ) ) ;
#63106=CARTESIAN_POINT ( 'NONE',  ( 4.000000000000000000, 17.93750000000000355, 27.69059892324149885 ) ) ;
#63141=CARTESIAN_POINT ( 'NONE',  ( -1.878215178124999163, 18.30312499938548143, 26.74683588394047007 ) ) ;
#63143=CARTESIAN_POINT ( 'NONE',  ( -3.756430356249999214, 20.02812499938548285, 27.83122392262697531 ) ) ;
#63147=CARTESIAN_POINT ( 'NONE',  ( 0.000000000000000000, 25.54316770519903557, 26.00000000000000000 ) ) ;
#63150=LINE ( 'NONE', #12545, #36023 ) ;
#63188=ORIENTED_EDGE ( 'NONE', *, *, #70897, .T. ) ;
#63218=ORIENTED_EDGE ( 'NONE', *, *, #458, .F. ) ;
#63236=CARTESIAN_POINT ( 'NONE',  ( 2.655984681222220721E-16, 16.80312499938548498, 25.66244784525396483 ) ) ;
#63266=CARTESIAN_POINT ( 'NONE',  ( 3.756430356249998770, 13.61562499938548498, 32.16877607737302469 ) ) ;
#63290=CARTESIAN_POINT ( 'NONE',  ( -1.071796769724491671, 13.08259618943233704, 26.00000000000000355 ) ) ;
#63291=FACE_OUTER_BOUND ( 'NONE', #35592, .T. ) ;
#63330=CARTESIAN_POINT ( 'NONE',  ( 1.878215178124997609, 17.51562499938548356, 33.25316411605952993 ) ) ;
#63359=CARTESIAN_POINT ( 'NONE',  ( -1.999999999999999112, 13.04374999877096641, 26.53589838486224650 ) ) ;
#63392=CARTESIAN_POINT ( 'NONE',  ( -3.756430356250000102, 16.57812499938548356, 30.00000000000000000 ) ) ;
#63424=CARTESIAN_POINT ( 'NONE',  ( 0.6945846161026939525, 20.50052346155192851, 33.93923243933046763 ) ) ;
#63463=CARTESIAN_POINT ( 'NONE',  ( 4.000000000000000000, 15.63124999877096499, 27.69059892324149885 ) ) ;
#63479=EDGE_CURVE ( 'NONE', #47310, #67390, #57005, .T. ) ;
#63488=CARTESIAN_POINT ( 'NONE',  ( 4.000109024101403676, 24.99997092690864520, 30.26059014310604312 ) ) ;
#63506=CARTESIAN_POINT ( 'NONE',  ( -1.878215178124999163, 19.20312499938548356, 26.74683588394047007 ) ) ;
#63508=CARTESIAN_POINT ( 'NONE',  ( -2.000000000000001776, 13.70000000000000107, 33.46410161513775705 ) ) ;
#63535=( BOUNDED_CURVE ( )  B_SPLINE_CURVE ( 2, ( #45160, #102, #28173, #18504, #11535, #1183, #29607, #6351, #62496 ),
 .UNSPECIFIED., .F., .F. ) 
 B_SPLINE_CURVE_WITH_KNOTS ( ( 3, 2, 2, 2, 3 ),
 ( 0.3472222222222222654, 0.3518518518518518601, 0.3611111111111111049, 0.3703703703703703498, 0.3750000000000000000 ),
 .UNSPECIFIED. ) 
 CURVE ( )  GEOMETRIC_REPRESENTATION_ITEM ( )  RATIONAL_B_SPLINE_CURVE ( ( 0.9330127018922194093, 0.9330127018922197424, 1.000000000000000000, 0.8660254037844387076, 1.000000000000000000, 0.8660254037844387076, 1.000000000000000000, 0.9330127018922194093, 0.9330127018922194093 ) ) 
 REPRESENTATION_ITEM ( '' )  );
#63545=CARTESIAN_POINT ( 'NONE',  ( -3.756430356250001434, 20.66562499938548569, 32.16877607737301048 ) ) ;
#63598=CARTESIAN_POINT ( 'NONE',  ( 3.756430356250000102, 18.04062499938548214, 30.00000000000000000 ) ) ;
#63625=CARTESIAN_POINT ( 'NONE',  ( -1.999999999999999112, 20.24374999877096570, 26.53589838486224650 ) ) ;
#63649=CYLINDRICAL_SURFACE ( 'NONE', #37118, 4.000000000000000000 ) ;
#63686=CARTESIAN_POINT ( 'NONE',  ( -3.756430356250001434, 16.50312499938548783, 32.16877607737301048 ) ) ;
#63709=CARTESIAN_POINT ( 'NONE',  ( 4.000000000000000000, 14.73124999877096819, 27.69059892324149530 ) ) ;
#63744=CARTESIAN_POINT ( 'NONE',  ( 3.756430356249998770, 18.11562499938548143, 32.16877607737301759 ) ) ;
#63778=CARTESIAN_POINT ( 'NONE',  ( 2.828200636599751609E-16, 18.91249999999999787, 25.38119784648299415 ) ) ;
#63796=CARTESIAN_POINT ( 'NONE',  ( 0.000000000000000000, 27.50000000000000000, 26.00000000000000000 ) ) ;
#63800=CARTESIAN_POINT ( 'NONE',  ( 4.898587196589412829E-16, 27.50000000000000000, 34.00000000000000000 ) ) ;
#63825=DIRECTION ( 'NONE',  ( 0.000000000000000000, 0.000000000000000000, -1.000000000000000000 ) ) ;
#63842=CARTESIAN_POINT ( 'NONE',  ( 2.007161504316465894, 25.40607256557218108, 26.53021119236196412 ) ) ;
#63858=CARTESIAN_POINT ( 'NONE',  ( 1.878215178125000495, 17.32812499938548356, 26.74683588394047007 ) ) ;
#63860=CARTESIAN_POINT ( 'NONE',  ( 2.655984681222220721E-16, 20.40312499938548285, 25.66244784525396483 ) ) ;
#63871=ORIENTED_EDGE ( 'NONE', *, *, #24336, .F. ) ;
#63898=CARTESIAN_POINT ( 'NONE',  ( 0.6522905807966048464, 20.75364847883808395, 33.69936292076899065 ) ) ;
#63929=CARTESIAN_POINT ( 'NONE',  ( 1.071796769724479237, 20.63615380933863364, 25.99999999999999645 ) ) ;
#63959=CARTESIAN_POINT ( 'NONE',  ( 3.756430356249998770, 19.35312499938548214, 32.16877607737301759 ) ) ;
#63988=CARTESIAN_POINT ( 'NONE',  ( 3.756430356250000102, 12.75312499938548427, 30.00000000000000000 ) ) ;
#64040=ORIENTED_EDGE ( 'NONE', *, *, #35090, .F. ) ;
#64049=CARTESIAN_POINT ( 'NONE',  ( 2.655984681222220721E-16, 16.80312499938548143, 25.66244784525396483 ) ) ;
#64101=( BOUNDED_CURVE ( )  B_SPLINE_CURVE ( 2, ( #18987, #37090, #35633, #65164, #41195, #41549, #13095, #58154, #7559 ),
 .UNSPECIFIED., .F., .F. ) 
 B_SPLINE_CURVE_WITH_KNOTS ( ( 3, 2, 2, 2, 3 ),
 ( 0.5972222222222222099, 0.6018518518518518601, 0.6111111111111111605, 0.6203703703703703498, 0.6250000000000000000 ),
 .UNSPECIFIED. ) 
 CURVE ( )  GEOMETRIC_REPRESENTATION_ITEM ( )  RATIONAL_B_SPLINE_CURVE ( ( 0.9330127018922194093, 0.9330127018922194093, 1.000000000000000000, 0.8660254037844387076, 1.000000000000000000, 0.8660254037844387076, 1.000000000000000000, 0.9330127018922194093, 0.9330127018922194093 ) ) 
 REPRESENTATION_ITEM ( '' )  );
#64105=CARTESIAN_POINT ( 'NONE',  ( -3.756430356249999214, 16.99062499938548498, 27.83122392262697176 ) ) ;
#64116=CARTESIAN_POINT ( 'NONE',  ( 4.898587196589412829E-16, 27.50000000000000000, 34.00000000000000000 ) ) ;
#64141=CARTESIAN_POINT ( 'NONE',  ( -8.484601909799255319E-16, 18.68750000000000000, 34.61880215351700940 ) ) ;
#64171=ADVANCED_FACE ( 'NONE', ( #20541 ), #66736, .F. ) ;
#64176=AXIS2_PLACEMENT_3D ( 'NONE', #22688, #66312, #15689 ) ;
#64180=CARTESIAN_POINT ( 'NONE',  ( 3.999999999999998668, 18.25624999877096855, 32.30940107675850470 ) ) ;
#64207=CARTESIAN_POINT ( 'NONE',  ( 3.999999999999998668, 13.36250000000000071, 32.30940107675850470 ) ) ;
#64224=CARTESIAN_POINT ( 'NONE',  ( -3.756430356250000102, 13.76562499938548356, 30.00000000000000000 ) ) ;
#64226=CARTESIAN_POINT ( 'NONE',  ( 4.000000000000000000, 12.95000000000000107, 30.00000000000000000 ) ) ;
#64267=CARTESIAN_POINT ( 'NONE',  ( -3.756430356249999214, 18.79062499938548214, 27.83122392262697531 ) ) ;
#64277=ORIENTED_EDGE ( 'NONE', *, *, #66154, .T. ) ;
#64322=CARTESIAN_POINT ( 'NONE',  ( -1.878215178125001827, 20.59062499938548285, 33.25316411605952283 ) ) ;
#64338=CARTESIAN_POINT ( 'NONE',  ( -1.071796769724492115, 15.51740381056766438, 34.00000000000000000 ) ) ;
#64352=ORIENTED_EDGE ( 'NONE', *, *, #66154, .F. ) ;
#64356=CARTESIAN_POINT ( 'NONE',  ( -3.756430356250000102, 12.97812499938548214, 30.00000000000000000 ) ) ;
#64386=ADVANCED_FACE ( 'NONE', ( #56372 ), #45288, .T. ) ;
#64411=CARTESIAN_POINT ( 'NONE',  ( -3.756430356250000990, 12.90312499938548463, 32.16877607737301048 ) ) ;
#64417=CARTESIAN_POINT ( 'NONE',  ( 3.756430356250000546, 17.17812499938548143, 27.83122392262697886 ) ) ;
#64427=CARTESIAN_POINT ( 'NONE',  ( -3.756430356249999214, 15.52812499938548108, 27.83122392262697531 ) ) ;
#64441=CARTESIAN_POINT ( 'NONE',  ( 3.999999999999998668, 14.20624999877096606, 32.30940107675850470 ) ) ;
#64473=CARTESIAN_POINT ( 'NONE',  ( 1.878215178125000495, 17.77812499938548285, 26.74683588394047007 ) ) ;
#64474=CARTESIAN_POINT ( 'NONE',  ( -3.999999999999999112, 14.48750000000000071, 27.69059892324149530 ) ) ;
#64503=DIRECTION ( 'NONE',  ( -0.000000000000000000, -1.000000000000000000, -0.000000000000000000 ) ) ;
#64514=CARTESIAN_POINT ( 'NONE',  ( -2.000000000000001776, 19.49374999877096570, 33.46410161513775705 ) ) ;
#64567=CARTESIAN_POINT ( 'NONE',  ( 0.000000000000000000, 27.50000000000000000, 26.00000000000000000 ) ) ;
#64578=CARTESIAN_POINT ( 'NONE',  ( 2.441552069295954475, 25.34000229536805548, 33.17907134633756527 ) ) ;
#64595=CARTESIAN_POINT ( 'NONE',  ( -3.756430356250000102, 19.72812499938548214, 30.00000000000000000 ) ) ;
#64597=CARTESIAN_POINT ( 'NONE',  ( 4.000000000000000000, 15.68750000000000000, 27.69059892324149530 ) ) ;
#64634=ORIENTED_EDGE ( 'NONE', *, *, #21313, .F. ) ;
#64641=AXIS2_PLACEMENT_3D ( 'NONE', #56613, #6369, #34073 ) ;
#64676=CARTESIAN_POINT ( 'NONE',  ( -2.646227255512634713, 25.30407769034638576, 26.98922086287628019 ) ) ;
#64679=CARTESIAN_POINT ( 'NONE',  ( -1.243387493232115393E-14, 15.76249999999999929, 26.00000000000000000 ) ) ;
#64692=CARTESIAN_POINT ( 'NONE',  ( 3.756430356250000102, 18.94062499938548427, 30.00000000000000000 ) ) ;
#64722=CARTESIAN_POINT ( 'NONE',  ( -3.756430356249999214, 12.94062499938548250, 27.83122392262697531 ) ) ;
#64782=CARTESIAN_POINT ( 'NONE',  ( 1.878215178125000495, 16.76562499938548356, 26.74683588394047007 ) ) ;
#64791=CARTESIAN_POINT ( 'NONE',  ( 1.878215178125000495, 14.96562499938548463, 26.74683588394047007 ) ) ;
#64798=CARTESIAN_POINT ( 'NONE',  ( -4.000000000000000000, 14.97499999999999964, 30.00000000000000000 ) ) ;
#64807=CARTESIAN_POINT ( 'NONE',  ( 4.000000000000000000, 13.83124999877096606, 27.69059892324149530 ) ) ;
#64811=ORIENTED_EDGE ( 'NONE', *, *, #64818, .F. ) ;
#64818=EDGE_CURVE ( 'NONE', #49631, #13067, #44305, .T. ) ;
#64830=EDGE_CURVE ( 'NONE', #31816, #70824, #64101, .T. ) ;
#64840=DIRECTION ( 'NONE',  ( 0.000000000000000000, 0.000000000000000000, -1.000000000000000000 ) ) ;
#64843=CARTESIAN_POINT ( 'NONE',  ( 1.878215178124997609, 20.32812499938548356, 33.25316411605952993 ) ) ;
#64844=CYLINDRICAL_SURFACE ( 'NONE', #12597, 4.000000000000000000 ) ;
#64847=ORIENTED_EDGE ( 'NONE', *, *, #12973, .T. ) ;
#64855=VERTEX_POINT ( 'NONE', #9028 ) ;
#64858=ORIENTED_EDGE ( 'NONE', *, *, #5878, .T. ) ;
#64961=CARTESIAN_POINT ( 'NONE',  ( -3.756430356249999214, 13.72812499938548392, 27.83122392262697531 ) ) ;
#64963=CARTESIAN_POINT ( 'NONE',  ( 3.999999999999998668, 14.71250000000000036, 32.30940107675850470 ) ) ;
#65029=CARTESIAN_POINT ( 'NONE',  ( 4.000000000000000000, 20.58124999877096784, 27.69059892324149885 ) ) ;
#65041=EDGE_CURVE ( 'NONE', #16672, #4034, #61748, .T. ) ;
#65044=CARTESIAN_POINT ( 'NONE',  ( 1.878215178124997609, 13.57812499938548356, 33.25316411605952993 ) ) ;
#65055=CARTESIAN_POINT ( 'NONE',  ( 3.756430356250000102, 19.84062499938548640, 30.00000000000000000 ) ) ;
#65071=( GEOMETRIC_REPRESENTATION_CONTEXT ( 3 ) GLOBAL_UNCERTAINTY_ASSIGNED_CONTEXT ( ( #52118 ) ) GLOBAL_UNIT_ASSIGNED_CONTEXT ( ( #22740, #39758, #51192 ) ) REPRESENTATION_CONTEXT ( 'NONE', 'WORKASPACE' ) );
#65086=CARTESIAN_POINT ( 'NONE',  ( 3.756430356250000546, 15.49062499938548321, 27.83122392262697886 ) ) ;
#65132=EDGE_LOOP ( 'NONE', ( #47385, #42851, #22337, #7899 ) ) ;
#65140=CARTESIAN_POINT ( 'NONE',  ( -3.756430356249999214, 13.27812499938548285, 27.83122392262697176 ) ) ;
#65147=CARTESIAN_POINT ( 'NONE',  ( 3.756430356250000102, 19.84062499938548640, 30.00000000000000000 ) ) ;
#65156=CARTESIAN_POINT ( 'NONE',  ( 3.756430356250000102, 15.79062499938548392, 30.00000000000000000 ) ) ;
#65164=CARTESIAN_POINT ( 'NONE',  ( 3.999999999999998668, 17.41250000000000142, 32.30940107675850470 ) ) ;
#65172=CARTESIAN_POINT ( 'NONE',  ( 1.999999999999997335, 16.86874999877096570, 33.46410161513775705 ) ) ;
#65184=EDGE_CURVE ( 'NONE', #4034, #62113, #41478, .T. ) ;
#65204=CARTESIAN_POINT ( 'NONE',  ( 3.756430356250000546, 19.99062499938547788, 27.83122392262697886 ) ) ;
#65217=ORIENTED_EDGE ( 'NONE', *, *, #5701, .F. ) ;
#65291=CARTESIAN_POINT ( 'NONE',  ( -1.071796769724480347, 18.61115380933862795, 34.00000000000000711 ) ) ;
#65294=CARTESIAN_POINT ( 'NONE',  ( -3.756430356250000102, 12.97812499938548214, 30.00000000000000000 ) ) ;
#65295=CARTESIAN_POINT ( 'NONE',  ( -2.672702088255949472E-15, 13.90624999877096890, 26.00000000000000000 ) ) ;
#65322=CARTESIAN_POINT ( 'NONE',  ( -1.878215178125001827, 19.80312499938548143, 33.25316411605952283 ) ) ;
#65324=CARTESIAN_POINT ( 'NONE',  ( -1.999999999999999112, 14.45000000000000107, 26.53589838486224650 ) ) ;
#65404=CARTESIAN_POINT ( 'NONE',  ( -1.292810628673454865, 25.48745481703416971, 33.79429592041256569 ) ) ;
#65408=CARTESIAN_POINT ( 'NONE',  ( -3.756430356250001434, 13.46562499938548285, 32.16877607737301048 ) ) ;
#65420=CARTESIAN_POINT ( 'NONE',  ( -1.878215178125001827, 18.79062499938548214, 33.25316411605952283 ) ) ;
#65451=CARTESIAN_POINT ( 'NONE',  ( 2.655984681222220721E-16, 15.11562499938548321, 25.66244784525396483 ) ) ;
#65466=AXIS2_PLACEMENT_3D ( 'NONE', #7063, #35492, #41054 ) ;
#65478=CARTESIAN_POINT ( 'NONE',  ( 1.999999999999997335, 20.07499999999999929, 33.46410161513775705 ) ) ;
#65499=CARTESIAN_POINT ( 'NONE',  ( -1.071796769724490339, 19.77634618820329848, 26.00000000000000000 ) ) ;
#65511=CARTESIAN_POINT ( 'NONE',  ( 2.655984681222220721E-16, 13.20312499938548534, 25.66244784525396483 ) ) ;
#65514=VERTEX_POINT ( 'NONE', #67380 ) ;
#65519=CARTESIAN_POINT ( 'NONE',  ( 2.655984681222220721E-16, 19.05312499938548143, 25.66244784525396483 ) ) ;
#65528=CARTESIAN_POINT ( 'NONE',  ( 2.655984681222220721E-16, 16.35312499938548214, 25.66244784525396483 ) ) ;
#65536=CARTESIAN_POINT ( 'NONE',  ( 4.000000000000000000, 15.23750000000000071, 27.69059892324149885 ) ) ;
#65543=CARTESIAN_POINT ( 'NONE',  ( -8.484601909799255319E-16, 15.93124999877096748, 34.61880215351700940 ) ) ;
#65570=CARTESIAN_POINT ( 'NONE',  ( -4.000000000000000000, 12.72499999999999964, 30.00000000000000000 ) ) ;
#65573=CARTESIAN_POINT ( 'NONE',  ( 3.756430356250000102, 20.40312499938548285, 30.00000000000000000 ) ) ;
#65583=CARTESIAN_POINT ( 'NONE',  ( -4.000000000000000888, 20.41250000000000142, 32.30940107675850470 ) ) ;
#65597=VECTOR ( 'NONE', #59746, 1000.000000000000000 ) ;
#65607=CARTESIAN_POINT ( 'NONE',  ( -4.000000000000000000, 14.91874999877096641, 30.00000000000000000 ) ) ;
#65613=DIRECTION ( 'NONE',  ( -0.000000000000000000, -1.000000000000000000, -0.000000000000000000 ) ) ;
#65628=CARTESIAN_POINT ( 'NONE',  ( -1.071796769724492115, 19.11740381056766225, 34.00000000000000000 ) ) ;
#65636=CYLINDRICAL_SURFACE ( 'NONE', #15986, 4.000000000000000000 ) ;
#65658=CARTESIAN_POINT ( 'NONE',  ( -1.626862140677534273E-15, 18.18124999877096215, 34.00000000000000000 ) ) ;
#65667=CARTESIAN_POINT ( 'NONE',  ( -1.999999999999999112, 16.69999999999999929, 26.53589838486224650 ) ) ;
#65693=CARTESIAN_POINT ( 'NONE',  ( -3.756430356249999214, 20.14062499938548356, 27.83122392262697531 ) ) ;
#65695=CARTESIAN_POINT ( 'NONE',  ( -4.000000000000000000, 14.52500000000000036, 30.00000000000000000 ) ) ;
#65715=CARTESIAN_POINT ( 'NONE',  ( -3.999999999999999112, 15.38750000000000107, 27.69059892324149530 ) ) ;
#65732=ORIENTED_EDGE ( 'NONE', *, *, #45894, .F. ) ;
#65771=CARTESIAN_POINT ( 'NONE',  ( -4.000000000000000888, 15.91249999999999964, 32.30940107675850470 ) ) ;
#65780=CARTESIAN_POINT ( 'NONE',  ( 1.999999999999997335, 15.57500000000000107, 33.46410161513775705 ) ) ;
#65823=CARTESIAN_POINT ( 'NONE',  ( -3.756430356250001434, 13.91562499938548392, 32.16877607737301048 ) ) ;
#65850=DIRECTION ( 'NONE',  ( -0.000000000000000000, -1.000000000000000000, -0.000000000000000000 ) ) ;
#65854=( BOUNDED_CURVE ( )  B_SPLINE_CURVE ( 2, ( #65295, #37957, #265, #38702, #10978, #44618, #17591, #51228, #16508 ),
 .UNSPECIFIED., .F., .F. ) 
 B_SPLINE_CURVE_WITH_KNOTS ( ( 3, 2, 2, 2, 3 ),
 ( 0.1250000000000000000, 0.1296296296296296224, 0.1388888888888888951, 0.1481481481481481399, 0.1527777777777777901 ),
 .UNSPECIFIED. ) 
 CURVE ( )  GEOMETRIC_REPRESENTATION_ITEM ( )  RATIONAL_B_SPLINE_CURVE ( ( 0.9330127018922192983, 0.9330127018922194093, 1.000000000000000000, 0.8660254037844387076, 1.000000000000000000, 0.8660254037844387076, 1.000000000000000000, 0.9330127018922191873, 0.9330127018922194093 ) ) 
 REPRESENTATION_ITEM ( '' )  );
#65868=EDGE_CURVE ( 'NONE', #32715, #51293, #56571, .T. ) ;
#65887=CARTESIAN_POINT ( 'NONE',  ( -3.756430356249999214, 18.67812499938548143, 27.83122392262697531 ) ) ;
#65897=CARTESIAN_POINT ( 'NONE',  ( 1.878215178125000495, 15.41562499938548392, 26.74683588394047007 ) ) ;
#65912=CARTESIAN_POINT ( 'NONE',  ( 1.999999999999997335, 15.51874999877096784, 33.46410161513775705 ) ) ;
#65921=CARTESIAN_POINT ( 'NONE',  ( -1.071796769724496334, 16.17634618820330061, 26.00000000000000355 ) ) ;
#65944=CARTESIAN_POINT ( 'NONE',  ( -3.756430356250000990, 18.86562499938548498, 32.16877607737301048 ) ) ;
#65945=CARTESIAN_POINT ( 'NONE',  ( -4.000000000000000000, 14.52500000000000036, 30.00000000000000000 ) ) ;
#65954=LINE ( 'NONE', #27170, #8874 ) ;
#66027=CARTESIAN_POINT ( 'NONE',  ( -7.967954043666661671E-16, 14.32812499938548179, 34.33755215474603517 ) ) ;
#66035=CYLINDRICAL_SURFACE ( 'NONE', #54313, 4.000000000000000000 ) ;
#66037=CARTESIAN_POINT ( 'NONE',  ( -3.999999999999999112, 16.73750000000000071, 27.69059892324149530 ) ) ;
#66060=CARTESIAN_POINT ( 'NONE',  ( -3.756430356249999214, 14.62812499938548250, 27.83122392262697531 ) ) ;
#66062=CARTESIAN_POINT ( 'NONE',  ( 2.828200636599751609E-16, 16.21250000000000213, 25.38119784648299415 ) ) ;
#66081=CARTESIAN_POINT ( 'NONE',  ( -1.999999999999999112, 15.35000000000000142, 26.53589838486224650 ) ) ;
#66137=CARTESIAN_POINT ( 'NONE',  ( -1.243387493232115393E-14, 15.76249999999999929, 26.00000000000000000 ) ) ;
#66146=CARTESIAN_POINT ( 'NONE',  ( -3.756430356249999214, 13.39062499938548179, 27.83122392262697531 ) ) ;
#66154=EDGE_CURVE ( 'NONE', #70620, #68959, #8452, .T. ) ;
#66189=CARTESIAN_POINT ( 'NONE',  ( -1.878215178125001827, 15.75312499938548427, 33.25316411605952283 ) ) ;
#66231=FACE_OUTER_BOUND ( 'NONE', #8200, .T. ) ;
#66234=ORIENTED_EDGE ( 'NONE', *, *, #19843, .F. ) ;
#66243=CARTESIAN_POINT ( 'NONE',  ( -7.967954043666661671E-16, 13.87812499938548250, 34.33755215474603517 ) ) ;
#66249=CARTESIAN_POINT ( 'NONE',  ( 2.655984681222220721E-16, 19.50312499938548427, 25.66244784525396483 ) ) ;
#66259=CARTESIAN_POINT ( 'NONE',  ( -3.756430356250001434, 18.30312499938548143, 32.16877607737301048 ) ) ;
#66276=CARTESIAN_POINT ( 'NONE',  ( 3.999999999999998668, 16.00624999877096499, 32.30940107675850470 ) ) ;
#66312=DIRECTION ( 'NONE',  ( -0.000000000000000000, -1.000000000000000000, -0.000000000000000000 ) ) ;
#66317=ORIENTED_EDGE ( 'NONE', *, *, #49986, .T. ) ;
#66342=CARTESIAN_POINT ( 'NONE',  ( 5.810221930991193690E-16, 17.56250000000000000, 26.00000000000000000 ) ) ;
#66393=CARTESIAN_POINT ( 'NONE',  ( 1.878215178124997609, 13.01562499938548356, 33.25316411605952993 ) ) ;
#66399=CARTESIAN_POINT ( 'NONE',  ( -1.071796769724490339, 18.42634618820330061, 26.00000000000000000 ) ) ;
#66403=CARTESIAN_POINT ( 'NONE',  ( 2.393811435568372112E-14, 16.88750000000000284, 34.00000000000000000 ) ) ;
#66412=EDGE_LOOP ( 'NONE', ( #20982, #56283, #41637, #27323 ) ) ;
#66430=CARTESIAN_POINT ( 'NONE',  ( -7.967954043666661671E-16, 15.67812499938548321, 34.33755215474603517 ) ) ;
#66432=CARTESIAN_POINT ( 'NONE',  ( -4.000000000000000000, 16.77499999999999858, 30.00000000000000000 ) ) ;
#66466=EDGE_LOOP ( 'NONE', ( #37293, #70548 ) ) ;
#66468=CYLINDRICAL_SURFACE ( 'NONE', #59772, 4.000000000000000000 ) ;
#66478=CARTESIAN_POINT ( 'NONE',  ( -1.071796769724490783, 13.21115380933863293, 34.00000000000000711 ) ) ;
#66512=CARTESIAN_POINT ( 'NONE',  ( -7.967954043666661671E-16, 16.69062499938548427, 34.33755215474603517 ) ) ;
#66534=CARTESIAN_POINT ( 'NONE',  ( -1.626862140677534273E-15, 19.58750000000000213, 34.00000000000000000 ) ) ;
#66552=ORIENTED_EDGE ( 'NONE', *, *, #41750, .F. ) ;
#66555=CARTESIAN_POINT ( 'NONE',  ( -3.756430356249999214, 14.29062499938548214, 27.83122392262697531 ) ) ;
#66586=LINE ( 'NONE', #21874, #72735 ) ;
#66611=EDGE_LOOP ( 'NONE', ( #44464, #920, #55020, #20464 ) ) ;
#66616=CARTESIAN_POINT ( 'NONE',  ( -3.756430356249999214, 15.07812499938548356, 27.83122392262697176 ) ) ;
#66618=DIRECTION ( 'NONE',  ( 0.000000000000000000, 0.000000000000000000, -1.000000000000000000 ) ) ;
#66619=ORIENTED_EDGE ( 'NONE', *, *, #12168, .T. ) ;
#66622=CARTESIAN_POINT ( 'NONE',  ( 1.878215178125000495, 20.36562499938548143, 26.74683588394047007 ) ) ;
#66631=CARTESIAN_POINT ( 'NONE',  ( 1.878215178125000495, 17.66562499938548214, 26.74683588394047007 ) ) ;
#66641=CARTESIAN_POINT ( 'NONE',  ( 4.000000000000000000, 15.19999999999999929, 30.00000000000000000 ) ) ;
#66648=CARTESIAN_POINT ( 'NONE',  ( 2.000000000000000444, 17.01874999877096428, 26.53589838486224650 ) ) ;
#66736=PLANE ( 'NONE',  #34799 ) ;
#66768=CARTESIAN_POINT ( 'NONE',  ( -1.878215178125001827, 14.29062499938548392, 33.25316411605952283 ) ) ;
#66773=EDGE_CURVE ( 'NONE', #71220, #60301, #71393, .T. ) ;
#66777=CARTESIAN_POINT ( 'NONE',  ( -7.967954043666661671E-16, 14.89062499938548179, 34.33755215474603517 ) ) ;
#66778=CARTESIAN_POINT ( 'NONE',  ( -4.000000000000000888, 15.40624999877096535, 32.30940107675850470 ) ) ;
#66797=CARTESIAN_POINT ( 'NONE',  ( 4.000000000000000000, 19.70000000000000284, 30.00000000000000000 ) ) ;
#66806=CARTESIAN_POINT ( 'NONE',  ( 3.756430356250000546, 14.92812499938548321, 27.83122392262697886 ) ) ;
#66808=CARTESIAN_POINT ( 'NONE',  ( 4.000000000000000000, 17.00000000000000000, 30.00000000000000000 ) ) ;
#66826=CARTESIAN_POINT ( 'NONE',  ( -1.626862140677534273E-15, 19.98124999877096641, 34.00000000000000000 ) ) ;
#66887=CARTESIAN_POINT ( 'NONE',  ( 0.000000000000000000, 12.50000000000000000, 30.00000000000000000 ) ) ;
#66891=CARTESIAN_POINT ( 'NONE',  ( -3.756430356250001434, 15.71562499938548108, 32.16877607737301048 ) ) ;
#66900=CARTESIAN_POINT ( 'NONE',  ( 2.417052323292336544E-14, 20.48749999999999716, 34.00000000000000000 ) ) ;
#66934=CARTESIAN_POINT ( 'NONE',  ( 3.756430356250000546, 18.64062499938548001, 27.83122392262697886 ) ) ;
#66939=VECTOR ( 'NONE', #13190, 1000.000000000000000 ) ;
#66959=CARTESIAN_POINT ( 'NONE',  ( -2.000000000000001776, 13.64374999877096784, 33.46410161513775705 ) ) ;
#66987=ORIENTED_EDGE ( 'NONE', *, *, #42756, .F. ) ;
#66992=CARTESIAN_POINT ( 'NONE',  ( -3.756430356250000990, 15.15312499938548463, 32.16877607737301048 ) ) ;
#67008=CARTESIAN_POINT ( 'NONE',  ( -7.967954043666661671E-16, 17.92812499938548498, 34.33755215474603517 ) ) ;
#67025=CARTESIAN_POINT ( 'NONE',  ( 2.000000000000000444, 18.81874999877096499, 26.53589838486224650 ) ) ;
#67028=CARTESIAN_POINT ( 'NONE',  ( 3.999999999999998668, 12.91249999999999964, 32.30940107675850470 ) ) ;
#67048=EDGE_CURVE ( 'NONE', #45011, #71132, #43864, .T. ) ;
#67086=ORIENTED_EDGE ( 'NONE', *, *, #47391, .T. ) ;
#67092=CARTESIAN_POINT ( 'NONE',  ( 1.999999999999997335, 17.31874999877096499, 33.46410161513775705 ) ) ;
#67139=CARTESIAN_POINT ( 'NONE',  ( -3.756430356249999214, 13.72812499938548392, 27.83122392262697531 ) ) ;
#67147=CARTESIAN_POINT ( 'NONE',  ( -3.756430356250000102, 14.77812499938548463, 30.00000000000000000 ) ) ;
#67150=CARTESIAN_POINT ( 'NONE',  ( 2.393811435568372112E-14, 16.88750000000000284, 34.00000000000000000 ) ) ;
#67156=EDGE_LOOP ( 'NONE', ( #16289, #45158, #28888, #60027 ) ) ;
#67174=CARTESIAN_POINT ( 'NONE',  ( -1.878215178125001827, 16.09062499938548285, 33.25316411605952283 ) ) ;
#67177=CARTESIAN_POINT ( 'NONE',  ( -1.999999999999999112, 18.05000000000000071, 26.53589838486224650 ) ) ;
#67190=ORIENTED_EDGE ( 'NONE', *, *, #43763, .T. ) ;
#67243=( NAMED_UNIT ( * ) PLANE_ANGLE_UNIT ( ) SI_UNIT ( $, .RADIAN. ) );
#67255=DIRECTION ( 'NONE',  ( -0.000000000000000000, -1.000000000000000000, -0.000000000000000000 ) ) ;
#67259=CARTESIAN_POINT ( 'NONE',  ( -1.878215178124999163, 15.15312499938548285, 26.74683588394047007 ) ) ;
#67269=CARTESIAN_POINT ( 'NONE',  ( 1.071796769724500997, 18.25759618943233065, 33.99999999999999289 ) ) ;
#67303=CARTESIAN_POINT ( 'NONE',  ( 3.756430356250000102, 17.70312499938548356, 30.00000000000000000 ) ) ;
#67356=CARTESIAN_POINT ( 'NONE',  ( -7.967954043666661671E-16, 15.22812499938548392, 34.33755215474603517 ) ) ;
#67371=CARTESIAN_POINT ( 'NONE',  ( -3.756430356250000102, 19.61562499938548143, 30.00000000000000000 ) ) ;
#67380=CARTESIAN_POINT ( 'NONE',  ( -2.672702088255949472E-15, 13.06250000000000355, 26.00000000000000000 ) ) ;
#67386=CARTESIAN_POINT ( 'NONE',  ( -1.999999999999999112, 18.44374999877096499, 26.53589838486224650 ) ) ;
#67389=CARTESIAN_POINT ( 'NONE',  ( 4.000000000000000000, 12.98749999999999893, 27.69059892324149885 ) ) ;
#67390=VERTEX_POINT ( 'NONE', #11597 ) ;
#67397=CARTESIAN_POINT ( 'NONE',  ( 5.810221930991193690E-16, 14.41249999999999787, 26.00000000000000000 ) ) ;
#67418=CARTESIAN_POINT ( 'NONE',  ( -2.498395430326213790E-14, 20.65624999877097068, 26.00000000000000000 ) ) ;
#67424=VERTEX_POINT ( 'NONE', #67397 ) ;
#67429=( BOUNDED_CURVE ( )  B_SPLINE_CURVE ( 2, ( #9525, #54591, #65667, #66037, #26520, #49418, #49786, #59751, #67150 ),
 .UNSPECIFIED., .F., .F. ) 
 B_SPLINE_CURVE_WITH_KNOTS ( ( 3, 2, 2, 2, 3 ),
 ( 0.5138888888888889506, 0.5185185185185184897, 0.5277777777777777901, 0.5370370370370370905, 0.5416666666666667407 ),
 .UNSPECIFIED. ) 
 CURVE ( )  GEOMETRIC_REPRESENTATION_ITEM ( )  RATIONAL_B_SPLINE_CURVE ( ( 0.9330127018922192983, 0.9330127018922200755, 1.000000000000000000, 0.8660254037844387076, 1.000000000000000000, 0.8660254037844387076, 1.000000000000000000, 0.9330127018922185211, 0.9330127018922192983 ) ) 
 REPRESENTATION_ITEM ( '' )  );
#67441=ADVANCED_FACE ( 'NONE', ( #51119 ), #40041, .T. ) ;
#67454=CARTESIAN_POINT ( 'NONE',  ( 0.3499497844256071466, 20.88781155722894312, 33.99999999999999289 ) ) ;
#67503=CARTESIAN_POINT ( 'NONE',  ( 3.756430356250000546, 14.14062499938548356, 27.83122392262697886 ) ) ;
#67534=CARTESIAN_POINT ( 'NONE',  ( 4.000000000000000000, 17.93750000000000355, 27.69059892324149530 ) ) ;
#67586=EDGE_CURVE ( 'NONE', #59214, #3561, #26810, .T. ) ;
#67613=CARTESIAN_POINT ( 'NONE',  ( 2.655984681222220721E-16, 16.91562499938548214, 25.66244784525396483 ) ) ;
#67622=CARTESIAN_POINT ( 'NONE',  ( -1.071796769724492115, 16.41740381056766651, 34.00000000000000000 ) ) ;
#67655=CARTESIAN_POINT ( 'NONE',  ( 3.756430356250000102, 16.80312499938548498, 30.00000000000000000 ) ) ;
#67707=CARTESIAN_POINT ( 'NONE',  ( 3.756430356250000546, 14.02812499938548285, 27.83122392262697886 ) ) ;
#67723=CARTESIAN_POINT ( 'NONE',  ( -3.756430356249999214, 19.12812499938548427, 27.83122392262697531 ) ) ;
#67739=CARTESIAN_POINT ( 'NONE',  ( -4.000000000000000000, 17.61874999877096570, 30.00000000000000000 ) ) ;
#67742=CARTESIAN_POINT ( 'NONE',  ( -4.000000000000000000, 17.61874999877096570, 30.00000000000000000 ) ) ;
#67771=CARTESIAN_POINT ( 'NONE',  ( -2.000000000000001776, 20.84374999877096357, 33.46410161513775705 ) ) ;
#67857=( BOUNDED_CURVE ( )  B_SPLINE_CURVE ( 2, ( #19953, #13684, #46592, #53584, #36590, #65029, #42506, #63929, #18493 ),
 .UNSPECIFIED., .F., .F. ) 
 B_SPLINE_CURVE_WITH_KNOTS ( ( 3, 2, 2, 2, 3 ),
 ( 0.9305555555555555802, 0.9351851851851852304, 0.9444444444444444198, 0.9537037037037037202, 0.9583333333333333703 ),
 .UNSPECIFIED. ) 
 CURVE ( )  GEOMETRIC_REPRESENTATION_ITEM ( )  RATIONAL_B_SPLINE_CURVE ( ( 0.9330127018922194093, 0.9330127018922194093, 1.000000000000000000, 0.8660254037844387076, 1.000000000000000000, 0.8660254037844387076, 1.000000000000000000, 0.9330127018922185211, 0.9330127018922192983 ) ) 
 REPRESENTATION_ITEM ( '' )  );
#67861=CARTESIAN_POINT ( 'NONE',  ( 2.655984681222220721E-16, 13.76562499938548534, 25.66244784525396483 ) ) ;
#67886=ORIENTED_EDGE ( 'NONE', *, *, #57999, .F. ) ;
#67891=CARTESIAN_POINT ( 'NONE',  ( 2.000000000000000444, 18.42500000000000071, 26.53589838486224650 ) ) ;
#67905=ORIENTED_EDGE ( 'NONE', *, *, #10225, .T. ) ;
#67935=CARTESIAN_POINT ( 'NONE',  ( -2.000000000000001776, 20.39374999877096428, 33.46410161513775705 ) ) ;
#67973=CARTESIAN_POINT ( 'NONE',  ( 2.655984681222220721E-16, 16.01562499938548356, 25.66244784525396483 ) ) ;
#67986=ORIENTED_EDGE ( 'NONE', *, *, #53130, .F. ) ;
#68005=EDGE_CURVE ( 'NONE', #49299, #70914, #58917, .T. ) ;
#68015=CARTESIAN_POINT ( 'NONE',  ( -1.878215178125001827, 18.00312499938548427, 33.25316411605952283 ) ) ;
#68054=ORIENTED_EDGE ( 'NONE', *, *, #12973, .F. ) ;
#68070=CARTESIAN_POINT ( 'NONE',  ( 0.6945827174705067053, 27.50000000000000000, 33.93923277410605976 ) ) ;
#68072=CARTESIAN_POINT ( 'NONE',  ( -1.878215178125001827, 16.54062499938548569, 33.25316411605952283 ) ) ;
#68093=ORIENTED_EDGE ( 'NONE', *, *, #62835, .F. ) ;
#68105=CARTESIAN_POINT ( 'NONE',  ( 3.999999999999998668, 17.80624999877096215, 32.30940107675850470 ) ) ;
#68118=VERTEX_POINT ( 'NONE', #24111 ) ;
#68155=ORIENTED_EDGE ( 'NONE', *, *, #60559, .T. ) ;
#68190=DIRECTION ( 'NONE',  ( 0.000000000000000000, 0.000000000000000000, 1.000000000000000000 ) ) ;
#68198=VERTEX_POINT ( 'NONE', #20384 ) ;
#68202=AXIS2_PLACEMENT_3D ( 'NONE', #29739, #18993, #19733 ) ;
#68227=CARTESIAN_POINT ( 'NONE',  ( -3.756430356250000102, 14.32812499938548356, 30.00000000000000000 ) ) ;
#68228=CARTESIAN_POINT ( 'NONE',  ( 0.000000000000000000, 27.50000000000000000, 26.00000000000000000 ) ) ;
#68253=EDGE_CURVE ( 'NONE', #69015, #38031, #55484, .T. ) ;
#68258=CARTESIAN_POINT ( 'NONE',  ( -3.999999999999999556, 20.33749999999999858, 27.69059892324149175 ) ) ;
#68270=CARTESIAN_POINT ( 'NONE',  ( 2.000000000000000444, 13.86874999877096748, 26.53589838486224650 ) ) ;
#68295=CARTESIAN_POINT ( 'NONE',  ( 1.071796769724491227, 14.39240381056766438, 26.00000000000000000 ) ) ;
#68338=CARTESIAN_POINT ( 'NONE',  ( 3.756430356249998770, 17.66562499938548214, 32.16877607737302469 ) ) ;
#68340=CARTESIAN_POINT ( 'NONE',  ( -3.756430356250001434, 20.10312499938548214, 32.16877607737301048 ) ) ;
#68377=CARTESIAN_POINT ( 'NONE',  ( 3.756430356250000102, 18.60312499938548214, 30.00000000000000000 ) ) ;
#68400=CARTESIAN_POINT ( 'NONE',  ( 4.000000000000000000, 13.38124999877096677, 27.69059892324149885 ) ) ;
#68429=CARTESIAN_POINT ( 'NONE',  ( -3.756430356250000990, 16.50312499938548427, 32.16877607737301048 ) ) ;
#68431=ORIENTED_EDGE ( 'NONE', *, *, #24642, .F. ) ;
#68459=CARTESIAN_POINT ( 'NONE',  ( -3.999999999999999556, 18.93124999877096570, 27.69059892324149175 ) ) ;
#68468=CARTESIAN_POINT ( 'NONE',  ( 4.000000000000000000, 12.89374999877096606, 30.00000000000000000 ) ) ;
#68469=DIRECTION ( 'NONE',  ( 0.000000000000000000, 0.000000000000000000, -1.000000000000000000 ) ) ;
#68486=CARTESIAN_POINT ( 'NONE',  ( -1.243387493232115393E-14, 14.86250000000000071, 26.00000000000000000 ) ) ;
#68519=CARTESIAN_POINT ( 'NONE',  ( 2.393811435568372112E-14, 19.08124999877097139, 34.00000000000000000 ) ) ;
#68524=CARTESIAN_POINT ( 'NONE',  ( -1.878215178124999163, 15.04062499938548392, 26.74683588394047007 ) ) ;
#68559=EDGE_CURVE ( 'NONE', #46076, #41970, #59362, .T. ) ;
#68578=CARTESIAN_POINT ( 'NONE',  ( 1.071796769724491227, 13.94240381056766509, 26.00000000000000000 ) ) ;
#68585=CARTESIAN_POINT ( 'NONE',  ( -7.967954043666661671E-16, 18.04062499938548214, 34.33755215474603517 ) ) ;
#68599=ORIENTED_EDGE ( 'NONE', *, *, #10213, .F. ) ;
#68617=CARTESIAN_POINT ( 'NONE',  ( 4.000000000000000000, 18.80000000000000071, 30.00000000000000000 ) ) ;
#68618=VECTOR ( 'NONE', #53453, 1000.000000000000000 ) ;
#68653=ORIENTED_EDGE ( 'NONE', *, *, #61021, .T. ) ;
#68662=B_SPLINE_CURVE_WITH_KNOTS ( 'NONE', 1,
 ( #8006, #33989 ),
 .UNSPECIFIED., .F., .F.,
 ( 2, 2 ),
 ( 0.000000000000000000, 1.000000000000000000 ),
 .UNSPECIFIED. ) ;
#68694=CYLINDRICAL_SURFACE ( 'NONE', #62654, 4.000000000000000000 ) ;
#68701=CARTESIAN_POINT ( 'NONE',  ( -3.756430356249999214, 17.89062499938548356, 27.83122392262697531 ) ) ;
#68703=CARTESIAN_POINT ( 'NONE',  ( -4.000000000000000000, 13.62500000000000000, 30.00000000000000000 ) ) ;
#68740=CARTESIAN_POINT ( 'NONE',  ( -7.967954043666661671E-16, 20.29062499938548214, 34.33755215474603517 ) ) ;
#68765=CARTESIAN_POINT ( 'NONE',  ( -2.672702088255949472E-15, 13.45624999877096784, 26.00000000000000000 ) ) ;
#68796=CARTESIAN_POINT ( 'NONE',  ( 1.878215178124997609, 17.51562499938548356, 33.25316411605952993 ) ) ;
#68798=ORIENTED_EDGE ( 'NONE', *, *, #24642, .T. ) ;
#68825=CARTESIAN_POINT ( 'NONE',  ( -1.878215178124999163, 12.90312499938548463, 26.74683588394047007 ) ) ;
#68857=CARTESIAN_POINT ( 'NONE',  ( 2.000000000000000444, 16.62500000000000000, 26.53589838486224650 ) ) ;
#68869=LINE ( 'NONE', #47418, #71432 ) ;
#68879=CARTESIAN_POINT ( 'NONE',  ( -4.000000000000000888, 19.00624999877096499, 32.30940107675850470 ) ) ;
#68884=CARTESIAN_POINT ( 'NONE',  ( -3.756430356249999214, 17.77812499938548285, 27.83122392262697531 ) ) ;
#68910=CARTESIAN_POINT ( 'NONE',  ( -3.999999999999999556, 13.53124999877096535, 27.69059892324149175 ) ) ;
#68946=CARTESIAN_POINT ( 'NONE',  ( -3.756430356249999214, 18.34062499938548640, 27.83122392262697176 ) ) ;
#68959=VERTEX_POINT ( 'NONE', #9253 ) ;
#68975=ORIENTED_EDGE ( 'NONE', *, *, #19271, .F. ) ;
#68981=CARTESIAN_POINT ( 'NONE',  ( -0.7391741542267653564, 20.47364048460824648, 34.19203975659616646 ) ) ;
#69015=VERTEX_POINT ( 'NONE', #58743 ) ;
#69018=CARTESIAN_POINT ( 'NONE',  ( 1.999999999999997335, 15.51874999877096784, 33.46410161513775705 ) ) ;
#69047=VECTOR ( 'NONE', #50872, 1000.000000000000000 ) ;
#69065=CARTESIAN_POINT ( 'NONE',  ( 3.756430356250000546, 19.09062499938548640, 27.83122392262697886 ) ) ;
#69067=CARTESIAN_POINT ( 'NONE',  ( -4.000000000000000888, 13.21250000000000036, 32.30940107675850470 ) ) ;
#69077=ORIENTED_EDGE ( 'NONE', *, *, #50916, .F. ) ;
#69104=CARTESIAN_POINT ( 'NONE',  ( -1.878215178125001827, 20.70312499938548001, 33.25316411605952283 ) ) ;
#69118=PRODUCT_DEFINITION_CONTEXT ( 'detailed design', #38961, 'design' ) ;
#69162=CARTESIAN_POINT ( 'NONE',  ( 1.878215178124997609, 17.96562499938548285, 33.25316411605952993 ) ) ;
#69173=CARTESIAN_POINT ( 'NONE',  ( 2.393811435568372112E-14, 19.08124999877097139, 34.00000000000000000 ) ) ;
#69190=CARTESIAN_POINT ( 'NONE',  ( -2.000000000000001776, 19.94374999877096499, 33.46410161513775705 ) ) ;
#69216=CARTESIAN_POINT ( 'NONE',  ( -2.672702088255949472E-15, 13.06250000000000355, 26.00000000000000000 ) ) ;
#69217=DIRECTION ( 'NONE',  ( -0.000000000000000000, -1.000000000000000000, -0.000000000000000000 ) ) ;
#69250=CARTESIAN_POINT ( 'NONE',  ( 3.756430356250000546, 18.52812499938548285, 27.83122392262697886 ) ) ;
#69275=CARTESIAN_POINT ( 'NONE',  ( 2.000000000000000444, 12.96874999877096712, 26.53589838486224650 ) ) ;
#69279=VERTEX_POINT ( 'NONE', #21415 ) ;
#69287=ADVANCED_FACE ( 'NONE', ( #49873 ), #22152, .T. ) ;
#69309=CARTESIAN_POINT ( 'NONE',  ( 2.655984681222220721E-16, 17.81562499938548427, 25.66244784525396483 ) ) ;
#69360=CARTESIAN_POINT ( 'NONE',  ( 1.071796769724489673, 13.88615380933863364, 26.00000000000000000 ) ) ;
#69383=ORIENTED_EDGE ( 'NONE', *, *, #25554, .F. ) ;
#69385=CARTESIAN_POINT ( 'NONE',  ( 4.000000000000000000, 14.30000000000000071, 30.00000000000000000 ) ) ;
#69397=CARTESIAN_POINT ( 'NONE',  ( 5.810221930991193690E-16, 18.01249999999999218, 26.00000000000000000 ) ) ;
#69401=CARTESIAN_POINT ( 'NONE',  ( 2.393811435568372112E-14, 18.68750000000000355, 34.00000000000000000 ) ) ;
#69406=DIRECTION ( 'NONE',  ( 0.000000000000000000, 0.000000000000000000, -1.000000000000000000 ) ) ;
#69411=CARTESIAN_POINT ( 'NONE',  ( 1.071796769724490561, 13.30759618943233491, 34.00000000000000000 ) ) ;
#69420=DIRECTION ( 'NONE',  ( -0.000000000000000000, -1.000000000000000000, -0.000000000000000000 ) ) ;
#69426=CARTESIAN_POINT ( 'NONE',  ( 3.756430356249998770, 19.46562499938548285, 32.16877607737302469 ) ) ;
#69428=CARTESIAN_POINT ( 'NONE',  ( -1.878215178125001827, 20.59062499938548285, 33.25316411605952283 ) ) ;
#69465=CARTESIAN_POINT ( 'NONE',  ( -3.756430356250001434, 19.31562499938548427, 32.16877607737301048 ) ) ;
#69480=EDGE_CURVE ( 'NONE', #12248, #57768, #28319, .T. ) ;
#69520=CARTESIAN_POINT ( 'NONE',  ( -3.756430356250000102, 16.91562499938548214, 30.00000000000000000 ) ) ;
#69549=CARTESIAN_POINT ( 'NONE',  ( -3.999999999999999556, 19.83124999877096073, 27.69059892324149175 ) ) ;
#69571=DIRECTION ( 'NONE',  ( -0.000000000000000000, -1.000000000000000000, -0.000000000000000000 ) ) ;
#69579=CARTESIAN_POINT ( 'NONE',  ( 4.000000000000000000, 16.58750000000000213, 27.69059892324149885 ) ) ;
#69594=EDGE_LOOP ( 'NONE', ( #19553, #28354, #62228, #11356 ) ) ;
#69609=CARTESIAN_POINT ( 'NONE',  ( -1.878215178125001827, 17.44062499938548072, 33.25316411605952283 ) ) ;
#69631=CARTESIAN_POINT ( 'NONE',  ( 2.000000000000000444, 13.41874999877096641, 26.53589838486224650 ) ) ;
#69663=CARTESIAN_POINT ( 'NONE',  ( -3.756430356250000102, 17.92812499938548498, 30.00000000000000000 ) ) ;
#69699=CARTESIAN_POINT ( 'NONE',  ( -2.000000000000001776, 19.09999999999999787, 33.46410161513775705 ) ) ;
#69714=VERTEX_POINT ( 'NONE', #37138 ) ;
#69757=ADVANCED_FACE ( 'NONE', ( #38236 ), #31235, .T. ) ;
#69779=CARTESIAN_POINT ( 'NONE',  ( -1.878215178124999163, 18.75312499938548427, 26.74683588394047007 ) ) ;
#69781=CARTESIAN_POINT ( 'NONE',  ( -8.484601909799255319E-16, 12.83750000000000036, 34.61880215351700940 ) ) ;
#69820=CARTESIAN_POINT ( 'NONE',  ( 1.878215178125000495, 20.47812499938548569, 26.74683588394047007 ) ) ;
#69857=CARTESIAN_POINT ( 'NONE',  ( -3.591883811668507676, 25.10396054455708637, 31.77987931115919906 ) ) ;
#69872=VECTOR ( 'NONE', #3932, 1000.000000000000000 ) ;
#69874=CARTESIAN_POINT ( 'NONE',  ( -3.756430356250000102, 18.71562499938548285, 30.00000000000000000 ) ) ;
#69904=CARTESIAN_POINT ( 'NONE',  ( 4.000000000000000000, 20.13124999877096499, 27.69059892324149530 ) ) ;
#69915=ORIENTED_EDGE ( 'NONE', *, *, #37745, .F. ) ;
#69940=ORIENTED_EDGE ( 'NONE', *, *, #17942, .F. ) ;
#69964=CARTESIAN_POINT ( 'NONE',  ( -1.878215178124999163, 17.29062499938548214, 26.74683588394047007 ) ) ;
#69975=CARTESIAN_POINT ( 'NONE',  ( -3.756430356250001434, 15.15312499938548463, 32.16877607737301048 ) ) ;
#69989=CARTESIAN_POINT ( 'NONE',  ( -3.999999999999999556, 13.98124999877096641, 27.69059892324149175 ) ) ;
#70021=CARTESIAN_POINT ( 'NONE',  ( -3.756430356250000102, 17.47812499938548214, 30.00000000000000000 ) ) ;
#70050=ORIENTED_EDGE ( 'NONE', *, *, #56762, .T. ) ;
#70056=CARTESIAN_POINT ( 'NONE',  ( -2.498395430326213790E-14, 18.46250000000000213, 26.00000000000000000 ) ) ;
#70120=CARTESIAN_POINT ( 'NONE',  ( 3.793609269539072404, 25.05402749099526005, 28.70526358585616578 ) ) ;
#70129=AXIS2_PLACEMENT_3D ( 'NONE', #41142, #69217, #1983 ) ;
#70134=CARTESIAN_POINT ( 'NONE',  ( -1.626862140677534273E-15, 17.33749999999999858, 34.00000000000000000 ) ) ;
#70137=CARTESIAN_POINT ( 'NONE',  ( -3.756430356250000102, 20.17812499938548143, 30.00000000000000000 ) ) ;
#70139=CARTESIAN_POINT ( 'NONE',  ( 2.828200636599751609E-16, 15.31250000000000000, 25.38119784648299415 ) ) ;
#70149=AXIS2_PLACEMENT_3D ( 'NONE', #10360, #72783, #22166 ) ;
#70202=AXIS2_PLACEMENT_3D ( 'NONE', #62382, #46488, #51668 ) ;
#70219=CARTESIAN_POINT ( 'NONE',  ( -1.042164773807799261, 25.50793453900451979, 26.12922642428445741 ) ) ;
#70222=CARTESIAN_POINT ( 'NONE',  ( -3.756430356250000102, 14.77812499938548463, 30.00000000000000000 ) ) ;
#70236=CARTESIAN_POINT ( 'NONE',  ( 3.756430356250000546, 18.97812499938548214, 27.83122392262697886 ) ) ;
#70270=CARTESIAN_POINT ( 'NONE',  ( -2.000000000000001776, 20.39374999877096428, 33.46410161513775705 ) ) ;
#70279=CARTESIAN_POINT ( 'NONE',  ( 1.071796769724500997, 18.70759618943233349, 33.99999999999999289 ) ) ;
#70282=ORIENTED_EDGE ( 'NONE', *, *, #71109, .T. ) ;
#70290=EDGE_CURVE ( 'NONE', #17018, #38031, #10935, .T. ) ;
#70297=CARTESIAN_POINT ( 'NONE',  ( -1.243387493232115393E-14, 15.31250000000000000, 26.00000000000000000 ) ) ;
#70323=CARTESIAN_POINT ( 'NONE',  ( -7.967954043666661671E-16, 12.97812499938548392, 34.33755215474603517 ) ) ;
#70330=CARTESIAN_POINT ( 'NONE',  ( 3.756430356250000546, 18.07812499938548711, 27.83122392262697886 ) ) ;
#70339=CARTESIAN_POINT ( 'NONE',  ( 3.756430356250000546, 15.37812499938548427, 27.83122392262697886 ) ) ;
#70356=CARTESIAN_POINT ( 'NONE',  ( -1.999999999999999112, 13.49374999877096570, 26.53589838486224650 ) ) ;
#70390=CARTESIAN_POINT ( 'NONE',  ( -3.756430356249999214, 19.24062499938548143, 27.83122392262697176 ) ) ;
#70417=CARTESIAN_POINT ( 'NONE',  ( 1.071796769724491227, 14.33615380933862937, 26.00000000000000000 ) ) ;
#70421=ORIENTED_EDGE ( 'NONE', *, *, #12871, .F. ) ;
#70458=( BOUNDED_CURVE ( )  B_SPLINE_CURVE ( 2, ( #66826, #16558, #39109, #16916, #27298, #33550, #38750, #56100, #45376 ),
 .UNSPECIFIED., .F., .F. ) 
 B_SPLINE_CURVE_WITH_KNOTS ( ( 3, 2, 2, 2, 3 ),
 ( 0.8750000000000000000, 0.8796296296296296502, 0.8888888888888888395, 0.8981481481481481399, 0.9027777777777777901 ),
 .UNSPECIFIED. ) 
 CURVE ( )  GEOMETRIC_REPRESENTATION_ITEM ( )  RATIONAL_B_SPLINE_CURVE ( ( 0.9330127018922194093, 0.9330127018922194093, 1.000000000000000000, 0.8660254037844387076, 1.000000000000000000, 0.8660254037844387076, 1.000000000000000000, 0.9330127018922194093, 0.9330127018922194093 ) ) 
 REPRESENTATION_ITEM ( '' )  );
#70501=CARTESIAN_POINT ( 'NONE',  ( 0.000000000000000000, 27.50000000000000000, 30.00000000000000000 ) ) ;
#70510=CARTESIAN_POINT ( 'NONE',  ( 3.756430356249998770, 13.05312499938548321, 32.16877607737302469 ) ) ;
#70512=CARTESIAN_POINT ( 'NONE',  ( 3.999999999999998668, 16.06250000000000000, 32.30940107675850470 ) ) ;
#70517=CARTESIAN_POINT ( 'NONE',  ( 2.393811435568372112E-14, 18.23750000000000071, 34.00000000000000000 ) ) ;
#70548=ORIENTED_EDGE ( 'NONE', *, *, #16156, .F. ) ;
#70590=CARTESIAN_POINT ( 'NONE',  ( 3.756430356249998770, 14.06562499938548250, 32.16877607737302469 ) ) ;
#70603=CARTESIAN_POINT ( 'NONE',  ( -1.878215178124999163, 19.54062499938548214, 26.74683588394047007 ) ) ;
#70605=ORIENTED_EDGE ( 'NONE', *, *, #4912, .F. ) ;
#70620=VERTEX_POINT ( 'NONE', #23422 ) ;
#70627=EDGE_LOOP ( 'NONE', ( #23927, #53243, #35283, #43439 ) ) ;
#70631=CARTESIAN_POINT ( 'NONE',  ( -3.756430356250001434, 16.16562499938548569, 32.16877607737301048 ) ) ;
#70639=CARTESIAN_POINT ( 'NONE',  ( 3.999999999999998668, 18.76250000000000284, 32.30940107675850470 ) ) ;
#70656=CARTESIAN_POINT ( 'NONE',  ( -1.243387493232115393E-14, 16.15624999877096712, 26.00000000000000000 ) ) ;
#70685=CARTESIAN_POINT ( 'NONE',  ( -1.999999999999999112, 14.00000000000000000, 26.53589838486224650 ) ) ;
#70692=CARTESIAN_POINT ( 'NONE',  ( -1.878215178125001827, 20.59062499938548285, 33.25316411605952283 ) ) ;
#70701=CARTESIAN_POINT ( 'NONE',  ( 3.756430356250000102, 16.24062499938548143, 30.00000000000000000 ) ) ;
#70716=CARTESIAN_POINT ( 'NONE',  ( 1.999999999999997335, 15.06874999877096677, 33.46410161513775705 ) ) ;
#70742=VECTOR ( 'NONE', #21418, 1000.000000000000000 ) ;
#70748=CARTESIAN_POINT ( 'NONE',  ( -3.999999999999999112, 12.68750000000000000, 27.69059892324149530 ) ) ;
#70751=CARTESIAN_POINT ( 'NONE',  ( 1.878215178125000495, 19.57812499938548356, 26.74683588394047007 ) ) ;
#70824=VERTEX_POINT ( 'NONE', #66342 ) ;
#70842=EDGE_CURVE ( 'NONE', #31816, #51293, #20160, .T. ) ;
#70847=CARTESIAN_POINT ( 'NONE',  ( 3.999999999999998668, 16.96249999999999858, 32.30940107675850470 ) ) ;
#70874=CARTESIAN_POINT ( 'NONE',  ( 1.878215178124997609, 19.87812499938548072, 33.25316411605952993 ) ) ;
#70876=CARTESIAN_POINT ( 'NONE',  ( 1.999999999999997335, 16.02500000000000213, 33.46410161513775705 ) ) ;
#70897=EDGE_CURVE ( 'NONE', #53615, #13783, #42714, .T. ) ;
#70914=VERTEX_POINT ( 'NONE', #8725 ) ;
#70915=ORIENTED_EDGE ( 'NONE', *, *, #21036, .T. ) ;
#70932=LINE ( 'NONE', #14768, #36172 ) ;
#70959=CARTESIAN_POINT ( 'NONE',  ( 3.756430356250000546, 14.59062499938548463, 27.83122392262697886 ) ) ;
#70970=CARTESIAN_POINT ( 'NONE',  ( -3.756430356250000102, 19.16562499938548214, 30.00000000000000000 ) ) ;
#70981=CARTESIAN_POINT ( 'NONE',  ( 1.071796769724491893, 14.60134618820329777, 34.00000000000000000 ) ) ;
#71000=CARTESIAN_POINT ( 'NONE',  ( 2.655984681222220721E-16, 15.56562499938548250, 25.66244784525396483 ) ) ;
#71072=CARTESIAN_POINT ( 'NONE',  ( 3.756430356250000546, 16.72812499938548214, 27.83122392262697886 ) ) ;
#71086=CARTESIAN_POINT ( 'NONE',  ( -4.000000000000000888, 17.20624999877096428, 32.30940107675850470 ) ) ;
#71099=VECTOR ( 'NONE', #29987, 1000.000000000000000 ) ;
#71109=EDGE_CURVE ( 'NONE', #27542, #40431, #35841, .T. ) ;
#71119=CARTESIAN_POINT ( 'NONE',  ( 2.655984681222220721E-16, 20.51562499938548356, 25.66244784525396483 ) ) ;
#71128=CARTESIAN_POINT ( 'NONE',  ( -1.071796769724502107, 20.28259618943232923, 26.00000000000000711 ) ) ;
#71132=VERTEX_POINT ( 'NONE', #10193 ) ;
#71153=CARTESIAN_POINT ( 'NONE',  ( 1.071796769724479237, 18.44240381056765798, 25.99999999999999645 ) ) ;
#71154=CARTESIAN_POINT ( 'NONE',  ( -1.071796769724492115, 18.16115380933862866, 34.00000000000000000 ) ) ;
#71157=CARTESIAN_POINT ( 'NONE',  ( 0.000000000000000000, 27.50000000000000000, 26.00000000000000000 ) ) ;
#71209=CARTESIAN_POINT ( 'NONE',  ( -3.756430356250000102, 13.42812499938548321, 30.00000000000000000 ) ) ;
#71220=VERTEX_POINT ( 'NONE', #33445 ) ;
#71236=CARTESIAN_POINT ( 'NONE',  ( 2.655984681222220721E-16, 13.20312499938548534, 25.66244784525396483 ) ) ;
#71238=CARTESIAN_POINT ( 'NONE',  ( 2.828200636599751609E-16, 14.86250000000000071, 25.38119784648299415 ) ) ;
#71287=ORIENTED_EDGE ( 'NONE', *, *, #16220, .F. ) ;
#71305=EDGE_CURVE ( 'NONE', #5101, #57768, #849, .T. ) ;
#71326=CARTESIAN_POINT ( 'NONE',  ( 3.756430356250000546, 13.24062499938548321, 27.83122392262697886 ) ) ;
#71337=CARTESIAN_POINT ( 'NONE',  ( 3.756430356249998770, 20.25312499938547717, 32.16877607737301759 ) ) ;
#71370=CARTESIAN_POINT ( 'NONE',  ( 1.878215178125000495, 15.52812499938548285, 26.74683588394047007 ) ) ;
#71393=B_SPLINE_CURVE_WITH_KNOTS ( 'NONE', 1,
 ( #9044, #58170 ),
 .UNSPECIFIED., .F., .F.,
 ( 2, 2 ),
 ( 0.000000000000000000, 1.000000000000000000 ),
 .UNSPECIFIED. ) ;
#71425=CARTESIAN_POINT ( 'NONE',  ( -1.878215178124999163, 12.79062499938548392, 26.74683588394047007 ) ) ;
#71432=VECTOR ( 'NONE', #8258, 1000.000000000000000 ) ;
#71443=CARTESIAN_POINT ( 'NONE',  ( -3.756430356250000102, 16.46562499938548285, 30.00000000000000000 ) ) ;
#71459=CARTESIAN_POINT ( 'NONE',  ( -2.000000000000001776, 15.44374999877096677, 33.46410161513775705 ) ) ;
#71485=CARTESIAN_POINT ( 'NONE',  ( -1.071796769724480347, 18.66740381056766651, 34.00000000000000711 ) ) ;
#71492=CARTESIAN_POINT ( 'NONE',  ( -3.756430356249999214, 20.59062499938548640, 27.83122392262697176 ) ) ;
#71575=CARTESIAN_POINT ( 'NONE',  ( 1.878215178125000495, 13.61562499938548321, 26.74683588394047007 ) ) ;
#71602=DIRECTION ( 'NONE',  ( 0.000000000000000000, 1.000000000000000000, 0.000000000000000000 ) ) ;
#71613=CARTESIAN_POINT ( 'NONE',  ( 3.756430356250000546, 12.67812499938548143, 27.83122392262697886 ) ) ;
#71615=CARTESIAN_POINT ( 'NONE',  ( 4.000000000000000000, 16.10000000000000142, 30.00000000000000000 ) ) ;
#71648=CARTESIAN_POINT ( 'NONE',  ( -1.071796769724492115, 17.76740381056766438, 34.00000000000000000 ) ) ;
#71692=CARTESIAN_POINT ( 'NONE',  ( -1.071796769724486120, 15.96740381056766722, 34.00000000000000000 ) ) ;
#71701=CARTESIAN_POINT ( 'NONE',  ( 4.000000000000000000, 15.68750000000000000, 27.69059892324149885 ) ) ;
#71711=CARTESIAN_POINT ( 'NONE',  ( 0.000000000000000000, 27.50000000000000000, 30.00000000000000000 ) ) ;
#71713=ORIENTED_EDGE ( 'NONE', *, *, #68005, .F. ) ;
#71722=CARTESIAN_POINT ( 'NONE',  ( 4.000000000000000000, 14.69374999877096677, 30.00000000000000000 ) ) ;
#71744=CARTESIAN_POINT ( 'NONE',  ( 3.756430356249998770, 15.41562499938548392, 32.16877607737302469 ) ) ;
#71753=DIRECTION ( 'NONE',  ( -1.000000000000000000, -0.000000000000000000, -0.000000000000000000 ) ) ;
#71798=CARTESIAN_POINT ( 'NONE',  ( 3.756430356249998770, 13.95312499938548534, 32.16877607737301759 ) ) ;
#71804=CARTESIAN_POINT ( 'NONE',  ( 3.756430356250000102, 19.39062499938548356, 30.00000000000000000 ) ) ;
#71813=CARTESIAN_POINT ( 'NONE',  ( -1.878215178125001827, 17.89062499938548356, 33.25316411605952283 ) ) ;
#71828=CARTESIAN_POINT ( 'NONE',  ( 2.828200636599751609E-16, 16.60624999877096641, 25.38119784648299415 ) ) ;
#71856=EDGE_CURVE ( 'NONE', #8994, #27542, #25496, .T. ) ;
#71860=CARTESIAN_POINT ( 'NONE',  ( -7.967954043666661671E-16, 19.39062499938548356, 34.33755215474603517 ) ) ;
#71861=CARTESIAN_POINT ( 'NONE',  ( 0.000000000000000000, 27.50000000000000000, 30.00000000000000000 ) ) ;
#71878=CARTESIAN_POINT ( 'NONE',  ( 4.000000000000000000, 19.25000000000000000, 30.00000000000000000 ) ) ;
#71931=CARTESIAN_POINT ( 'NONE',  ( -1.626862140677534273E-15, 16.83124999877096428, 34.00000000000000000 ) ) ;
#71940=CARTESIAN_POINT ( 'NONE',  ( 3.756430356250000102, 13.54062499938548392, 30.00000000000000000 ) ) ;
#71948=CARTESIAN_POINT ( 'NONE',  ( 2.655984681222220721E-16, 12.86562499938548321, 25.66244784525396483 ) ) ;
#71968=DIRECTION ( 'NONE',  ( -0.000000000000000000, -1.000000000000000000, -0.000000000000000000 ) ) ;
#71973=VERTEX_POINT ( 'NONE', #66534 ) ;
#71977=CARTESIAN_POINT ( 'NONE',  ( 2.655984681222220721E-16, 14.55312499938548321, 25.66244784525396483 ) ) ;
#71979=CARTESIAN_POINT ( 'NONE',  ( -8.484601909799255319E-16, 17.78750000000000142, 34.61880215351700940 ) ) ;
#72011=ORIENTED_EDGE ( 'NONE', *, *, #59196, .T. ) ;
#72023=CARTESIAN_POINT ( 'NONE',  ( -1.071796769724490561, 13.02634618820330381, 26.00000000000000000 ) ) ;
#72055=CARTESIAN_POINT ( 'NONE',  ( -3.756430356249999214, 15.64062499938548179, 27.83122392262697531 ) ) ;
#72063=CARTESIAN_POINT ( 'NONE',  ( 2.000000000000000444, 16.56874999877096499, 26.53589838486224650 ) ) ;
#72093=ORIENTED_EDGE ( 'NONE', *, *, #65868, .F. ) ;
#72096=CARTESIAN_POINT ( 'NONE',  ( -3.756430356250000102, 15.67812499938548143, 30.00000000000000000 ) ) ;
#72139=DIRECTION ( 'NONE',  ( -0.000000000000000000, -1.000000000000000000, -0.000000000000000000 ) ) ;
#72142=CARTESIAN_POINT ( 'NONE',  ( 0.000000000000000000, 27.50000000000000000, 30.00000000000000000 ) ) ;
#72155=CARTESIAN_POINT ( 'NONE',  ( 2.655984681222220721E-16, 13.65312499938548285, 25.66244784525396483 ) ) ;
#72161=CARTESIAN_POINT ( 'NONE',  ( -3.756430356250000102, 20.06562499938548072, 30.00000000000000000 ) ) ;
#72171=CARTESIAN_POINT ( 'NONE',  ( 2.655984681222220721E-16, 18.15312499938548285, 25.66244784525396483 ) ) ;
#72181=CARTESIAN_POINT ( 'NONE',  ( 3.999999999999998668, 15.16250000000000142, 32.30940107675850470 ) ) ;
#72188=CARTESIAN_POINT ( 'NONE',  ( 3.999999999999998668, 16.90624999877096712, 32.30940107675850470 ) ) ;
#72300=CARTESIAN_POINT ( 'NONE',  ( -3.756430356250001434, 13.80312499938548321, 32.16877607737301048 ) ) ;
#72308=CARTESIAN_POINT ( 'NONE',  ( -1.878215178124999163, 15.60312499938548392, 26.74683588394047007 ) ) ;
#72336=CARTESIAN_POINT ( 'NONE',  ( 1.878215178124997609, 14.36562499938548321, 33.25316411605952993 ) ) ;
#72338=CARTESIAN_POINT ( 'NONE',  ( 2.828200636599751609E-16, 16.66249999999999787, 25.38119784648299415 ) ) ;
#72398=DIRECTION ( 'NONE',  ( -0.000000000000000000, -1.000000000000000000, -0.000000000000000000 ) ) ;
#72417=CARTESIAN_POINT ( 'NONE',  ( -3.756430356250000102, 17.02812499938548285, 30.00000000000000000 ) ) ;
#72428=DIRECTION ( 'NONE',  ( 0.000000000000000000, 0.000000000000000000, -1.000000000000000000 ) ) ;
#72457=VERTEX_POINT ( 'NONE', #2127 ) ;
#72460=CARTESIAN_POINT ( 'NONE',  ( -7.967954043666661671E-16, 18.04062499938548214, 34.33755215474603517 ) ) ;
#72495=EDGE_CURVE ( 'NONE', #41056, #49222, #31282, .T. ) ;
#72503=FACE_OUTER_BOUND ( 'NONE', #32298, .T. ) ;
#72516=CARTESIAN_POINT ( 'NONE',  ( -7.967954043666661671E-16, 14.32812499938548356, 34.33755215474603517 ) ) ;
#72533=CARTESIAN_POINT ( 'NONE',  ( -3.756430356249999214, 18.67812499938548143, 27.83122392262697531 ) ) ;
#72549=CARTESIAN_POINT ( 'NONE',  ( -2.000000000000001776, 18.14374999877096428, 33.46410161513775705 ) ) ;
#72581=AXIS2_PLACEMENT_3D ( 'NONE', #15153, #15515, #54692 ) ;
#72584=CARTESIAN_POINT ( 'NONE',  ( -1.071796769724479903, 20.86115380933863150, 34.00000000000000711 ) ) ;
#72602=EDGE_CURVE ( 'NONE', #24717, #69279, #42008, .T. ) ;
#72649=EDGE_CURVE ( 'NONE', #12632, #49222, #8030, .T. ) ;
#72669=CARTESIAN_POINT ( 'NONE',  ( -1.878215178125001827, 13.39062499938548356, 33.25316411605952283 ) ) ;
#72676=CARTESIAN_POINT ( 'NONE',  ( 3.756430356249998770, 14.06562499938548250, 32.16877607737301759 ) ) ;
#72677=CARTESIAN_POINT ( 'NONE',  ( -3.999999999999999112, 15.33124999877096606, 27.69059892324149530 ) ) ;
#72678=AXIS2_PLACEMENT_3D ( 'NONE', #33026, #21570, #61461 ) ;
#72700=ORIENTED_EDGE ( 'NONE', *, *, #68253, .F. ) ;
#72703=CARTESIAN_POINT ( 'NONE',  ( -1.878215178124999163, 14.59062499938548463, 26.74683588394047007 ) ) ;
#72706=CARTESIAN_POINT ( 'NONE',  ( -4.000000000000000000, 18.12500000000000355, 30.00000000000000000 ) ) ;
#72735=VECTOR ( 'NONE', #60658, 1000.000000000000000 ) ;
#72783=DIRECTION ( 'NONE',  ( 1.000000000000000000, 0.000000000000000000, 0.000000000000000000 ) ) ;
#72788=CARTESIAN_POINT ( 'NONE',  ( -3.756430356250001434, 16.16562499938548569, 32.16877607737301048 ) ) ;
#72831=CARTESIAN_POINT ( 'NONE',  ( 1.878215178124997609, 17.17812499938548498, 33.25316411605952993 ) ) ;
#72844=EDGE_LOOP ( 'NONE', ( #4435, #64040, #22693, #37239 ) ) ;
#72888=CARTESIAN_POINT ( 'NONE',  ( 1.878215178125000495, 15.41562499938548392, 26.74683588394047007 ) ) ;
#72902=CARTESIAN_POINT ( 'NONE',  ( 2.655984681222220721E-16, 19.50312499938548427, 25.66244784525396483 ) ) ;
#72916=CARTESIAN_POINT ( 'NONE',  ( 3.999999999999998668, 17.35624999877096641, 32.30940107675850470 ) ) ;
#72919=CARTESIAN_POINT ( 'NONE',  ( -2.000000000000001776, 17.69374999877096855, 33.46410161513775705 ) ) ;
#72942=EDGE_CURVE ( 'NONE', #70914, #53615, #42973, .T. ) ;
#72950=FACE_OUTER_BOUND ( 'NONE', #43189, .T. ) ;
#73035=CARTESIAN_POINT ( 'NONE',  ( 3.756430356250000102, 15.45312499938548356, 30.00000000000000000 ) ) ;
#73036=CARTESIAN_POINT ( 'NONE',  ( 1.138803498474273873E-14, 15.48124999877096641, 34.00000000000000000 ) ) ;
#73067=CARTESIAN_POINT ( 'NONE',  ( -4.000000000000000000, 17.67500000000000071, 30.00000000000000000 ) ) ;
#73138=COLOUR_RGB('Sky Blue',0.24,0.69,0.87);
#73139=FILL_AREA_STYLE_COLOUR('',#73138);
#73140=FILL_AREA_STYLE('',(#73139));
#73141=SURFACE_STYLE_FILL_AREA(#73140);
#73142=SURFACE_SIDE_STYLE('',(#73141));
#73143=SURFACE_STYLE_USAGE(.BOTH.,#73142);
#73144=PRESENTATION_STYLE_ASSIGNMENT((#73143));
ENDSEC;
END-ISO-10303-21;
